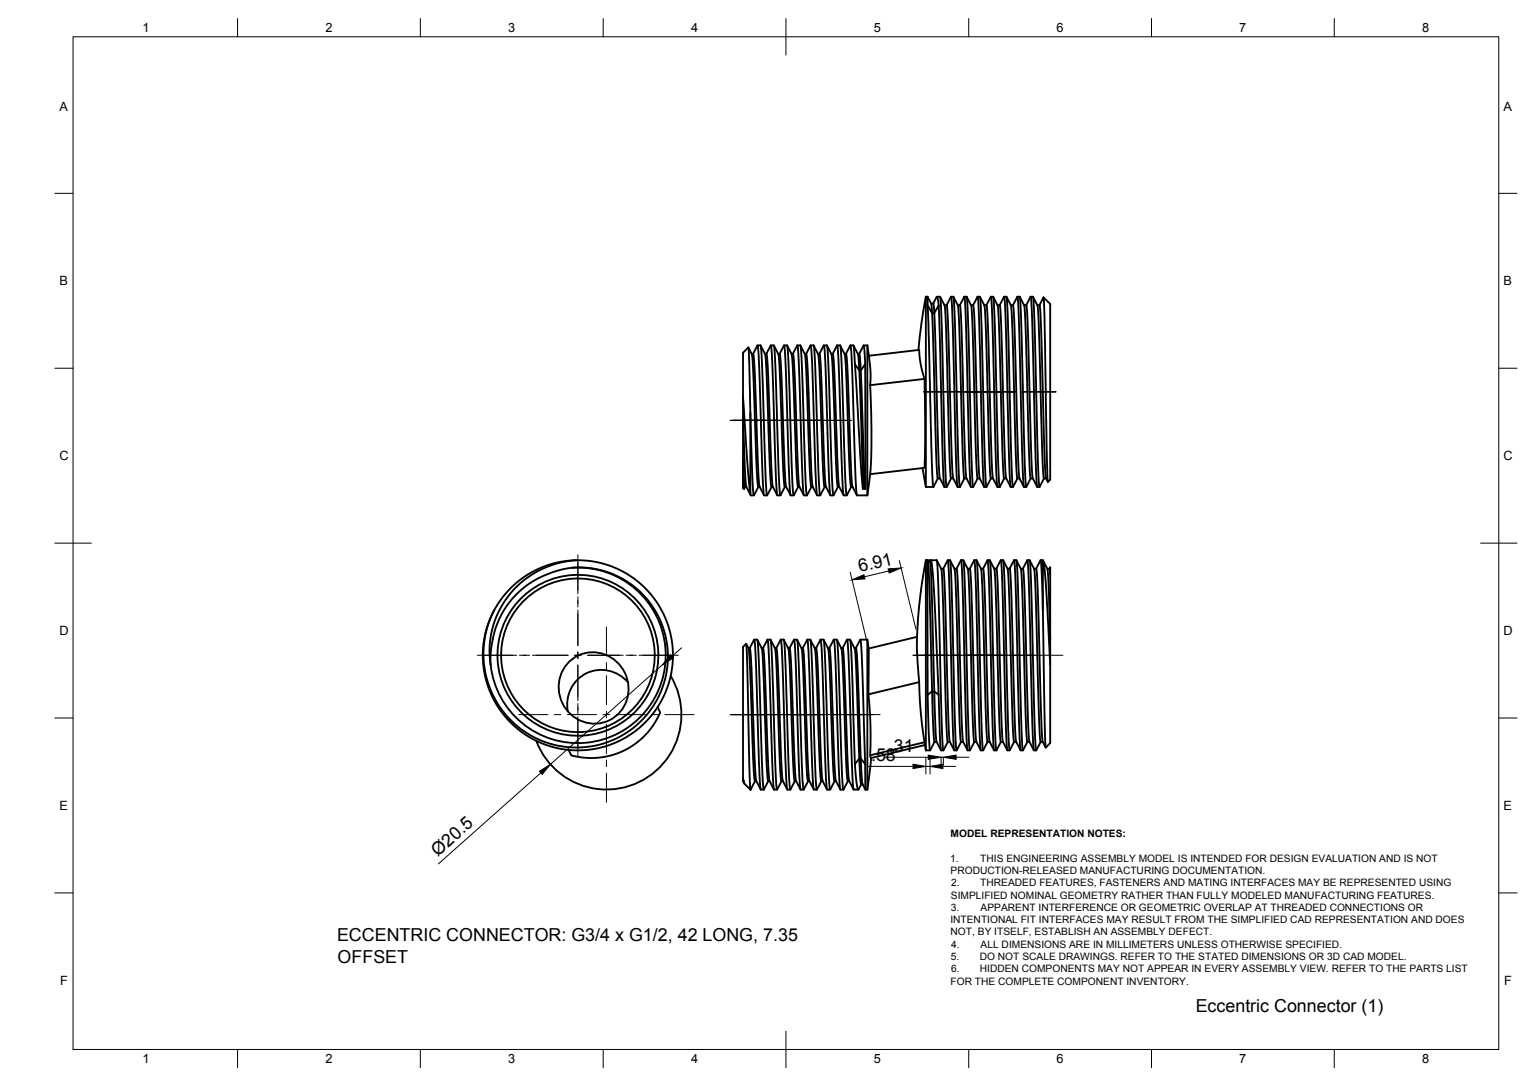
ISO-10303-21;
HEADER;
/* Generated by software containing ST-Developer
 * from STEP Tools, Inc. (www.steptools.com) 
 */

FILE_DESCRIPTION(
/* description */ ('STEP AP214'),
/* implementation_level */ '2;1');

FILE_NAME(
/* name */ 'Eccentric Connector (1).step',
/* time_stamp */ '2026-10-05T23:18:41-07:00',
/* author */ (''),
/* organization */ (''),
/* preprocessor_version */ 'ST-DEVELOPER v20.2',
/* originating_system */ 'Autodesk Translation Framework v15.15.0.0',
/* authorisation */ '');

FILE_SCHEMA (('AUTOMOTIVE_DESIGN { 1 0 10303 214 3 1 1 }'));
ENDSEC;

DATA;
#10=MECHANICAL_DESIGN_GEOMETRIC_PRESENTATION_REPRESENTATION('',(#111),#221662);
#72=MANIFOLD_SOLID_BREP('Body1',#79334);
#85=SHAPE_REPRESENTATION_RELATIONSHIP('SRR','None',#221720,#98);
#98=ADVANCED_BREP_SHAPE_REPRESENTATION('',(#72),#221660);
#111=STYLED_ITEM('',(#221783),#72);
#207=B_SPLINE_SURFACE_WITH_KNOTS('',3,3,((#208963,#208964,#208965,#208966,
#208967,#208968,#208969),(#208970,#208971,#208972,#208973,#208974,#208975,
#208976),(#208977,#208978,#208979,#208980,#208981,#208982,#208983),(#208984,
#208985,#208986,#208987,#208988,#208989,#208990)),.UNSPECIFIED.,.F.,.F.,
 .F.,(4,4),(4,1,1,1,4),(0.,1.),(0.,0.25,0.5,0.75,1.),.UNSPECIFIED.);
#208=B_SPLINE_SURFACE_WITH_KNOTS('',3,3,((#209027,#209028,#209029,#209030,
#209031,#209032,#209033,#209034,#209035,#209036,#209037,#209038,#209039,
#209040,#209041,#209042,#209043,#209044,#209045,#209046,#209047,#209048,
#209049,#209050,#209051,#209052,#209053,#209054,#209055,#209056,#209057,
#209058,#209059,#209060,#209061,#209062,#209063,#209064,#209065,#209066,
#209067,#209068,#209069,#209070,#209071,#209072,#209073,#209074,#209075,
#209076,#209077,#209078,#209079,#209080,#209081,#209082,#209083,#209084,
#209085,#209086,#209087,#209088,#209089,#209090,#209091,#209092,#209093),
(#209094,#209095,#209096,#209097,#209098,#209099,#209100,#209101,#209102,
#209103,#209104,#209105,#209106,#209107,#209108,#209109,#209110,#209111,
#209112,#209113,#209114,#209115,#209116,#209117,#209118,#209119,#209120,
#209121,#209122,#209123,#209124,#209125,#209126,#209127,#209128,#209129,
#209130,#209131,#209132,#209133,#209134,#209135,#209136,#209137,#209138,
#209139,#209140,#209141,#209142,#209143,#209144,#209145,#209146,#209147,
#209148,#209149,#209150,#209151,#209152,#209153,#209154,#209155,#209156,
#209157,#209158,#209159,#209160),(#209161,#209162,#209163,#209164,#209165,
#209166,#209167,#209168,#209169,#209170,#209171,#209172,#209173,#209174,
#209175,#209176,#209177,#209178,#209179,#209180,#209181,#209182,#209183,
#209184,#209185,#209186,#209187,#209188,#209189,#209190,#209191,#209192,
#209193,#209194,#209195,#209196,#209197,#209198,#209199,#209200,#209201,
#209202,#209203,#209204,#209205,#209206,#209207,#209208,#209209,#209210,
#209211,#209212,#209213,#209214,#209215,#209216,#209217,#209218,#209219,
#209220,#209221,#209222,#209223,#209224,#209225,#209226,#209227),(#209228,
#209229,#209230,#209231,#209232,#209233,#209234,#209235,#209236,#209237,
#209238,#209239,#209240,#209241,#209242,#209243,#209244,#209245,#209246,
#209247,#209248,#209249,#209250,#209251,#209252,#209253,#209254,#209255,
#209256,#209257,#209258,#209259,#209260,#209261,#209262,#209263,#209264,
#209265,#209266,#209267,#209268,#209269,#209270,#209271,#209272,#209273,
#209274,#209275,#209276,#209277,#209278,#209279,#209280,#209281,#209282,
#209283,#209284,#209285,#209286,#209287,#209288,#209289,#209290,#209291,
#209292,#209293,#209294)),.UNSPECIFIED.,.F.,.F.,.F.,(4,4),(4,1,1,1,1,1,
1,1,1,1,1,1,1,1,1,1,1,1,1,1,1,1,1,1,1,1,1,1,1,1,1,1,1,1,1,1,1,1,1,1,1,1,
1,1,1,1,1,1,1,1,1,1,1,1,1,1,1,1,1,1,1,1,1,1,4),(0.,1.),(0.,0.0156250000000022,
0.0312500000000006,0.0468750000000009,0.0625000000000012,0.0781250000000015,
0.0937500000000018,0.109375000000002,0.124999999999983,0.140624999999983,
0.156249999999984,0.171874999999984,0.187499999999984,0.203124999999984,
0.218749999999985,0.234374999999986,0.249999999999986,0.265624999999986,
0.281249999999986,0.296874999999986,0.312499999999987,0.328124999999987,
0.343749999999987,0.359374999999987,0.374999999999988,0.390624999999988,
0.406249999999988,0.421874999999989,0.437499999999989,0.45312499999999,
0.46874999999999,0.48437499999999,0.49999999999999,0.515624999999991,0.531249999999991,
0.546874999999991,0.562499999999992,0.578124999999992,0.593749999999992,
0.609374999999993,0.624999999999993,0.640624999999993,0.65625,0.671875,
0.6875,0.703125,0.71875,0.734375,0.75,0.765625,0.78125,0.796875,0.8125,
0.828125,0.84375,0.859375,0.875,0.890625,0.90625,0.921875,0.9375,0.953125,
0.96875,0.984375,1.),.UNSPECIFIED.);
#209=B_SPLINE_SURFACE_WITH_KNOTS('',3,3,((#209336,#209337,#209338,#209339,
#209340,#209341,#209342,#209343,#209344,#209345,#209346,#209347,#209348,
#209349,#209350,#209351,#209352,#209353,#209354,#209355,#209356,#209357,
#209358,#209359,#209360,#209361,#209362,#209363,#209364,#209365,#209366,
#209367,#209368,#209369,#209370,#209371,#209372,#209373,#209374,#209375,
#209376,#209377,#209378,#209379,#209380,#209381,#209382,#209383,#209384,
#209385,#209386,#209387,#209388,#209389,#209390,#209391,#209392,#209393,
#209394,#209395,#209396,#209397,#209398,#209399,#209400,#209401,#209402),
(#209403,#209404,#209405,#209406,#209407,#209408,#209409,#209410,#209411,
#209412,#209413,#209414,#209415,#209416,#209417,#209418,#209419,#209420,
#209421,#209422,#209423,#209424,#209425,#209426,#209427,#209428,#209429,
#209430,#209431,#209432,#209433,#209434,#209435,#209436,#209437,#209438,
#209439,#209440,#209441,#209442,#209443,#209444,#209445,#209446,#209447,
#209448,#209449,#209450,#209451,#209452,#209453,#209454,#209455,#209456,
#209457,#209458,#209459,#209460,#209461,#209462,#209463,#209464,#209465,
#209466,#209467,#209468,#209469),(#209470,#209471,#209472,#209473,#209474,
#209475,#209476,#209477,#209478,#209479,#209480,#209481,#209482,#209483,
#209484,#209485,#209486,#209487,#209488,#209489,#209490,#209491,#209492,
#209493,#209494,#209495,#209496,#209497,#209498,#209499,#209500,#209501,
#209502,#209503,#209504,#209505,#209506,#209507,#209508,#209509,#209510,
#209511,#209512,#209513,#209514,#209515,#209516,#209517,#209518,#209519,
#209520,#209521,#209522,#209523,#209524,#209525,#209526,#209527,#209528,
#209529,#209530,#209531,#209532,#209533,#209534,#209535,#209536),(#209537,
#209538,#209539,#209540,#209541,#209542,#209543,#209544,#209545,#209546,
#209547,#209548,#209549,#209550,#209551,#209552,#209553,#209554,#209555,
#209556,#209557,#209558,#209559,#209560,#209561,#209562,#209563,#209564,
#209565,#209566,#209567,#209568,#209569,#209570,#209571,#209572,#209573,
#209574,#209575,#209576,#209577,#209578,#209579,#209580,#209581,#209582,
#209583,#209584,#209585,#209586,#209587,#209588,#209589,#209590,#209591,
#209592,#209593,#209594,#209595,#209596,#209597,#209598,#209599,#209600,
#209601,#209602,#209603)),.UNSPECIFIED.,.F.,.F.,.F.,(4,4),(4,1,1,1,1,1,
1,1,1,1,1,1,1,1,1,1,1,1,1,1,1,1,1,1,1,1,1,1,1,1,1,1,1,1,1,1,1,1,1,1,1,1,
1,1,1,1,1,1,1,1,1,1,1,1,1,1,1,1,1,1,1,1,1,1,4),(0.,1.),(0.,0.0156250000000031,
0.03125,0.046875,0.0625,0.078125,0.09375,0.109375,0.124999999999992,0.140624999999992,
0.156249999999992,0.171874999999992,0.187499999999992,0.203124999999992,
0.218749999999993,0.234374999999993,0.249999999999993,0.265624999999993,
0.281249999999993,0.296874999999993,0.312499999999993,0.328124999999993,
0.343749999999994,0.359374999999994,0.374999999999994,0.390624999999994,
0.406249999999994,0.421874999999994,0.437499999999994,0.453125,0.46875,
0.484375,0.5,0.515625,0.53125,0.546875,0.5625,0.578125,0.59375,0.609375,
0.625,0.640625,0.65625,0.671875,0.6875,0.703125,0.71875,0.734375,0.75,0.765625,
0.78125,0.796875,0.8125,0.828125,0.84375,0.859375,0.875,0.890625,0.90625,
0.921875,0.9375,0.953125,0.96875,0.984375,1.),.UNSPECIFIED.);
#210=B_SPLINE_SURFACE_WITH_KNOTS('',3,3,((#209610,#209611,#209612,#209613,
#209614,#209615,#209616),(#209617,#209618,#209619,#209620,#209621,#209622,
#209623),(#209624,#209625,#209626,#209627,#209628,#209629,#209630),(#209631,
#209632,#209633,#209634,#209635,#209636,#209637)),.UNSPECIFIED.,.F.,.F.,
 .F.,(4,4),(4,1,1,1,4),(0.,1.),(0.,0.250000000000029,0.500000000000019,
0.75000000000001,1.),.UNSPECIFIED.);
#211=B_SPLINE_SURFACE_WITH_KNOTS('',3,3,((#209651,#209652,#209653,#209654,
#209655,#209656,#209657),(#209658,#209659,#209660,#209661,#209662,#209663,
#209664),(#209665,#209666,#209667,#209668,#209669,#209670,#209671),(#209672,
#209673,#209674,#209675,#209676,#209677,#209678)),.UNSPECIFIED.,.F.,.F.,
 .F.,(4,4),(4,1,1,1,4),(0.,1.),(0.,0.25,0.5,0.75,1.),.UNSPECIFIED.);
#212=B_SPLINE_SURFACE_WITH_KNOTS('',3,3,((#209685,#209686,#209687,#209688,
#209689,#209690,#209691,#209692,#209693,#209694,#209695,#209696,#209697,
#209698,#209699,#209700,#209701,#209702,#209703,#209704,#209705,#209706,
#209707,#209708,#209709,#209710,#209711,#209712,#209713,#209714,#209715,
#209716,#209717,#209718,#209719,#209720,#209721,#209722,#209723,#209724,
#209725,#209726,#209727,#209728,#209729,#209730,#209731,#209732,#209733,
#209734,#209735,#209736,#209737,#209738,#209739,#209740,#209741,#209742,
#209743,#209744,#209745,#209746,#209747,#209748,#209749,#209750,#209751),
(#209752,#209753,#209754,#209755,#209756,#209757,#209758,#209759,#209760,
#209761,#209762,#209763,#209764,#209765,#209766,#209767,#209768,#209769,
#209770,#209771,#209772,#209773,#209774,#209775,#209776,#209777,#209778,
#209779,#209780,#209781,#209782,#209783,#209784,#209785,#209786,#209787,
#209788,#209789,#209790,#209791,#209792,#209793,#209794,#209795,#209796,
#209797,#209798,#209799,#209800,#209801,#209802,#209803,#209804,#209805,
#209806,#209807,#209808,#209809,#209810,#209811,#209812,#209813,#209814,
#209815,#209816,#209817,#209818),(#209819,#209820,#209821,#209822,#209823,
#209824,#209825,#209826,#209827,#209828,#209829,#209830,#209831,#209832,
#209833,#209834,#209835,#209836,#209837,#209838,#209839,#209840,#209841,
#209842,#209843,#209844,#209845,#209846,#209847,#209848,#209849,#209850,
#209851,#209852,#209853,#209854,#209855,#209856,#209857,#209858,#209859,
#209860,#209861,#209862,#209863,#209864,#209865,#209866,#209867,#209868,
#209869,#209870,#209871,#209872,#209873,#209874,#209875,#209876,#209877,
#209878,#209879,#209880,#209881,#209882,#209883,#209884,#209885),(#209886,
#209887,#209888,#209889,#209890,#209891,#209892,#209893,#209894,#209895,
#209896,#209897,#209898,#209899,#209900,#209901,#209902,#209903,#209904,
#209905,#209906,#209907,#209908,#209909,#209910,#209911,#209912,#209913,
#209914,#209915,#209916,#209917,#209918,#209919,#209920,#209921,#209922,
#209923,#209924,#209925,#209926,#209927,#209928,#209929,#209930,#209931,
#209932,#209933,#209934,#209935,#209936,#209937,#209938,#209939,#209940,
#209941,#209942,#209943,#209944,#209945,#209946,#209947,#209948,#209949,
#209950,#209951,#209952)),.UNSPECIFIED.,.F.,.F.,.F.,(4,4),(4,1,1,1,1,1,
1,1,1,1,1,1,1,1,1,1,1,1,1,1,1,1,1,1,1,1,1,1,1,1,1,1,1,1,1,1,1,1,1,1,1,1,
1,1,1,1,1,1,1,1,1,1,1,1,1,1,1,1,1,1,1,1,1,1,4),(0.,1.),(0.,0.0156250000000031,
0.03125,0.046875,0.0625,0.078125,0.09375,0.109375,0.124999999999992,0.140624999999992,
0.156249999999992,0.171874999999992,0.187499999999992,0.203124999999992,
0.218749999999993,0.234374999999993,0.249999999999993,0.265624999999993,
0.281249999999993,0.296874999999993,0.312499999999993,0.328124999999993,
0.343749999999994,0.359374999999994,0.374999999999994,0.390624999999994,
0.406249999999994,0.421874999999994,0.437499999999994,0.453125,0.46875,
0.484375,0.5,0.515625,0.53125,0.546875,0.5625,0.578125,0.59375,0.609375,
0.625,0.640625,0.65625,0.671875,0.6875,0.703125,0.71875,0.734375,0.75,0.765625,
0.78125,0.796875,0.8125,0.828125,0.84375,0.859375,0.875,0.890625,0.90625,
0.921875,0.9375,0.953125,0.96875,0.984375,1.),.UNSPECIFIED.);
#213=B_SPLINE_SURFACE_WITH_KNOTS('',3,3,((#209954,#209955,#209956,#209957,
#209958,#209959,#209960,#209961,#209962,#209963,#209964,#209965,#209966,
#209967,#209968,#209969,#209970,#209971,#209972,#209973,#209974,#209975,
#209976,#209977,#209978,#209979,#209980,#209981,#209982,#209983,#209984,
#209985,#209986,#209987,#209988,#209989,#209990,#209991,#209992,#209993,
#209994,#209995,#209996,#209997,#209998,#209999,#210000,#210001,#210002,
#210003,#210004,#210005,#210006,#210007,#210008,#210009,#210010,#210011,
#210012,#210013,#210014,#210015,#210016,#210017,#210018,#210019,#210020),
(#210021,#210022,#210023,#210024,#210025,#210026,#210027,#210028,#210029,
#210030,#210031,#210032,#210033,#210034,#210035,#210036,#210037,#210038,
#210039,#210040,#210041,#210042,#210043,#210044,#210045,#210046,#210047,
#210048,#210049,#210050,#210051,#210052,#210053,#210054,#210055,#210056,
#210057,#210058,#210059,#210060,#210061,#210062,#210063,#210064,#210065,
#210066,#210067,#210068,#210069,#210070,#210071,#210072,#210073,#210074,
#210075,#210076,#210077,#210078,#210079,#210080,#210081,#210082,#210083,
#210084,#210085,#210086,#210087),(#210088,#210089,#210090,#210091,#210092,
#210093,#210094,#210095,#210096,#210097,#210098,#210099,#210100,#210101,
#210102,#210103,#210104,#210105,#210106,#210107,#210108,#210109,#210110,
#210111,#210112,#210113,#210114,#210115,#210116,#210117,#210118,#210119,
#210120,#210121,#210122,#210123,#210124,#210125,#210126,#210127,#210128,
#210129,#210130,#210131,#210132,#210133,#210134,#210135,#210136,#210137,
#210138,#210139,#210140,#210141,#210142,#210143,#210144,#210145,#210146,
#210147,#210148,#210149,#210150,#210151,#210152,#210153,#210154),(#210155,
#210156,#210157,#210158,#210159,#210160,#210161,#210162,#210163,#210164,
#210165,#210166,#210167,#210168,#210169,#210170,#210171,#210172,#210173,
#210174,#210175,#210176,#210177,#210178,#210179,#210180,#210181,#210182,
#210183,#210184,#210185,#210186,#210187,#210188,#210189,#210190,#210191,
#210192,#210193,#210194,#210195,#210196,#210197,#210198,#210199,#210200,
#210201,#210202,#210203,#210204,#210205,#210206,#210207,#210208,#210209,
#210210,#210211,#210212,#210213,#210214,#210215,#210216,#210217,#210218,
#210219,#210220,#210221)),.UNSPECIFIED.,.F.,.F.,.F.,(4,4),(4,1,1,1,1,1,
1,1,1,1,1,1,1,1,1,1,1,1,1,1,1,1,1,1,1,1,1,1,1,1,1,1,1,1,1,1,1,1,1,1,1,1,
1,1,1,1,1,1,1,1,1,1,1,1,1,1,1,1,1,1,1,1,1,1,4),(0.,1.),(0.,0.0156250000000022,
0.0312500000000006,0.0468750000000009,0.0625000000000012,0.0781250000000015,
0.0937500000000018,0.109375000000002,0.124999999999983,0.140624999999983,
0.156249999999984,0.171874999999984,0.187499999999984,0.203124999999984,
0.218749999999985,0.234374999999986,0.249999999999986,0.265624999999986,
0.281249999999986,0.296874999999986,0.312499999999987,0.328124999999987,
0.343749999999987,0.359374999999987,0.374999999999988,0.390624999999988,
0.406249999999988,0.421874999999989,0.437499999999989,0.45312499999999,
0.46874999999999,0.48437499999999,0.49999999999999,0.515624999999991,0.531249999999991,
0.546874999999991,0.562499999999992,0.578124999999992,0.593749999999992,
0.609374999999993,0.624999999999993,0.640624999999993,0.65625,0.671875,
0.6875,0.703125,0.71875,0.734375,0.75,0.765625,0.78125,0.796875,0.8125,
0.828125,0.84375,0.859375,0.875,0.890625,0.90625,0.921875,0.9375,0.953125,
0.96875,0.984375,1.),.UNSPECIFIED.);
#214=B_SPLINE_SURFACE_WITH_KNOTS('',3,3,((#210223,#210224,#210225,#210226,
#210227,#210228,#210229,#210230,#210231,#210232,#210233,#210234,#210235,
#210236,#210237,#210238,#210239,#210240,#210241),(#210242,#210243,#210244,
#210245,#210246,#210247,#210248,#210249,#210250,#210251,#210252,#210253,
#210254,#210255,#210256,#210257,#210258,#210259,#210260),(#210261,#210262,
#210263,#210264,#210265,#210266,#210267,#210268,#210269,#210270,#210271,
#210272,#210273,#210274,#210275,#210276,#210277,#210278,#210279),(#210280,
#210281,#210282,#210283,#210284,#210285,#210286,#210287,#210288,#210289,
#210290,#210291,#210292,#210293,#210294,#210295,#210296,#210297,#210298)),
 .UNSPECIFIED.,.F.,.F.,.F.,(4,4),(4,1,1,1,1,1,1,1,1,1,1,1,1,1,1,1,4),(0.,
1.),(0.,0.0624999999999738,0.124999999999948,0.187499999999503,0.249999999999477,
0.312499999999451,0.374999999999424,0.437499999999398,0.499999999999372,
0.562499999999346,0.62499999999932,0.687499999998875,0.749999999998849,
0.812499999998822,0.874999999998796,0.93749999999877,1.),.UNSPECIFIED.);
#215=B_SPLINE_SURFACE_WITH_KNOTS('',3,3,((#210340,#210341,#210342,#210343,
#210344,#210345,#210346),(#210347,#210348,#210349,#210350,#210351,#210352,
#210353),(#210354,#210355,#210356,#210357,#210358,#210359,#210360),(#210361,
#210362,#210363,#210364,#210365,#210366,#210367)),.UNSPECIFIED.,.F.,.F.,
 .F.,(4,4),(4,1,1,1,4),(0.,1.),(0.,0.25,0.5,0.75,1.),.UNSPECIFIED.);
#216=B_SPLINE_SURFACE_WITH_KNOTS('',3,3,((#210404,#210405,#210406,#210407,
#210408,#210409,#210410,#210411,#210412,#210413,#210414,#210415,#210416,
#210417,#210418,#210419,#210420,#210421,#210422,#210423,#210424,#210425,
#210426,#210427,#210428,#210429,#210430,#210431,#210432,#210433,#210434,
#210435,#210436,#210437,#210438),(#210439,#210440,#210441,#210442,#210443,
#210444,#210445,#210446,#210447,#210448,#210449,#210450,#210451,#210452,
#210453,#210454,#210455,#210456,#210457,#210458,#210459,#210460,#210461,
#210462,#210463,#210464,#210465,#210466,#210467,#210468,#210469,#210470,
#210471,#210472,#210473),(#210474,#210475,#210476,#210477,#210478,#210479,
#210480,#210481,#210482,#210483,#210484,#210485,#210486,#210487,#210488,
#210489,#210490,#210491,#210492,#210493,#210494,#210495,#210496,#210497,
#210498,#210499,#210500,#210501,#210502,#210503,#210504,#210505,#210506,
#210507,#210508),(#210509,#210510,#210511,#210512,#210513,#210514,#210515,
#210516,#210517,#210518,#210519,#210520,#210521,#210522,#210523,#210524,
#210525,#210526,#210527,#210528,#210529,#210530,#210531,#210532,#210533,
#210534,#210535,#210536,#210537,#210538,#210539,#210540,#210541,#210542,
#210543)),.UNSPECIFIED.,.F.,.F.,.F.,(4,4),(4,1,1,1,1,1,1,1,1,1,1,1,1,1,
1,1,1,1,1,1,1,1,1,1,1,1,1,1,1,1,1,1,4),(0.,1.),(0.,0.0312500000000088,0.0625000000000175,
0.0937500000000263,0.125000000000035,0.156250000000044,0.187500000000053,
0.218750000000062,0.25000000000007,0.281250000000078,0.312500000000087,
0.343750000000096,0.375000000000105,0.406250000000114,0.437500000000123,
0.468750000000131,0.50000000000014,0.531250000000149,0.562500000000157,
0.593750000000166,0.625000000000175,0.656250000000184,0.687500000000192,
0.718750000000201,0.75000000000021,0.781250000000079,0.812500000000087,
0.843750000000096,0.875000000000105,0.906250000000114,0.937500000000122,
0.968750000000131,1.),.UNSPECIFIED.);
#217=B_SPLINE_SURFACE_WITH_KNOTS('',3,3,((#211020,#211021,#211022,#211023,
#211024,#211025,#211026,#211027,#211028,#211029,#211030,#211031,#211032,
#211033,#211034,#211035,#211036,#211037,#211038,#211039,#211040,#211041,
#211042,#211043,#211044,#211045,#211046,#211047,#211048,#211049,#211050,
#211051,#211052,#211053,#211054,#211055,#211056,#211057,#211058,#211059,
#211060,#211061,#211062,#211063,#211064,#211065,#211066,#211067,#211068,
#211069,#211070,#211071,#211072,#211073,#211074,#211075,#211076,#211077,
#211078,#211079,#211080,#211081,#211082,#211083,#211084,#211085,#211086),
(#211087,#211088,#211089,#211090,#211091,#211092,#211093,#211094,#211095,
#211096,#211097,#211098,#211099,#211100,#211101,#211102,#211103,#211104,
#211105,#211106,#211107,#211108,#211109,#211110,#211111,#211112,#211113,
#211114,#211115,#211116,#211117,#211118,#211119,#211120,#211121,#211122,
#211123,#211124,#211125,#211126,#211127,#211128,#211129,#211130,#211131,
#211132,#211133,#211134,#211135,#211136,#211137,#211138,#211139,#211140,
#211141,#211142,#211143,#211144,#211145,#211146,#211147,#211148,#211149,
#211150,#211151,#211152,#211153),(#211154,#211155,#211156,#211157,#211158,
#211159,#211160,#211161,#211162,#211163,#211164,#211165,#211166,#211167,
#211168,#211169,#211170,#211171,#211172,#211173,#211174,#211175,#211176,
#211177,#211178,#211179,#211180,#211181,#211182,#211183,#211184,#211185,
#211186,#211187,#211188,#211189,#211190,#211191,#211192,#211193,#211194,
#211195,#211196,#211197,#211198,#211199,#211200,#211201,#211202,#211203,
#211204,#211205,#211206,#211207,#211208,#211209,#211210,#211211,#211212,
#211213,#211214,#211215,#211216,#211217,#211218,#211219,#211220),(#211221,
#211222,#211223,#211224,#211225,#211226,#211227,#211228,#211229,#211230,
#211231,#211232,#211233,#211234,#211235,#211236,#211237,#211238,#211239,
#211240,#211241,#211242,#211243,#211244,#211245,#211246,#211247,#211248,
#211249,#211250,#211251,#211252,#211253,#211254,#211255,#211256,#211257,
#211258,#211259,#211260,#211261,#211262,#211263,#211264,#211265,#211266,
#211267,#211268,#211269,#211270,#211271,#211272,#211273,#211274,#211275,
#211276,#211277,#211278,#211279,#211280,#211281,#211282,#211283,#211284,
#211285,#211286,#211287)),.UNSPECIFIED.,.F.,.F.,.F.,(4,4),(4,1,1,1,1,1,
1,1,1,1,1,1,1,1,1,1,1,1,1,1,1,1,1,1,1,1,1,1,1,1,1,1,1,1,1,1,1,1,1,1,1,1,
1,1,1,1,1,1,1,1,1,1,1,1,1,1,1,1,1,1,1,1,1,1,4),(0.,1.),(0.,0.015625,0.03125,
0.046875,0.0625,0.078125,0.09375,0.109375,0.125,0.140625,0.15625,0.171875,
0.1875,0.203125,0.21875,0.234375,0.25,0.265625,0.28125,0.296875,0.3125,
0.328125,0.34375,0.359375,0.375,0.390625,0.40625,0.421875,0.4375,0.453125,
0.46875,0.484375,0.5,0.515625,0.53125,0.546875,0.5625,0.578125,0.59375,
0.609375,0.625,0.640625,0.65625,0.671875,0.6875,0.703125,0.71875,0.734375,
0.75,0.765625,0.78125,0.796875,0.8125,0.828125,0.84375,0.859375,0.875,0.890625,
0.90625,0.921875,0.9375,0.953125,0.96875,0.984375,1.),.UNSPECIFIED.);
#218=B_SPLINE_SURFACE_WITH_KNOTS('',3,3,((#211354,#211355,#211356,#211357,
#211358,#211359,#211360),(#211361,#211362,#211363,#211364,#211365,#211366,
#211367),(#211368,#211369,#211370,#211371,#211372,#211373,#211374),(#211375,
#211376,#211377,#211378,#211379,#211380,#211381)),.UNSPECIFIED.,.F.,.F.,
 .F.,(4,4),(4,1,1,1,4),(0.,1.),(0.,0.250000000000007,0.5,0.75,1.),
 .UNSPECIFIED.);
#219=B_SPLINE_SURFACE_WITH_KNOTS('',3,3,((#211409,#211410,#211411,#211412,
#211413,#211414,#211415),(#211416,#211417,#211418,#211419,#211420,#211421,
#211422),(#211423,#211424,#211425,#211426,#211427,#211428,#211429),(#211430,
#211431,#211432,#211433,#211434,#211435,#211436)),.UNSPECIFIED.,.F.,.F.,
 .F.,(4,4),(4,1,1,1,4),(0.,1.),(0.,0.25,0.5,0.75,1.),.UNSPECIFIED.);
#220=B_SPLINE_SURFACE_WITH_KNOTS('',3,3,((#211443,#211444,#211445,#211446,
#211447,#211448,#211449,#211450,#211451,#211452,#211453,#211454,#211455,
#211456,#211457,#211458,#211459,#211460,#211461,#211462,#211463,#211464,
#211465,#211466,#211467,#211468,#211469,#211470,#211471,#211472,#211473,
#211474,#211475,#211476,#211477,#211478,#211479,#211480,#211481,#211482,
#211483,#211484,#211485,#211486,#211487,#211488,#211489,#211490,#211491,
#211492,#211493,#211494,#211495,#211496,#211497,#211498,#211499,#211500,
#211501,#211502,#211503,#211504,#211505,#211506,#211507,#211508,#211509),
(#211510,#211511,#211512,#211513,#211514,#211515,#211516,#211517,#211518,
#211519,#211520,#211521,#211522,#211523,#211524,#211525,#211526,#211527,
#211528,#211529,#211530,#211531,#211532,#211533,#211534,#211535,#211536,
#211537,#211538,#211539,#211540,#211541,#211542,#211543,#211544,#211545,
#211546,#211547,#211548,#211549,#211550,#211551,#211552,#211553,#211554,
#211555,#211556,#211557,#211558,#211559,#211560,#211561,#211562,#211563,
#211564,#211565,#211566,#211567,#211568,#211569,#211570,#211571,#211572,
#211573,#211574,#211575,#211576),(#211577,#211578,#211579,#211580,#211581,
#211582,#211583,#211584,#211585,#211586,#211587,#211588,#211589,#211590,
#211591,#211592,#211593,#211594,#211595,#211596,#211597,#211598,#211599,
#211600,#211601,#211602,#211603,#211604,#211605,#211606,#211607,#211608,
#211609,#211610,#211611,#211612,#211613,#211614,#211615,#211616,#211617,
#211618,#211619,#211620,#211621,#211622,#211623,#211624,#211625,#211626,
#211627,#211628,#211629,#211630,#211631,#211632,#211633,#211634,#211635,
#211636,#211637,#211638,#211639,#211640,#211641,#211642,#211643),(#211644,
#211645,#211646,#211647,#211648,#211649,#211650,#211651,#211652,#211653,
#211654,#211655,#211656,#211657,#211658,#211659,#211660,#211661,#211662,
#211663,#211664,#211665,#211666,#211667,#211668,#211669,#211670,#211671,
#211672,#211673,#211674,#211675,#211676,#211677,#211678,#211679,#211680,
#211681,#211682,#211683,#211684,#211685,#211686,#211687,#211688,#211689,
#211690,#211691,#211692,#211693,#211694,#211695,#211696,#211697,#211698,
#211699,#211700,#211701,#211702,#211703,#211704,#211705,#211706,#211707,
#211708,#211709,#211710)),.UNSPECIFIED.,.F.,.F.,.F.,(4,4),(4,1,1,1,1,1,
1,1,1,1,1,1,1,1,1,1,1,1,1,1,1,1,1,1,1,1,1,1,1,1,1,1,1,1,1,1,1,1,1,1,1,1,
1,1,1,1,1,1,1,1,1,1,1,1,1,1,1,1,1,1,1,1,1,1,4),(0.,1.),(0.,0.015625,0.03125,
0.046875,0.0625,0.078125,0.09375,0.109375,0.125,0.140625,0.15625,0.171875,
0.1875,0.203125,0.21875,0.234375,0.25,0.265625,0.28125,0.296875,0.3125,
0.328125,0.34375,0.359375,0.375,0.390625,0.40625,0.421875,0.4375,0.453125,
0.46875,0.484375,0.5,0.515625,0.53125,0.546875,0.5625,0.578125,0.59375,
0.609375,0.625,0.640625,0.65625,0.671875,0.6875,0.703125,0.71875,0.734375,
0.75,0.765625,0.78125,0.796875,0.8125,0.828125,0.84375,0.859375,0.875,0.890625,
0.90625,0.921875,0.9375,0.953125,0.96875,0.984375,1.),.UNSPECIFIED.);
#221=B_SPLINE_SURFACE_WITH_KNOTS('',3,3,((#211790,#211791,#211792,#211793,
#211794,#211795,#211796,#211797,#211798,#211799,#211800,#211801,#211802,
#211803,#211804,#211805,#211806,#211807,#211808,#211809,#211810,#211811,
#211812,#211813,#211814,#211815,#211816,#211817,#211818,#211819,#211820,
#211821,#211822,#211823,#211824,#211825,#211826,#211827,#211828,#211829,
#211830,#211831,#211832,#211833,#211834,#211835,#211836,#211837,#211838,
#211839,#211840,#211841,#211842,#211843,#211844,#211845,#211846,#211847,
#211848,#211849,#211850,#211851,#211852,#211853,#211854,#211855,#211856),
(#211857,#211858,#211859,#211860,#211861,#211862,#211863,#211864,#211865,
#211866,#211867,#211868,#211869,#211870,#211871,#211872,#211873,#211874,
#211875,#211876,#211877,#211878,#211879,#211880,#211881,#211882,#211883,
#211884,#211885,#211886,#211887,#211888,#211889,#211890,#211891,#211892,
#211893,#211894,#211895,#211896,#211897,#211898,#211899,#211900,#211901,
#211902,#211903,#211904,#211905,#211906,#211907,#211908,#211909,#211910,
#211911,#211912,#211913,#211914,#211915,#211916,#211917,#211918,#211919,
#211920,#211921,#211922,#211923),(#211924,#211925,#211926,#211927,#211928,
#211929,#211930,#211931,#211932,#211933,#211934,#211935,#211936,#211937,
#211938,#211939,#211940,#211941,#211942,#211943,#211944,#211945,#211946,
#211947,#211948,#211949,#211950,#211951,#211952,#211953,#211954,#211955,
#211956,#211957,#211958,#211959,#211960,#211961,#211962,#211963,#211964,
#211965,#211966,#211967,#211968,#211969,#211970,#211971,#211972,#211973,
#211974,#211975,#211976,#211977,#211978,#211979,#211980,#211981,#211982,
#211983,#211984,#211985,#211986,#211987,#211988,#211989,#211990),(#211991,
#211992,#211993,#211994,#211995,#211996,#211997,#211998,#211999,#212000,
#212001,#212002,#212003,#212004,#212005,#212006,#212007,#212008,#212009,
#212010,#212011,#212012,#212013,#212014,#212015,#212016,#212017,#212018,
#212019,#212020,#212021,#212022,#212023,#212024,#212025,#212026,#212027,
#212028,#212029,#212030,#212031,#212032,#212033,#212034,#212035,#212036,
#212037,#212038,#212039,#212040,#212041,#212042,#212043,#212044,#212045,
#212046,#212047,#212048,#212049,#212050,#212051,#212052,#212053,#212054,
#212055,#212056,#212057)),.UNSPECIFIED.,.F.,.F.,.F.,(4,4),(4,1,1,1,1,1,
1,1,1,1,1,1,1,1,1,1,1,1,1,1,1,1,1,1,1,1,1,1,1,1,1,1,1,1,1,1,1,1,1,1,1,1,
1,1,1,1,1,1,1,1,1,1,1,1,1,1,1,1,1,1,1,1,1,1,4),(0.,1.),(0.,0.015625,0.03125,
0.046875,0.0625,0.078125,0.09375,0.109375,0.125,0.140625,0.15625,0.171875,
0.1875,0.203125,0.21875,0.234375,0.25,0.265625,0.28125,0.296875,0.3125,
0.328125,0.34375,0.359375,0.375,0.390625,0.40625,0.421875,0.4375,0.453125,
0.46875,0.484375,0.5,0.515625,0.53125,0.546875,0.5625,0.578125,0.59375,
0.609375,0.625,0.640625,0.65625,0.671875,0.6875,0.703125,0.71875,0.734375,
0.75,0.765625,0.78125,0.796875,0.8125,0.828125,0.84375,0.859375,0.875,0.890625,
0.90625,0.921875,0.9375,0.953125,0.96875,0.984375,1.),.UNSPECIFIED.);
#222=B_SPLINE_SURFACE_WITH_KNOTS('',3,3,((#212059,#212060,#212061,#212062,
#212063,#212064,#212065,#212066,#212067,#212068,#212069,#212070,#212071,
#212072,#212073,#212074,#212075,#212076,#212077,#212078,#212079,#212080,
#212081,#212082,#212083,#212084,#212085,#212086,#212087,#212088,#212089,
#212090,#212091,#212092,#212093),(#212094,#212095,#212096,#212097,#212098,
#212099,#212100,#212101,#212102,#212103,#212104,#212105,#212106,#212107,
#212108,#212109,#212110,#212111,#212112,#212113,#212114,#212115,#212116,
#212117,#212118,#212119,#212120,#212121,#212122,#212123,#212124,#212125,
#212126,#212127,#212128),(#212129,#212130,#212131,#212132,#212133,#212134,
#212135,#212136,#212137,#212138,#212139,#212140,#212141,#212142,#212143,
#212144,#212145,#212146,#212147,#212148,#212149,#212150,#212151,#212152,
#212153,#212154,#212155,#212156,#212157,#212158,#212159,#212160,#212161,
#212162,#212163),(#212164,#212165,#212166,#212167,#212168,#212169,#212170,
#212171,#212172,#212173,#212174,#212175,#212176,#212177,#212178,#212179,
#212180,#212181,#212182,#212183,#212184,#212185,#212186,#212187,#212188,
#212189,#212190,#212191,#212192,#212193,#212194,#212195,#212196,#212197,
#212198)),.UNSPECIFIED.,.F.,.F.,.F.,(4,4),(4,1,1,1,1,1,1,1,1,1,1,1,1,1,
1,1,1,1,1,1,1,1,1,1,1,1,1,1,1,1,1,1,4),(0.,1.),(0.,0.0312499999999743,0.0624999999999486,
0.0937499999999229,0.125000000000034,0.156250000000008,0.187499999999983,
0.218749999999957,0.249999999999932,0.281250000000043,0.312500000000017,
0.343749999999991,0.374999999999966,0.406250000000077,0.437500000000052,
0.468750000000026,0.5,0.531249999999974,0.562500000000086,0.59375000000006,
0.625000000000034,0.656250000000009,0.687499999999983,0.718750000000095,
0.750000000000069,0.781250000000043,0.812500000000017,0.843750000000129,
0.875000000000103,0.906250000000077,0.937500000000052,0.968750000000026,
1.),.UNSPECIFIED.);
#223=B_SPLINE_SURFACE_WITH_KNOTS('',3,3,((#212211,#212212,#212213,#212214,
#212215,#212216,#212217,#212218,#212219,#212220,#212221,#212222,#212223,
#212224,#212225,#212226,#212227,#212228,#212229,#212230,#212231,#212232,
#212233,#212234,#212235,#212236,#212237,#212238,#212239,#212240,#212241,
#212242,#212243,#212244,#212245,#212246,#212247,#212248,#212249,#212250,
#212251,#212252,#212253,#212254,#212255,#212256,#212257,#212258,#212259,
#212260,#212261,#212262,#212263,#212264,#212265,#212266,#212267,#212268,
#212269,#212270,#212271,#212272,#212273,#212274,#212275,#212276,#212277),
(#212278,#212279,#212280,#212281,#212282,#212283,#212284,#212285,#212286,
#212287,#212288,#212289,#212290,#212291,#212292,#212293,#212294,#212295,
#212296,#212297,#212298,#212299,#212300,#212301,#212302,#212303,#212304,
#212305,#212306,#212307,#212308,#212309,#212310,#212311,#212312,#212313,
#212314,#212315,#212316,#212317,#212318,#212319,#212320,#212321,#212322,
#212323,#212324,#212325,#212326,#212327,#212328,#212329,#212330,#212331,
#212332,#212333,#212334,#212335,#212336,#212337,#212338,#212339,#212340,
#212341,#212342,#212343,#212344),(#212345,#212346,#212347,#212348,#212349,
#212350,#212351,#212352,#212353,#212354,#212355,#212356,#212357,#212358,
#212359,#212360,#212361,#212362,#212363,#212364,#212365,#212366,#212367,
#212368,#212369,#212370,#212371,#212372,#212373,#212374,#212375,#212376,
#212377,#212378,#212379,#212380,#212381,#212382,#212383,#212384,#212385,
#212386,#212387,#212388,#212389,#212390,#212391,#212392,#212393,#212394,
#212395,#212396,#212397,#212398,#212399,#212400,#212401,#212402,#212403,
#212404,#212405,#212406,#212407,#212408,#212409,#212410,#212411),(#212412,
#212413,#212414,#212415,#212416,#212417,#212418,#212419,#212420,#212421,
#212422,#212423,#212424,#212425,#212426,#212427,#212428,#212429,#212430,
#212431,#212432,#212433,#212434,#212435,#212436,#212437,#212438,#212439,
#212440,#212441,#212442,#212443,#212444,#212445,#212446,#212447,#212448,
#212449,#212450,#212451,#212452,#212453,#212454,#212455,#212456,#212457,
#212458,#212459,#212460,#212461,#212462,#212463,#212464,#212465,#212466,
#212467,#212468,#212469,#212470,#212471,#212472,#212473,#212474,#212475,
#212476,#212477,#212478)),.UNSPECIFIED.,.F.,.F.,.F.,(4,4),(4,1,1,1,1,1,
1,1,1,1,1,1,1,1,1,1,1,1,1,1,1,1,1,1,1,1,1,1,1,1,1,1,1,1,1,1,1,1,1,1,1,1,
1,1,1,1,1,1,1,1,1,1,1,1,1,1,1,1,1,1,1,1,1,1,4),(0.,1.),(0.,0.015625,0.03125,
0.046875,0.0625,0.078125,0.09375,0.109375,0.125,0.140625,0.15625,0.171875,
0.1875,0.203125,0.21875,0.234375,0.25,0.265625,0.28125,0.296875,0.3125,
0.328125,0.34375,0.359375,0.375,0.390625,0.40625,0.421875,0.4375,0.453125,
0.46875,0.484375,0.5,0.515625,0.53125,0.546875,0.5625,0.578125,0.59375,
0.609375,0.625,0.640625,0.65625,0.671875,0.6875,0.703125,0.71875,0.734375,
0.75,0.765625,0.78125,0.796875,0.8125,0.828125,0.84375,0.859375,0.875,0.890625,
0.90625,0.921875,0.9375,0.953125,0.96875,0.984375,1.),.UNSPECIFIED.);
#224=B_SPLINE_SURFACE_WITH_KNOTS('',3,3,((#212480,#212481,#212482,#212483,
#212484,#212485,#212486,#212487,#212488,#212489,#212490,#212491,#212492,
#212493,#212494,#212495,#212496,#212497,#212498,#212499,#212500,#212501,
#212502,#212503,#212504,#212505,#212506,#212507,#212508,#212509,#212510,
#212511,#212512,#212513,#212514),(#212515,#212516,#212517,#212518,#212519,
#212520,#212521,#212522,#212523,#212524,#212525,#212526,#212527,#212528,
#212529,#212530,#212531,#212532,#212533,#212534,#212535,#212536,#212537,
#212538,#212539,#212540,#212541,#212542,#212543,#212544,#212545,#212546,
#212547,#212548,#212549),(#212550,#212551,#212552,#212553,#212554,#212555,
#212556,#212557,#212558,#212559,#212560,#212561,#212562,#212563,#212564,
#212565,#212566,#212567,#212568,#212569,#212570,#212571,#212572,#212573,
#212574,#212575,#212576,#212577,#212578,#212579,#212580,#212581,#212582,
#212583,#212584),(#212585,#212586,#212587,#212588,#212589,#212590,#212591,
#212592,#212593,#212594,#212595,#212596,#212597,#212598,#212599,#212600,
#212601,#212602,#212603,#212604,#212605,#212606,#212607,#212608,#212609,
#212610,#212611,#212612,#212613,#212614,#212615,#212616,#212617,#212618,
#212619)),.UNSPECIFIED.,.F.,.F.,.F.,(4,4),(4,1,1,1,1,1,1,1,1,1,1,1,1,1,
1,1,1,1,1,1,1,1,1,1,1,1,1,1,1,1,1,1,4),(0.,1.),(0.,0.031249999999901,0.0624999999999529,
0.0937500000000048,0.125000000000057,0.156250000000109,0.187500000000009,
0.218750000000062,0.250000000000113,0.281250000000165,0.312500000000066,
0.343750000000118,0.37500000000017,0.406250000000221,0.437500000000123,
0.468750000000175,0.500000000000226,0.531250000000278,0.562500000000179,
0.593750000000231,0.625000000000283,0.656250000000335,0.687500000000236,
0.718750000000288,0.75000000000034,0.781250000000392,0.812500000000292,
0.843750000000344,0.875000000000396,0.906250000000448,0.937500000000349,
0.968750000000401,1.),.UNSPECIFIED.);
#225=B_SPLINE_SURFACE_WITH_KNOTS('',3,3,((#212696,#212697,#212698,#212699,
#212700,#212701,#212702,#212703,#212704,#212705,#212706,#212707,#212708,
#212709,#212710,#212711,#212712,#212713,#212714),(#212715,#212716,#212717,
#212718,#212719,#212720,#212721,#212722,#212723,#212724,#212725,#212726,
#212727,#212728,#212729,#212730,#212731,#212732,#212733),(#212734,#212735,
#212736,#212737,#212738,#212739,#212740,#212741,#212742,#212743,#212744,
#212745,#212746,#212747,#212748,#212749,#212750,#212751,#212752),(#212753,
#212754,#212755,#212756,#212757,#212758,#212759,#212760,#212761,#212762,
#212763,#212764,#212765,#212766,#212767,#212768,#212769,#212770,#212771)),
 .UNSPECIFIED.,.F.,.F.,.F.,(4,4),(4,1,1,1,1,1,1,1,1,1,1,1,1,1,1,1,4),(0.,
1.),(0.,0.0625,0.124999999999643,0.187499999999643,0.249999999999643,0.312499999999286,
0.374999999999286,0.437499999999286,0.499999999999286,0.562499999998929,
0.624999999998929,0.687499999998929,0.749999999998572,0.812499999998572,
0.874999999998572,0.937499999998572,1.),.UNSPECIFIED.);
#1721=FACE_BOUND('',#29289,.T.);
#1722=FACE_BOUND('',#29291,.T.);
#1723=FACE_BOUND('',#29293,.T.);
#1724=FACE_BOUND('',#29297,.T.);
#1963=CONICAL_SURFACE('',#85991,12.87032685775,0.785398346845167);
#1964=CONICAL_SURFACE('',#86011,9.75000242976401,0.785398331532869);
#1965=CONICAL_SURFACE('',#86014,9.75000242976401,0.785398331532869);
#1966=CONICAL_SURFACE('',#86035,12.87032685775,0.785398346845167);
#1967=CONICAL_SURFACE('',#86042,10.75000319972,0.785398446953936);
#1968=CONICAL_SURFACE('',#86050,7.999997663262,0.785397845123046);
#2299=CYLINDRICAL_SURFACE('',#85968,10.25);
#2300=CYLINDRICAL_SURFACE('',#85971,10.25);
#2301=CYLINDRICAL_SURFACE('',#85972,10.25);
#2302=CYLINDRICAL_SURFACE('',#85973,10.25);
#2303=CYLINDRICAL_SURFACE('',#85974,10.25);
#2304=CYLINDRICAL_SURFACE('',#85975,10.25);
#2305=CYLINDRICAL_SURFACE('',#85976,10.25);
#2306=CYLINDRICAL_SURFACE('',#85977,10.25);
#2307=CYLINDRICAL_SURFACE('',#85978,13.);
#2308=CYLINDRICAL_SURFACE('',#85980,13.);
#2309=CYLINDRICAL_SURFACE('',#85982,13.);
#2310=CYLINDRICAL_SURFACE('',#85983,13.);
#2311=CYLINDRICAL_SURFACE('',#85984,13.);
#2312=CYLINDRICAL_SURFACE('',#85985,13.);
#2313=CYLINDRICAL_SURFACE('',#85986,13.);
#2314=CYLINDRICAL_SURFACE('',#85987,13.);
#2315=CYLINDRICAL_SURFACE('',#85988,13.);
#2316=CYLINDRICAL_SURFACE('',#85993,9.09006752601109);
#2317=CYLINDRICAL_SURFACE('',#85994,9.09006752601109);
#2318=CYLINDRICAL_SURFACE('',#85995,9.09006752601109);
#2319=CYLINDRICAL_SURFACE('',#85996,9.09006752601109);
#2320=CYLINDRICAL_SURFACE('',#85997,9.0900675260086);
#2321=CYLINDRICAL_SURFACE('',#85998,9.0900675260086);
#2322=CYLINDRICAL_SURFACE('',#85999,9.0900675260086);
#2323=CYLINDRICAL_SURFACE('',#86000,9.0900675260086);
#2324=CYLINDRICAL_SURFACE('',#86001,9.08769033371916);
#2325=CYLINDRICAL_SURFACE('',#86003,11.8397710119949);
#2326=CYLINDRICAL_SURFACE('',#86005,11.8397710119949);
#2327=CYLINDRICAL_SURFACE('',#86006,11.8397710119949);
#2328=CYLINDRICAL_SURFACE('',#86007,11.8397710119877);
#2329=CYLINDRICAL_SURFACE('',#86008,11.8397710119877);
#2330=CYLINDRICAL_SURFACE('',#86009,11.8397710119877);
#2331=CYLINDRICAL_SURFACE('',#86010,11.8397710119877);
#2332=CYLINDRICAL_SURFACE('',#86016,4.75);
#2333=CYLINDRICAL_SURFACE('',#86019,11.8397710119877);
#2334=CYLINDRICAL_SURFACE('',#86020,11.8397710119949);
#2335=CYLINDRICAL_SURFACE('',#86022,10.3625);
#2336=CYLINDRICAL_SURFACE('',#86023,9.08769033371916);
#2337=CYLINDRICAL_SURFACE('',#86025,9.0900675260086);
#2338=CYLINDRICAL_SURFACE('',#86026,9.09006752601109);
#2339=CYLINDRICAL_SURFACE('',#86037,13.);
#2340=CYLINDRICAL_SURFACE('',#86038,10.5);
#2341=CYLINDRICAL_SURFACE('',#86048,7.75);
#2342=CYLINDRICAL_SURFACE('',#86053,10.25);
#2343=CYLINDRICAL_SURFACE('',#86058,10.3625);
#2697=ELLIPSE('',#86017,4.91756185694802,4.75000000000025);
#2698=ELLIPSE('',#86018,4.91756185694662,4.74999999999883);
#9646=LINE('',#203970,#16713);
#9647=LINE('',#204037,#16714);
#9648=LINE('',#204089,#16715);
#9649=LINE('',#204141,#16716);
#9650=LINE('',#204283,#16717);
#9651=LINE('',#204417,#16718);
#9652=LINE('',#204554,#16719);
#9653=LINE('',#204693,#16720);
#9654=LINE('',#204831,#16721);
#9655=LINE('',#204967,#16722);
#9656=LINE('',#205096,#16723);
#9657=LINE('',#205110,#16724);
#9658=LINE('',#205244,#16725);
#9659=LINE('',#205387,#16726);
#9660=LINE('',#205552,#16727);
#9661=LINE('',#205712,#16728);
#9662=LINE('',#205879,#16729);
#9663=LINE('',#206044,#16730);
#9664=LINE('',#206207,#16731);
#9665=LINE('',#206216,#16732);
#9666=LINE('',#206225,#16733);
#9667=LINE('',#206303,#16734);
#9668=LINE('',#206419,#16735);
#9669=LINE('',#206439,#16736);
#9670=LINE('',#206521,#16737);
#9671=LINE('',#206589,#16738);
#9672=LINE('',#206737,#16739);
#9673=LINE('',#206881,#16740);
#9674=LINE('',#206897,#16741);
#9675=LINE('',#206975,#16742);
#9676=LINE('',#207043,#16743);
#9677=LINE('',#207171,#16744);
#9678=LINE('',#207317,#16745);
#9679=LINE('',#207334,#16746);
#9680=LINE('',#207487,#16747);
#9681=LINE('',#207645,#16748);
#9682=LINE('',#207803,#16749);
#9683=LINE('',#207835,#16750);
#9684=LINE('',#207937,#16751);
#9685=LINE('',#208019,#16752);
#9686=LINE('',#208181,#16753);
#9687=LINE('',#208339,#16754);
#9688=LINE('',#208471,#16755);
#9689=LINE('',#208573,#16756);
#9690=LINE('',#208591,#16757);
#9691=LINE('',#209012,#16758);
#9692=LINE('',#209296,#16759);
#9693=LINE('',#209335,#16760);
#9694=LINE('',#209953,#16761);
#9695=LINE('',#210222,#16762);
#9696=LINE('',#210314,#16763);
#9697=LINE('',#210389,#16764);
#9698=LINE('',#211295,#16765);
#9699=LINE('',#211789,#16766);
#9700=LINE('',#212058,#16767);
#9701=LINE('',#212479,#16768);
#9702=LINE('',#212636,#16769);
#9703=LINE('',#212641,#16770);
#9704=LINE('',#212650,#16771);
#9705=LINE('',#212654,#16772);
#9706=LINE('',#212787,#16773);
#16713=VECTOR('',#106083,10.25);
#16714=VECTOR('',#106084,10.25);
#16715=VECTOR('',#106089,1000.);
#16716=VECTOR('',#106092,10.25);
#16717=VECTOR('',#106095,10.25);
#16718=VECTOR('',#106098,10.25);
#16719=VECTOR('',#106101,10.25);
#16720=VECTOR('',#106104,10.25);
#16721=VECTOR('',#106107,10.25);
#16722=VECTOR('',#106110,10.25);
#16723=VECTOR('',#106113,13.);
#16724=VECTOR('',#106118,13.);
#16725=VECTOR('',#106123,13.);
#16726=VECTOR('',#106126,13.);
#16727=VECTOR('',#106129,13.);
#16728=VECTOR('',#106132,13.);
#16729=VECTOR('',#106135,13.);
#16730=VECTOR('',#106138,13.);
#16731=VECTOR('',#106145,13.);
#16732=VECTOR('',#106146,1000.);
#16733=VECTOR('',#106147,13.);
#16734=VECTOR('',#106150,12.87032685775);
#16735=VECTOR('',#106155,9.09006752601109);
#16736=VECTOR('',#106156,10.);
#16737=VECTOR('',#106159,9.09006752601109);
#16738=VECTOR('',#106162,9.09006752601109);
#16739=VECTOR('',#106165,9.09006752601109);
#16740=VECTOR('',#106168,9.0900675260086);
#16741=VECTOR('',#106169,10.);
#16742=VECTOR('',#106172,9.0900675260086);
#16743=VECTOR('',#106175,9.0900675260086);
#16744=VECTOR('',#106178,9.0900675260086);
#16745=VECTOR('',#106181,9.08769033371916);
#16746=VECTOR('',#106186,11.8397710119949);
#16747=VECTOR('',#106191,11.8397710119949);
#16748=VECTOR('',#106194,11.8397710119949);
#16749=VECTOR('',#106197,11.8397710119877);
#16750=VECTOR('',#106198,10.);
#16751=VECTOR('',#106201,11.8397710119877);
#16752=VECTOR('',#106204,11.8397710119877);
#16753=VECTOR('',#106207,11.8397710119877);
#16754=VECTOR('',#106210,9.75000242976401);
#16755=VECTOR('',#106223,4.75);
#16756=VECTOR('',#106234,1000.);
#16757=VECTOR('',#106235,1000.);
#16758=VECTOR('',#106244,1000.);
#16759=VECTOR('',#106245,10.);
#16760=VECTOR('',#106246,10.);
#16761=VECTOR('',#106249,10.);
#16762=VECTOR('',#106250,10.);
#16763=VECTOR('',#106253,1000.);
#16764=VECTOR('',#106268,1000.);
#16765=VECTOR('',#106269,10.);
#16766=VECTOR('',#106272,10.);
#16767=VECTOR('',#106273,10.);
#16768=VECTOR('',#106276,10.);
#16769=VECTOR('',#106281,10.5);
#16770=VECTOR('',#106288,10.75000319972);
#16771=VECTOR('',#106301,7.75);
#16772=VECTOR('',#106306,7.999997663262);
#16773=VECTOR('',#106321,1000.);
#19857=PLANE('',#86027);
#19858=PLANE('',#86028);
#19859=PLANE('',#86036);
#19860=PLANE('',#86044);
#19861=PLANE('',#86045);
#19862=PLANE('',#86046);
#19863=PLANE('',#86052);
#19864=PLANE('',#86057);
#23728=FACE_OUTER_BOUND('',#29219,.T.);
#23729=FACE_OUTER_BOUND('',#29220,.T.);
#23730=FACE_OUTER_BOUND('',#29221,.T.);
#23731=FACE_OUTER_BOUND('',#29222,.T.);
#23732=FACE_OUTER_BOUND('',#29223,.T.);
#23733=FACE_OUTER_BOUND('',#29224,.T.);
#23734=FACE_OUTER_BOUND('',#29225,.T.);
#23735=FACE_OUTER_BOUND('',#29226,.T.);
#23736=FACE_OUTER_BOUND('',#29227,.T.);
#23737=FACE_OUTER_BOUND('',#29228,.T.);
#23738=FACE_OUTER_BOUND('',#29229,.T.);
#23739=FACE_OUTER_BOUND('',#29230,.T.);
#23740=FACE_OUTER_BOUND('',#29231,.T.);
#23741=FACE_OUTER_BOUND('',#29232,.T.);
#23742=FACE_OUTER_BOUND('',#29233,.T.);
#23743=FACE_OUTER_BOUND('',#29234,.T.);
#23744=FACE_OUTER_BOUND('',#29235,.T.);
#23745=FACE_OUTER_BOUND('',#29236,.T.);
#23746=FACE_OUTER_BOUND('',#29237,.T.);
#23747=FACE_OUTER_BOUND('',#29238,.T.);
#23748=FACE_OUTER_BOUND('',#29239,.T.);
#23749=FACE_OUTER_BOUND('',#29240,.T.);
#23750=FACE_OUTER_BOUND('',#29241,.T.);
#23751=FACE_OUTER_BOUND('',#29242,.T.);
#23752=FACE_OUTER_BOUND('',#29243,.T.);
#23753=FACE_OUTER_BOUND('',#29244,.T.);
#23754=FACE_OUTER_BOUND('',#29245,.T.);
#23755=FACE_OUTER_BOUND('',#29246,.T.);
#23756=FACE_OUTER_BOUND('',#29247,.T.);
#23757=FACE_OUTER_BOUND('',#29248,.T.);
#23758=FACE_OUTER_BOUND('',#29249,.T.);
#23759=FACE_OUTER_BOUND('',#29250,.T.);
#23760=FACE_OUTER_BOUND('',#29251,.T.);
#23761=FACE_OUTER_BOUND('',#29252,.T.);
#23762=FACE_OUTER_BOUND('',#29253,.T.);
#23763=FACE_OUTER_BOUND('',#29254,.T.);
#23764=FACE_OUTER_BOUND('',#29255,.T.);
#23765=FACE_OUTER_BOUND('',#29256,.T.);
#23766=FACE_OUTER_BOUND('',#29257,.T.);
#23767=FACE_OUTER_BOUND('',#29258,.T.);
#23768=FACE_OUTER_BOUND('',#29259,.T.);
#23769=FACE_OUTER_BOUND('',#29260,.T.);
#23770=FACE_OUTER_BOUND('',#29261,.T.);
#23771=FACE_OUTER_BOUND('',#29262,.T.);
#23772=FACE_OUTER_BOUND('',#29263,.T.);
#23773=FACE_OUTER_BOUND('',#29264,.T.);
#23774=FACE_OUTER_BOUND('',#29265,.T.);
#23775=FACE_OUTER_BOUND('',#29266,.T.);
#23776=FACE_OUTER_BOUND('',#29267,.T.);
#23777=FACE_OUTER_BOUND('',#29268,.T.);
#23778=FACE_OUTER_BOUND('',#29269,.T.);
#23779=FACE_OUTER_BOUND('',#29270,.T.);
#23780=FACE_OUTER_BOUND('',#29271,.T.);
#23781=FACE_OUTER_BOUND('',#29272,.T.);
#23782=FACE_OUTER_BOUND('',#29273,.T.);
#23783=FACE_OUTER_BOUND('',#29274,.T.);
#23784=FACE_OUTER_BOUND('',#29275,.T.);
#23785=FACE_OUTER_BOUND('',#29276,.T.);
#23786=FACE_OUTER_BOUND('',#29277,.T.);
#23787=FACE_OUTER_BOUND('',#29278,.T.);
#23788=FACE_OUTER_BOUND('',#29279,.T.);
#23789=FACE_OUTER_BOUND('',#29280,.T.);
#23790=FACE_OUTER_BOUND('',#29281,.T.);
#23791=FACE_OUTER_BOUND('',#29282,.T.);
#23792=FACE_OUTER_BOUND('',#29283,.T.);
#23793=FACE_OUTER_BOUND('',#29284,.T.);
#23794=FACE_OUTER_BOUND('',#29285,.T.);
#23795=FACE_OUTER_BOUND('',#29286,.T.);
#23796=FACE_OUTER_BOUND('',#29287,.T.);
#23797=FACE_OUTER_BOUND('',#29288,.T.);
#23798=FACE_OUTER_BOUND('',#29290,.T.);
#23799=FACE_OUTER_BOUND('',#29292,.T.);
#23800=FACE_OUTER_BOUND('',#29294,.T.);
#23801=FACE_OUTER_BOUND('',#29295,.T.);
#23802=FACE_OUTER_BOUND('',#29296,.T.);
#23803=FACE_OUTER_BOUND('',#29298,.T.);
#23804=FACE_OUTER_BOUND('',#29299,.T.);
#23805=FACE_OUTER_BOUND('',#29300,.T.);
#23806=FACE_OUTER_BOUND('',#29301,.T.);
#23807=FACE_OUTER_BOUND('',#29302,.T.);
#29219=EDGE_LOOP('',(#74337,#74338,#74339,#74340,#74341,#74342,#74343,#74344,
#74345,#74346,#74347,#74348,#74349));
#29220=EDGE_LOOP('',(#74350,#74351,#74352,#74353));
#29221=EDGE_LOOP('',(#74354,#74355,#74356,#74357));
#29222=EDGE_LOOP('',(#74358,#74359,#74360,#74361,#74362));
#29223=EDGE_LOOP('',(#74363,#74364,#74365,#74366,#74367));
#29224=EDGE_LOOP('',(#74368,#74369,#74370,#74371));
#29225=EDGE_LOOP('',(#74372,#74373,#74374,#74375));
#29226=EDGE_LOOP('',(#74376,#74377,#74378,#74379,#74380));
#29227=EDGE_LOOP('',(#74381,#74382,#74383));
#29228=EDGE_LOOP('',(#74384,#74385,#74386,#74387,#74388,#74389,#74390));
#29229=EDGE_LOOP('',(#74391,#74392,#74393,#74394,#74395));
#29230=EDGE_LOOP('',(#74396,#74397,#74398,#74399,#74400));
#29231=EDGE_LOOP('',(#74401,#74402,#74403,#74404));
#29232=EDGE_LOOP('',(#74405,#74406,#74407,#74408,#74409));
#29233=EDGE_LOOP('',(#74410,#74411,#74412,#74413,#74414));
#29234=EDGE_LOOP('',(#74415,#74416,#74417,#74418));
#29235=EDGE_LOOP('',(#74419,#74420,#74421,#74422,#74423,#74424,#74425,#74426,
#74427,#74428));
#29236=EDGE_LOOP('',(#74429,#74430,#74431,#74432,#74433,#74434));
#29237=EDGE_LOOP('',(#74435,#74436,#74437,#74438,#74439));
#29238=EDGE_LOOP('',(#74440,#74441,#74442,#74443));
#29239=EDGE_LOOP('',(#74444,#74445,#74446,#74447));
#29240=EDGE_LOOP('',(#74448,#74449,#74450,#74451));
#29241=EDGE_LOOP('',(#74452,#74453,#74454,#74455,#74456));
#29242=EDGE_LOOP('',(#74457,#74458,#74459,#74460));
#29243=EDGE_LOOP('',(#74461,#74462,#74463,#74464));
#29244=EDGE_LOOP('',(#74465,#74466,#74467,#74468));
#29245=EDGE_LOOP('',(#74469,#74470,#74471,#74472));
#29246=EDGE_LOOP('',(#74473,#74474,#74475,#74476));
#29247=EDGE_LOOP('',(#74477,#74478,#74479,#74480));
#29248=EDGE_LOOP('',(#74481,#74482,#74483,#74484));
#29249=EDGE_LOOP('',(#74485,#74486,#74487,#74488,#74489));
#29250=EDGE_LOOP('',(#74490,#74491,#74492,#74493));
#29251=EDGE_LOOP('',(#74494,#74495,#74496,#74497));
#29252=EDGE_LOOP('',(#74498,#74499,#74500,#74501));
#29253=EDGE_LOOP('',(#74502,#74503,#74504,#74505,#74506,#74507,#74508));
#29254=EDGE_LOOP('',(#74509,#74510,#74511));
#29255=EDGE_LOOP('',(#74512,#74513,#74514,#74515));
#29256=EDGE_LOOP('',(#74516,#74517,#74518,#74519));
#29257=EDGE_LOOP('',(#74520,#74521,#74522,#74523));
#29258=EDGE_LOOP('',(#74524,#74525,#74526,#74527,#74528));
#29259=EDGE_LOOP('',(#74529,#74530,#74531,#74532,#74533,#74534,#74535));
#29260=EDGE_LOOP('',(#74536,#74537,#74538,#74539,#74540,#74541));
#29261=EDGE_LOOP('',(#74542,#74543,#74544,#74545,#74546,#74547));
#29262=EDGE_LOOP('',(#74548,#74549,#74550,#74551));
#29263=EDGE_LOOP('',(#74552,#74553,#74554,#74555,#74556,#74557,#74558,#74559,
#74560,#74561,#74562,#74563,#74564));
#29264=EDGE_LOOP('',(#74565,#74566,#74567,#74568,#74569,#74570,#74571,#74572,
#74573,#74574,#74575,#74576,#74577));
#29265=EDGE_LOOP('',(#74578,#74579,#74580,#74581,#74582));
#29266=EDGE_LOOP('',(#74583,#74584,#74585,#74586));
#29267=EDGE_LOOP('',(#74587,#74588,#74589,#74590,#74591));
#29268=EDGE_LOOP('',(#74592,#74593,#74594,#74595,#74596,#74597,#74598,#74599,
#74600,#74601,#74602,#74603,#74604,#74605));
#29269=EDGE_LOOP('',(#74606,#74607,#74608,#74609,#74610,#74611,#74612,#74613,
#74614,#74615,#74616,#74617,#74618,#74619));
#29270=EDGE_LOOP('',(#74620,#74621,#74622,#74623,#74624,#74625,#74626,#74627));
#29271=EDGE_LOOP('',(#74628,#74629,#74630,#74631,#74632));
#29272=EDGE_LOOP('',(#74633,#74634,#74635,#74636,#74637,#74638,#74639,#74640,
#74641));
#29273=EDGE_LOOP('',(#74642,#74643,#74644));
#29274=EDGE_LOOP('',(#74645,#74646,#74647,#74648));
#29275=EDGE_LOOP('',(#74649,#74650,#74651,#74652,#74653));
#29276=EDGE_LOOP('',(#74654,#74655,#74656,#74657,#74658,#74659,#74660,#74661,
#74662,#74663,#74664,#74665));
#29277=EDGE_LOOP('',(#74666,#74667,#74668,#74669,#74670));
#29278=EDGE_LOOP('',(#74671,#74672,#74673,#74674));
#29279=EDGE_LOOP('',(#74675,#74676,#74677,#74678,#74679));
#29280=EDGE_LOOP('',(#74680,#74681,#74682,#74683,#74684,#74685,#74686,#74687,
#74688,#74689,#74690));
#29281=EDGE_LOOP('',(#74691,#74692,#74693,#74694,#74695,#74696,#74697,#74698,
#74699,#74700));
#29282=EDGE_LOOP('',(#74701,#74702,#74703,#74704,#74705,#74706,#74707,#74708,
#74709,#74710,#74711));
#29283=EDGE_LOOP('',(#74712,#74713,#74714,#74715,#74716));
#29284=EDGE_LOOP('',(#74717,#74718,#74719,#74720,#74721,#74722,#74723,#74724,
#74725,#74726));
#29285=EDGE_LOOP('',(#74727,#74728,#74729,#74730,#74731,#74732,#74733,#74734,
#74735));
#29286=EDGE_LOOP('',(#74736,#74737,#74738,#74739,#74740));
#29287=EDGE_LOOP('',(#74741,#74742,#74743,#74744,#74745));
#29288=EDGE_LOOP('',(#74746,#74747,#74748,#74749,#74750,#74751,#74752));
#29289=EDGE_LOOP('',(#74753));
#29290=EDGE_LOOP('',(#74754));
#29291=EDGE_LOOP('',(#74755));
#29292=EDGE_LOOP('',(#74756));
#29293=EDGE_LOOP('',(#74757));
#29294=EDGE_LOOP('',(#74758,#74759,#74760,#74761));
#29295=EDGE_LOOP('',(#74762,#74763,#74764,#74765));
#29296=EDGE_LOOP('',(#74766,#74767,#74768,#74769,#74770));
#29297=EDGE_LOOP('',(#74771));
#29298=EDGE_LOOP('',(#74772,#74773,#74774,#74775,#74776,#74777,#74778,#74779));
#29299=EDGE_LOOP('',(#74780,#74781,#74782,#74783,#74784,#74785,#74786,#74787,
#74788,#74789,#74790,#74791));
#29300=EDGE_LOOP('',(#74792,#74793,#74794,#74795,#74796,#74797,#74798,#74799,
#74800));
#29301=EDGE_LOOP('',(#74801,#74802,#74803,#74804));
#29302=EDGE_LOOP('',(#74805,#74806,#74807,#74808));
#30340=B_SPLINE_CURVE_WITH_KNOTS('',3,(#203972,#203973,#203974,#203975,
#203976,#203977,#203978,#203979,#203980,#203981,#203982,#203983,#203984,
#203985,#203986,#203987,#203988,#203989,#203990,#203991,#203992,#203993,
#203994,#203995,#203996,#203997,#203998,#203999,#204000,#204001,#204002,
#204003,#204004,#204005,#204006,#204007,#204008,#204009,#204010,#204011,
#204012,#204013,#204014,#204015,#204016,#204017,#204018,#204019,#204020,
#204021,#204022,#204023,#204024,#204025,#204026,#204027,#204028,#204029,
#204030,#204031,#204032,#204033,#204034,#204035),.UNSPECIFIED.,.F.,.F.,
(4,2,2,2,2,2,2,2,2,2,2,2,2,2,2,2,2,2,2,2,2,2,2,2,2,2,2,2,2,2,2,4),(-23.4687033631746,
-23.3852838488551,-23.2308554847859,-23.0393647019256,-22.8498155999754,
-22.652833031898,-22.315915647242,-22.1130911030338,-21.9105460832706,-21.8118793336342,
-21.502550365139,-21.4036127891307,-21.0871228937064,-20.9089890751837,
-20.7563727831538,-20.5652998484044,-20.3758816924102,-20.1791368906873,
-19.7735353482811,-19.3679961261668,-19.0912031493949,-18.8269861994187,
-18.682485974505,-18.4754244900494,-18.3751033651293,-18.1841021938767,
-18.0344520619974,-17.8766239737055,-17.6844266758722,-17.4946282500565,
-17.2972509069455,-17.0172746992294),.UNSPECIFIED.);
#30341=B_SPLINE_CURVE_WITH_KNOTS('',3,(#204042,#204043,#204044,#204045,
#204046,#204047,#204048,#204049,#204050,#204051,#204052,#204053,#204054,
#204055,#204056,#204057,#204058,#204059,#204060,#204061,#204062,#204063),
 .UNSPECIFIED.,.F.,.F.,(4,2,2,2,2,2,2,2,2,2,4),(-25.3610794444717,-25.215820953514,
-25.0739186005887,-24.7915033253179,-24.6197089966247,-24.4661941325765,
-24.2748584769765,-24.0853564193073,-23.8884542762642,-23.5522025045507,
-23.4687033631746),.UNSPECIFIED.);
#30342=B_SPLINE_CURVE_WITH_KNOTS('',3,(#204065,#204066,#204067,#204068,
#204069,#204070,#204071,#204072,#204073,#204074,#204075,#204076),
 .UNSPECIFIED.,.F.,.F.,(4,2,2,2,2,4),(0.,0.250779295927707,0.498420132328089,
0.665822634254374,0.997622742450792,1.33240355331691),.UNSPECIFIED.);
#30343=B_SPLINE_CURVE_WITH_KNOTS('',3,(#204078,#204079,#204080,#204081,
#204082,#204083,#204084,#204085,#204086,#204087),.UNSPECIFIED.,.F.,.F.,
(4,2,2,2,4),(1.00000001498937E-6,0.17890870313992,0.360010001015776,0.541048047587083,
0.720025159562802),.UNSPECIFIED.);
#30344=B_SPLINE_CURVE_WITH_KNOTS('',3,(#204091,#204092,#204093,#204094,
#204095,#204096,#204097,#204098,#204099,#204100),.UNSPECIFIED.,.F.,.F.,
(4,2,2,2,4),(9.72076722375712E-6,0.1792358276481,0.360521578492281,0.541895207425263,
0.721026938707022),.UNSPECIFIED.);
#30345=B_SPLINE_CURVE_WITH_KNOTS('',3,(#204102,#204103,#204104,#204105,
#204106,#204107,#204108,#204109,#204110,#204111,#204112,#204113),
 .UNSPECIFIED.,.F.,.F.,(4,2,2,2,2,4),(4.89083575497185E-5,0.33528796581701,
0.667578151924638,0.835217190795273,1.08321230565051,1.33434816674587),
 .UNSPECIFIED.);
#30346=B_SPLINE_CURVE_WITH_KNOTS('',3,(#204114,#204115,#204116,#204117,
#204118,#204119,#204120,#204121,#204122,#204123,#204124,#204125,#204126,
#204127,#204128,#204129,#204130,#204131,#204132,#204133,#204134,#204135,
#204136,#204137),.UNSPECIFIED.,.F.,.F.,(4,2,2,2,2,2,2,2,2,2,2,4),(-1.8922192761269,
-1.82208104036279,-1.72310272792682,-1.57263894437134,-1.37868950925003,
-1.09799372962318,-0.944358317890287,-0.741461864009143,-0.570015728206036,
-0.287462712367492,-0.145517952353573,-0.000222633823225556),
 .UNSPECIFIED.);
#30347=B_SPLINE_CURVE_WITH_KNOTS('',3,(#204142,#204143,#204144,#204145,
#204146,#204147,#204148,#204149,#204150,#204151,#204152,#204153,#204154,
#204155,#204156,#204157,#204158,#204159,#204160,#204161,#204162,#204163,
#204164,#204165,#204166,#204167,#204168,#204169,#204170,#204171,#204172,
#204173,#204174,#204175,#204176,#204177,#204178,#204179,#204180,#204181,
#204182,#204183,#204184,#204185,#204186,#204187,#204188,#204189,#204190,
#204191,#204192,#204193,#204194,#204195,#204196,#204197,#204198,#204199,
#204200,#204201,#204202,#204203,#204204,#204205,#204206,#204207,#204208,
#204209,#204210,#204211),.UNSPECIFIED.,.F.,.F.,(4,2,2,2,2,2,2,2,2,2,2,2,
2,2,2,2,2,2,2,2,2,2,2,2,2,2,2,2,2,2,2,2,2,2,4),(-17.0172746992294,-16.9570341593048,
-16.792101803634,-16.6373190264763,-16.4457456987925,-16.2561661420914,
-16.0591346632691,-15.7218448464861,-15.5190147192512,-15.3164628814597,
-15.1613876841587,-15.0618956354682,-14.6562439169265,-14.2510449276501,
-14.0643280509466,-13.9112414278334,-13.7081367905437,-13.549089547108,
-13.2661265111997,-13.0733681568302,-12.9227481717328,-12.8230280772896,
-12.6800940302714,-12.5372991613764,-12.3424755693224,-12.2420612363616,
-12.0263381283204,-11.8746885503234,-11.6898041466877,-11.487305003181,
-11.1798393325958,-11.000772028645,-10.7623483749487,-10.5732527961531,
-10.5668376876055),.UNSPECIFIED.);
#30348=B_SPLINE_CURVE_WITH_KNOTS('',3,(#204212,#204213,#204214,#204215,
#204216,#204217,#204218,#204219,#204220,#204221,#204222,#204223,#204224,
#204225,#204226,#204227,#204228,#204229,#204230,#204231,#204232,#204233,
#204234,#204235,#204236,#204237,#204238,#204239,#204240,#204241,#204242,
#204243,#204244,#204245,#204246,#204247,#204248,#204249,#204250,#204251,
#204252,#204253,#204254,#204255,#204256,#204257,#204258,#204259,#204260,
#204261,#204262,#204263,#204264,#204265,#204266,#204267,#204268,#204269,
#204270,#204271,#204272,#204273,#204274,#204275,#204276,#204277,#204278,
#204279),.UNSPECIFIED.,.F.,.F.,(4,2,2,2,2,2,2,2,2,2,2,2,2,2,2,2,2,2,2,2,
2,2,2,2,2,2,2,2,2,2,2,2,2,4),(-8.34223146287018,-8.2437468689296,-8.1445331304528,
-8.00277428460089,-7.90363519637987,-7.75312469070092,-7.55950114862038,
-7.27821172189581,-7.123201953391,-6.92024992819774,-6.75401545855723,-6.41641697923769,
-6.21935513267499,-6.02975645077751,-5.83812241235353,-5.68302985602848,
-5.51983283504851,-5.17607855273823,-4.77054981706035,-4.57406021893795,
-4.3847652397882,-4.19413112242747,-4.04325574447564,-3.8525494370582,-3.56528972580251,
-3.39427279588752,-3.12386295022243,-2.92760142092666,-2.73840859284267,
-2.55306289660506,-2.40680761858462,-2.16930160980798,-1.96607832439979,
-1.8922192761269),.UNSPECIFIED.);
#30349=B_SPLINE_CURVE_WITH_KNOTS('',3,(#204284,#204285,#204286,#204287,
#204288,#204289,#204290,#204291,#204292,#204293,#204294,#204295,#204296,
#204297,#204298,#204299,#204300,#204301,#204302,#204303,#204304,#204305,
#204306,#204307,#204308,#204309,#204310,#204311,#204312,#204313,#204314,
#204315,#204316,#204317,#204318,#204319,#204320,#204321,#204322,#204323,
#204324,#204325,#204326,#204327,#204328,#204329,#204330,#204331,#204332,
#204333,#204334,#204335,#204336,#204337,#204338,#204339,#204340,#204341,
#204342,#204343,#204344,#204345,#204346,#204347),.UNSPECIFIED.,.F.,.F.,
(4,2,2,2,2,2,2,2,2,2,2,2,2,2,2,2,2,2,2,2,2,2,2,2,2,2,2,2,2,2,2,4),(-10.5668376876055,
-10.3695145546731,-10.209549091418,-10.0687533668579,-9.96852459979405,
-9.81829531262626,-9.62238319389152,-9.41979214179699,-9.16391241020837,
-8.89180940188572,-8.69451601949468,-8.5047725837468,-8.3127197684882,-8.15558944526667,
-8.00275113624896,-7.81574606685221,-7.41056799669842,-7.00492097173905,
-6.90542366392111,-6.74999661874291,-6.43214336167413,-6.3331580848781,
-6.13066135698989,-5.81906147311646,-5.63291565467514,-5.47685015982526,
-5.27386467844866,-5.11127794339281,-4.7662573920237,-4.3606919703882,-4.164031884149,
-4.11510768846113),.UNSPECIFIED.);
#30350=B_SPLINE_CURVE_WITH_KNOTS('',3,(#204348,#204349,#204350,#204351,
#204352,#204353,#204354,#204355,#204356,#204357,#204358,#204359,#204360,
#204361,#204362,#204363,#204364,#204365,#204366,#204367,#204368,#204369,
#204370,#204371,#204372,#204373,#204374,#204375,#204376,#204377,#204378,
#204379,#204380,#204381,#204382,#204383,#204384,#204385,#204386,#204387,
#204388,#204389,#204390,#204391,#204392,#204393,#204394,#204395,#204396,
#204397,#204398,#204399,#204400,#204401,#204402,#204403,#204404,#204405,
#204406,#204407,#204408,#204409,#204410,#204411,#204412,#204413),
 .UNSPECIFIED.,.F.,.F.,(4,2,2,2,2,2,2,2,2,2,2,2,2,2,2,2,2,2,2,2,2,2,2,2,
2,2,2,2,2,2,2,2,4),(-14.7941896039958,-14.7907288342538,-14.6014565735193,
-14.4050047082297,-13.999485821835,-13.6559995232801,-13.4926811791532,
-13.3376171268456,-13.1187143338417,-13.0182737576245,-12.8221486482289,
-12.6797078495678,-12.5371531258208,-12.437175717494,-12.2865086245459,
-12.0941605946292,-11.8104011366496,-11.6492897792206,-11.4461076163316,
-11.299077152733,-11.1046903401399,-11.0042879555534,-10.789600296376,-10.6389655833835,
-10.4463614481799,-10.1631164110068,-10.0033311713694,-9.80020187469263,
-9.64934811132958,-9.45988021821959,-9.05486186397317,-8.64923209009487,
-8.34223146287018),.UNSPECIFIED.);
#30351=B_SPLINE_CURVE_WITH_KNOTS('',3,(#204419,#204420,#204421,#204422,
#204423,#204424,#204425,#204426,#204427,#204428,#204429,#204430,#204431,
#204432,#204433,#204434,#204435,#204436,#204437,#204438,#204439,#204440,
#204441,#204442,#204443,#204444),.UNSPECIFIED.,.F.,.F.,(4,2,2,2,2,2,2,2,
2,2,2,2,4),(-25.358128575953,-25.2282057716136,-25.1006369562764,-24.8605143713168,
-24.6990322666366,-24.4301037612475,-24.1855417081035,-23.9829494758163,
-23.7841984111289,-23.6343112149622,-23.4204024134121,-23.2450169133133,
-23.0216689529943),.UNSPECIFIED.);
#30352=B_SPLINE_CURVE_WITH_KNOTS('',3,(#204445,#204446,#204447,#204448,
#204449,#204450,#204451,#204452,#204453,#204454,#204455,#204456,#204457,
#204458,#204459,#204460,#204461,#204462,#204463,#204464,#204465,#204466,
#204467,#204468,#204469,#204470,#204471,#204472,#204473,#204474,#204475,
#204476,#204477,#204478,#204479,#204480,#204481,#204482,#204483,#204484),
 .UNSPECIFIED.,.F.,.F.,(4,2,2,2,2,2,2,2,2,2,2,2,2,2,2,2,2,2,2,4),(-4.11510768846113,
-3.97465611214066,-3.78372531762154,-3.63167160766886,-3.44970718078692,
-3.13906620947007,-3.04035407326069,-2.72332235910956,-2.62436848539607,
-2.42186942376738,-2.2191087758114,-2.01653460754979,-1.63854808421647,
-1.23292144483628,-0.827416533095915,-0.728204201083642,-0.586019509433464,
-0.293840301528918,-0.148831020870704,-5.5569436307398E-6),
 .UNSPECIFIED.);
#30353=B_SPLINE_CURVE_WITH_KNOTS('',3,(#204485,#204486,#204487,#204488,
#204489,#204490,#204491,#204492,#204493,#204494,#204495,#204496,#204497,
#204498,#204499,#204500,#204501,#204502,#204503,#204504,#204505,#204506,
#204507,#204508,#204509,#204510,#204511,#204512,#204513,#204514,#204515,
#204516,#204517,#204518,#204519,#204520,#204521,#204522,#204523,#204524,
#204525,#204526,#204527,#204528,#204529,#204530,#204531,#204532,#204533,
#204534,#204535,#204536,#204537,#204538,#204539,#204540,#204541,#204542,
#204543,#204544,#204545,#204546,#204547,#204548,#204549,#204550),
 .UNSPECIFIED.,.F.,.F.,(4,2,2,2,2,2,2,2,2,2,2,2,2,2,2,2,2,2,2,2,2,2,2,2,
2,2,2,2,2,2,2,2,4),(-21.2441617485895,-21.070587928597,-20.9234573689237,
-20.8241336310768,-20.4185450674067,-20.0459830102852,-19.8434197686704,
-19.6692135233886,-19.4663449269589,-19.2438763143868,-19.0963949961391,
-18.90938123838,-18.7201711314077,-18.5238604605068,-18.1923834699827,-18.0229719748758,
-17.8689758692299,-17.5844471973557,-17.3819988020371,-17.2827921156069,
-17.0133277526635,-16.7668635407395,-16.6212559306274,-16.4125806174337,
-16.3122464198425,-16.1205036043305,-15.9714483969571,-15.7683020315977,
-15.6079042345084,-15.324423539191,-15.1319451009706,-14.9813001926369,
-14.7941896039958),.UNSPECIFIED.);
#30354=B_SPLINE_CURVE_WITH_KNOTS('',3,(#204555,#204556,#204557,#204558,
#204559,#204560,#204561,#204562,#204563,#204564,#204565,#204566,#204567,
#204568,#204569,#204570,#204571,#204572,#204573,#204574,#204575,#204576,
#204577,#204578,#204579,#204580,#204581,#204582,#204583,#204584,#204585,
#204586,#204587,#204588,#204589,#204590,#204591,#204592,#204593,#204594,
#204595,#204596,#204597,#204598,#204599,#204600,#204601,#204602,#204603,
#204604,#204605,#204606,#204607,#204608,#204609,#204610,#204611,#204612,
#204613,#204614,#204615,#204616,#204617,#204618,#204619,#204620,#204621,
#204622),.UNSPECIFIED.,.F.,.F.,(4,2,2,2,2,2,2,2,2,2,2,2,2,2,2,2,2,2,2,2,
2,2,2,2,2,2,2,2,2,2,2,2,2,4),(-23.0216689529943,-22.9399958735644,-22.7375037591772,
-22.5521572389522,-22.4005761281261,-22.1849223594256,-22.0845124981317,
-21.8897176262462,-21.6961038208106,-21.4935285235385,-21.3206979684953,
-21.1178183959759,-20.9646317914223,-20.6841456784191,-20.490099223666,
-20.3396486032863,-20.2408119398105,-20.048836819849,-19.8462725323272,
-19.6730062813175,-19.5196477425073,-19.3284088871973,-19.1389480903071,
-18.9421137731765,-18.5365182788126,-18.2626806906338,-18.0031887816691,
-17.8006076556692,-17.6055964822867,-17.4552678130184,-17.2409037369228,
-17.0654526175782,-16.7603904867758,-16.572626139466),.UNSPECIFIED.);
#30355=B_SPLINE_CURVE_WITH_KNOTS('',3,(#204624,#204625,#204626,#204627,
#204628,#204629,#204630,#204631,#204632,#204633,#204634,#204635,#204636,
#204637,#204638,#204639,#204640,#204641,#204642,#204643,#204644,#204645,
#204646,#204647,#204648,#204649,#204650,#204651,#204652,#204653,#204654,
#204655,#204656,#204657,#204658,#204659,#204660,#204661,#204662,#204663),
 .UNSPECIFIED.,.F.,.F.,(4,2,2,2,2,2,2,2,2,2,2,2,2,2,2,2,2,2,2,4),(-25.3597291394773,
-25.2285499994245,-25.099819969673,-24.8569096210103,-24.6946723481893,
-24.3848163488543,-24.2859059766642,-23.9700785764519,-23.7915143928961,
-23.6389722847768,-23.4479188760001,-23.2585105543305,-23.0617791374454,
-22.6561917407724,-22.3106553070311,-22.1617955868105,-22.0624360532406,
-21.6568261998587,-21.2513780415546,-21.2441617485895),.UNSPECIFIED.);
#30356=B_SPLINE_CURVE_WITH_KNOTS('',3,(#204664,#204665,#204666,#204667,
#204668,#204669,#204670,#204671,#204672,#204673,#204674,#204675,#204676,
#204677,#204678,#204679,#204680,#204681,#204682,#204683,#204684,#204685,
#204686,#204687,#204688,#204689),.UNSPECIFIED.,.F.,.F.,(4,2,2,2,2,2,2,2,
2,2,2,2,4),(-2.33658628848224,-2.10644543766237,-1.91798466615612,-1.74806681040746,
-1.47807527992586,-1.28215067339681,-1.09308272844972,-0.889352076714527,
-0.730281318729365,-0.586371993056161,-0.293984893799743,-0.14890606456612,
-5.55694363607431E-6),.UNSPECIFIED.);
#30357=B_SPLINE_CURVE_WITH_KNOTS('',3,(#204694,#204695,#204696,#204697,
#204698,#204699,#204700,#204701,#204702,#204703,#204704,#204705,#204706,
#204707,#204708,#204709,#204710,#204711,#204712,#204713,#204714,#204715,
#204716,#204717,#204718,#204719,#204720,#204721,#204722,#204723,#204724,
#204725,#204726,#204727,#204728,#204729,#204730,#204731,#204732,#204733,
#204734,#204735,#204736,#204737,#204738,#204739,#204740,#204741,#204742,
#204743,#204744,#204745,#204746,#204747,#204748,#204749,#204750,#204751,
#204752,#204753,#204754,#204755,#204756,#204757,#204758,#204759),
 .UNSPECIFIED.,.F.,.F.,(4,2,2,2,2,2,2,2,2,2,2,2,2,2,2,2,2,2,2,2,2,2,2,2,
2,2,2,2,2,2,2,2,4),(-16.572626139466,-16.5579064723409,-16.4588708780629,
-16.189728250312,-16.0236918146546,-15.8358602520613,-15.6400498510376,
-15.3125659356413,-15.1409698691107,-14.987336698355,-14.7960302402308,
-14.6065447833013,-14.4096696235586,-14.0040574873121,-13.7301365342186,
-13.4704980259158,-13.2679112814905,-13.0729287155005,-12.9225917833455,
-12.8244358269876,-12.6792390808328,-12.5343267001255,-12.3468510891694,
-11.941714258584,-11.5360819504349,-11.4365769701358,-11.2806264452415,
-10.964592008435,-10.8656781544007,-10.5558023852578,-10.4571215809503,
-10.1390736746432,-10.1206942749107),.UNSPECIFIED.);
#30358=B_SPLINE_CURVE_WITH_KNOTS('',3,(#204760,#204761,#204762,#204763,
#204764,#204765,#204766,#204767,#204768,#204769,#204770,#204771,#204772,
#204773,#204774,#204775,#204776,#204777,#204778,#204779,#204780,#204781,
#204782,#204783,#204784,#204785,#204786,#204787,#204788,#204789,#204790,
#204791,#204792,#204793,#204794,#204795,#204796,#204797,#204798,#204799,
#204800,#204801,#204802,#204803,#204804,#204805,#204806,#204807,#204808,
#204809,#204810,#204811,#204812,#204813,#204814,#204815,#204816,#204817,
#204818,#204819,#204820,#204821,#204822,#204823,#204824,#204825,#204826,
#204827),.UNSPECIFIED.,.F.,.F.,(4,2,2,2,2,2,2,2,2,2,2,2,2,2,2,2,2,2,2,2,
2,2,2,2,2,2,2,2,2,2,2,2,2,4),(-8.78547365602618,-8.69348451276142,-8.5041269058269,
-8.31327657074127,-8.16156881945659,-7.97709475252234,-7.77459226543236,
-7.46494243339529,-7.28228169534135,-7.14413707085143,-6.94154150864123,
-6.69020367748547,-6.41969738046043,-6.22336323422511,-6.03413591023072,
-5.84650660349539,-5.69854632462125,-5.48123669444399,-5.27845229594527,
-5.09164011359389,-4.88915281314924,-4.59150589507809,-4.42554170215773,
-4.2606008691664,-4.05800247084799,-3.80526013087876,-3.53432581759653,
-3.33769514728129,-3.14832978216314,-2.95745696485319,-2.80566562102031,
-2.62178165020044,-2.41927475517814,-2.33658628848224),.UNSPECIFIED.);
#30359=B_SPLINE_CURVE_WITH_KNOTS('',3,(#204832,#204833,#204834,#204835,
#204836,#204837,#204838,#204839,#204840,#204841,#204842,#204843,#204844,
#204845,#204846,#204847,#204848,#204849,#204850,#204851,#204852,#204853,
#204854,#204855,#204856,#204857,#204858,#204859,#204860,#204861,#204862,
#204863,#204864,#204865,#204866,#204867,#204868,#204869,#204870,#204871,
#204872,#204873,#204874,#204875,#204876,#204877,#204878,#204879,#204880,
#204881,#204882,#204883,#204884,#204885,#204886,#204887,#204888,#204889,
#204890,#204891,#204892,#204893,#204894,#204895),.UNSPECIFIED.,.F.,.F.,
(4,2,2,2,2,2,2,2,2,2,2,2,2,2,2,2,2,2,2,2,2,2,2,2,2,2,2,2,2,2,2,4),(-10.1206942749107,
-10.0400839521642,-9.83759471021484,-9.52699477320647,-9.34264981477488,
-9.19621348106729,-8.99352683439908,-8.79166491131934,-8.5890659650105,
-8.35566614364774,-8.15254681303885,-8.0011384430874,-7.81236926147717,
-7.40730673342809,-7.00167445589182,-6.90213798484658,-6.74473748892279,
-6.43338739195136,-6.33464876950753,-6.01857571089482,-5.91965836156433,
-5.60981558607575,-5.51113398519595,-5.19302395275696,-5.09402985252356,
-4.8915360684116,-4.58119198016509,-4.39730850756027,-4.25322027900818,
-4.05057562847383,-3.83652325505148,-3.66932922096601),.UNSPECIFIED.);
#30360=B_SPLINE_CURVE_WITH_KNOTS('',3,(#204896,#204897,#204898,#204899,
#204900,#204901,#204902,#204903,#204904,#204905,#204906,#204907,#204908,
#204909,#204910,#204911,#204912,#204913,#204914,#204915,#204916,#204917,
#204918,#204919,#204920,#204921,#204922,#204923,#204924,#204925,#204926,
#204927,#204928,#204929,#204930,#204931,#204932,#204933,#204934,#204935,
#204936,#204937,#204938,#204939,#204940,#204941,#204942,#204943,#204944,
#204945,#204946,#204947,#204948,#204949,#204950,#204951,#204952,#204953,
#204954,#204955,#204956,#204957,#204958,#204959,#204960,#204961,#204962,
#204963),.UNSPECIFIED.,.F.,.F.,(4,2,2,2,2,2,2,2,2,2,2,2,2,2,2,2,2,2,2,2,
2,2,2,2,2,2,2,2,2,2,2,2,2,4),(-15.2358584380909,-14.8883885392091,-14.728212944849,
-14.5251956127154,-14.3683968473714,-14.182115397803,-13.9864134048351,
-13.6598620632904,-13.4877215195534,-13.3341662488961,-13.1166141821009,
-13.0161814909876,-12.8205979419664,-12.6780030352916,-12.5352842902373,
-12.435411099845,-12.2847577367461,-12.0922290363848,-11.8087984536162,
-11.6485680946771,-11.4454108591613,-11.2958281511512,-11.1047309033229,
-11.0044031080027,-10.7971359215093,-10.6524992354358,-10.3905358718725,
-10.1152482405395,-9.70960192401104,-9.51214685878303,-9.32229105452583,
-9.22401521382655,-8.8901013239156,-8.78547365602618),.UNSPECIFIED.);
#30361=B_SPLINE_CURVE_WITH_KNOTS('',3,(#204969,#204970,#204971,#204972,
#204973,#204974,#204975,#204976,#204977,#204978,#204979,#204980,#204981,
#204982,#204983,#204984,#204985,#204986,#204987,#204988,#204989,#204990,
#204991,#204992),.UNSPECIFIED.,.F.,.F.,(4,2,2,2,2,2,2,2,2,2,2,4),(5.07374035525052E-5,
0.196063149027679,0.390967942257574,0.792252129422216,1.19229882428634,
1.39196195962885,1.59087444470586,1.78833640693344,1.98791847080214,2.18776996778451,
2.48510060443421,2.78256740042434),.UNSPECIFIED.);
#30362=B_SPLINE_CURVE_WITH_KNOTS('',3,(#204993,#204994,#204995,#204996,
#204997,#204998,#204999,#205000,#205001,#205002,#205003,#205004,#205005,
#205006,#205007,#205008,#205009,#205010,#205011,#205012,#205013,#205014,
#205015,#205016,#205017,#205018,#205019,#205020,#205021,#205022,#205023,
#205024,#205025,#205026,#205027,#205028,#205029,#205030),.UNSPECIFIED.,
 .F.,.F.,(4,2,2,2,2,2,2,2,2,2,2,2,2,2,2,2,2,2,4),(-3.66932922096601,-3.63379619948926,
-3.43837159610714,-3.23577904909041,-2.97792121223131,-2.70491838769706,
-2.29941172035685,-2.10299660590446,-1.91373585149283,-1.72322993852301,
-1.57285025595175,-1.37821359396355,-1.09875040975318,-0.947825149927794,
-0.745015350883296,-0.562989317652314,-0.284735747904233,-0.144100026768447,
-1.91474371047745E-5),.UNSPECIFIED.);
#30363=B_SPLINE_CURVE_WITH_KNOTS('',3,(#205031,#205032,#205033,#205034,
#205035,#205036,#205037,#205038,#205039,#205040,#205041,#205042,#205043,
#205044,#205045,#205046,#205047,#205048,#205049,#205050,#205051,#205052,
#205053,#205054,#205055,#205056,#205057,#205058,#205059,#205060,#205061,
#205062,#205063,#205064,#205065,#205066,#205067,#205068,#205069,#205070,
#205071,#205072,#205073,#205074,#205075,#205076,#205077,#205078,#205079,
#205080,#205081,#205082,#205083,#205084,#205085,#205086,#205087,#205088,
#205089,#205090,#205091,#205092),.UNSPECIFIED.,.F.,.F.,(4,2,2,2,2,2,2,2,
2,2,2,2,2,2,2,2,2,2,2,2,2,2,2,2,2,2,2,2,2,2,4),(-21.689764260827,-21.5004354920718,
-21.4014712593995,-21.0843183727269,-20.9856029012984,-20.675026378304,
-20.576123130789,-20.2605890177469,-20.1044705304227,-20.0049574917496,
-19.599311014219,-19.2223904560661,-19.0198129778767,-18.8170498102401,
-18.6145467724549,-18.5155815017818,-18.1983732976846,-18.0996606679563,
-17.7891316225265,-17.6314561471473,-17.5319132563183,-17.1262842576294,
-16.7212408715178,-16.5321987154693,-16.3809997804679,-16.2235136125589,
-16.031384250264,-15.8416120625211,-15.6442728268669,-15.2386130816602,
-15.2358584380909),.UNSPECIFIED.);
#30364=B_SPLINE_CURVE_WITH_KNOTS('',3,(#205098,#205099,#205100,#205101,
#205102,#205103,#205104,#205105),.UNSPECIFIED.,.F.,.F.,(4,2,2,4),(9.21790452011069,
9.43188320060596,9.73296466447981,10.0352832224195),.UNSPECIFIED.);
#30365=B_SPLINE_CURVE_WITH_KNOTS('',3,(#205111,#205112,#205113,#205114,
#205115,#205116,#205117,#205118,#205119,#205120,#205121,#205122,#205123,
#205124,#205125,#205126,#205127,#205128,#205129,#205130,#205131,#205132,
#205133,#205134,#205135,#205136,#205137,#205138,#205139,#205140,#205141,
#205142,#205143,#205144,#205145,#205146,#205147,#205148,#205149,#205150,
#205151,#205152,#205153,#205154,#205155,#205156,#205157,#205158,#205159,
#205160,#205161,#205162,#205163,#205164,#205165,#205166,#205167,#205168,
#205169,#205170,#205171,#205172,#205173,#205174),.UNSPECIFIED.,.F.,.F.,
(4,2,2,2,2,2,2,2,2,2,2,2,2,2,2,2,2,2,2,2,2,2,2,2,2,2,2,2,2,2,2,4),(1.03510113506635,
1.42190076144482,1.65975570624358,1.90918310386553,2.03534477977229,2.54453754089879,
2.78186254656011,3.03265366633356,3.15880260896223,3.66811591822015,3.9093765188749,
4.15314502279335,4.27935426029752,4.78786109189824,5.01857442700664,5.24596204488937,
5.53988512634698,5.76236179366713,6.26691663032822,6.39333733950275,6.62191123079057,
6.74582667446146,6.99053079452599,7.33725916007856,7.58275600969113,7.82878226923088,
8.05831356871582,8.32996067834969,8.55807863234559,9.0659946634424,9.1922346984401,
9.21790452011069),.UNSPECIFIED.);
#30366=B_SPLINE_CURVE_WITH_KNOTS('',3,(#205178,#205179,#205180,#205181),
 .UNSPECIFIED.,.F.,.F.,(4,4),(0.,0.000545808001568916),.UNSPECIFIED.);
#30367=B_SPLINE_CURVE_WITH_KNOTS('',3,(#205183,#205184,#205185,#205186,
#205187,#205188,#205189,#205190,#205191,#205192,#205193,#205194,#205195,
#205196,#205197,#205198,#205199,#205200,#205201,#205202,#205203,#205204,
#205205,#205206,#205207,#205208,#205209,#205210,#205211,#205212),
 .UNSPECIFIED.,.F.,.F.,(4,2,2,2,2,2,2,2,2,2,2,2,2,2,4),(0.,0.161665978883775,
0.323391460360772,0.526063184698653,0.925852633975413,1.05183001042864,
1.56958669063238,1.76531286768935,1.96277562636044,2.47502393525148,2.70447577935272,
3.02961056722481,3.22205209759142,3.37599328488627,3.53032372881095),
 .UNSPECIFIED.);
#30368=B_SPLINE_CURVE_WITH_KNOTS('',3,(#205213,#205214,#205215,#205216,
#205217,#205218,#205219,#205220,#205221,#205222,#205223,#205224,#205225,
#205226,#205227,#205228,#205229,#205230,#205231,#205232,#205233,#205234,
#205235,#205236,#205237,#205238,#205239,#205240),.UNSPECIFIED.,.F.,.F.,
(4,2,2,2,2,2,2,2,2,2,2,2,2,4),(-4.09286724239512,-3.809817967321,-3.64049485149474,
-3.12585719629425,-2.93571507424271,-2.57217968239084,-2.39990451051648,
-1.88602332786757,-1.68187581713282,-1.33960776342174,-1.16853206857936,
-0.653965814988459,-0.343366468889826,-1.00000001346245E-6),
 .UNSPECIFIED.);
#30369=B_SPLINE_CURVE_WITH_KNOTS('',3,(#205246,#205247,#205248,#205249,
#205250,#205251,#205252,#205253,#205254,#205255,#205256,#205257,#205258,
#205259,#205260,#205261,#205262,#205263,#205264,#205265,#205266,#205267,
#205268,#205269,#205270,#205271,#205272,#205273,#205274,#205275,#205276,
#205277,#205278,#205279,#205280,#205281,#205282,#205283,#205284,#205285,
#205286,#205287,#205288,#205289,#205290,#205291,#205292,#205293,#205294,
#205295,#205296,#205297,#205298,#205299,#205300,#205301,#205302,#205303,
#205304,#205305,#205306,#205307,#205308,#205309,#205310,#205311,#205312,
#205313),.UNSPECIFIED.,.F.,.F.,(4,2,2,2,2,2,2,2,2,2,2,2,2,2,2,2,2,2,2,2,
2,2,2,2,2,2,2,2,2,2,2,2,2,4),(19.9487996122062,20.142855664464,20.3820278485055,
20.6144155244437,20.7885129097536,21.0464983427962,21.346008746776,21.4714454550556,
21.6929535544609,21.9237633529913,22.2093771833086,22.3344845972046,22.5904306859218,
22.8486338537469,22.9737744527411,23.2243002103828,23.4635057336823,23.6958961400256,
23.8701093935839,24.1280890660469,24.4283422020099,24.5537978750225,24.7778505729301,
25.0089108086963,25.3110493184325,25.4365629915189,25.6675530044301,25.9257492918385,
26.0506057192989,26.3016248087996,26.5596650416896,26.8209909987335,26.954995010501,
27.0898578193234),.UNSPECIFIED.);
#30370=B_SPLINE_CURVE_WITH_KNOTS('',3,(#205314,#205315,#205316,#205317,
#205318,#205319,#205320,#205321,#205322,#205323,#205324,#205325),
 .UNSPECIFIED.,.F.,.F.,(4,2,2,2,2,4),(4.25269675076831E-5,0.255194498558364,
0.508955632320006,0.799301344136182,0.91256206172092,1.03510113506635),
 .UNSPECIFIED.);
#30371=B_SPLINE_CURVE_WITH_KNOTS('',3,(#205326,#205327,#205328,#205329,
#205330,#205331,#205332,#205333,#205334,#205335,#205336,#205337,#205338,
#205339,#205340,#205341,#205342,#205343,#205344,#205345,#205346,#205347,
#205348,#205349,#205350,#205351,#205352,#205353,#205354,#205355,#205356,
#205357,#205358,#205359,#205360,#205361,#205362,#205363,#205364,#205365,
#205366,#205367,#205368,#205369,#205370,#205371,#205372,#205373,#205374,
#205375,#205376,#205377,#205378,#205379,#205380,#205381,#205382,#205383),
 .UNSPECIFIED.,.F.,.F.,(4,2,2,2,2,2,2,2,2,2,2,2,2,2,2,2,2,2,2,2,2,2,2,2,
2,2,2,2,4),(-12.2749063733074,-12.1187904451948,-11.8798089113104,-11.5535691718836,
-11.3094012788877,-10.8019635842849,-10.6138794912441,-10.2280063178699,
-10.0105009951333,-9.68641783018162,-9.41284063967618,-8.97177822450054,
-8.76888849823266,-8.36889877655667,-8.24292592734775,-7.88568962568576,
-7.63571172493582,-7.27227457659428,-7.02175834137767,-6.65613264294611,
-6.26737152351897,-6.07660330010159,-5.57048100512442,-5.3257325836551,
-4.99778399629202,-4.71802225801622,-4.39296620643604,-4.16592791232279,
-4.09286724239512),.UNSPECIFIED.);
#30372=B_SPLINE_CURVE_WITH_KNOTS('',3,(#205388,#205389,#205390,#205391,
#205392,#205393,#205394,#205395,#205396,#205397,#205398,#205399,#205400,
#205401,#205402,#205403,#205404,#205405,#205406,#205407,#205408,#205409,
#205410,#205411,#205412,#205413,#205414,#205415,#205416,#205417,#205418,
#205419,#205420,#205421,#205422,#205423,#205424,#205425,#205426,#205427,
#205428,#205429,#205430,#205431,#205432,#205433,#205434,#205435,#205436,
#205437,#205438,#205439,#205440,#205441,#205442,#205443,#205444,#205445,
#205446,#205447,#205448,#205449,#205450,#205451,#205452,#205453,#205454,
#205455,#205456,#205457,#205458,#205459,#205460,#205461,#205462,#205463,
#205464,#205465),.UNSPECIFIED.,.F.,.F.,(4,2,2,2,2,2,2,2,2,2,2,2,2,2,2,2,
2,2,2,2,2,2,2,2,2,2,2,2,2,2,2,2,2,2,2,2,2,2,4),(11.7724815045368,11.9880232082335,
12.2186987115618,12.4765421102483,12.6019106871588,12.8601182538573,13.0971443443364,
13.328594358856,13.5448091327034,13.7614888636755,13.9929278017894,14.2301122870459,
14.488318743795,14.6137006386228,14.8715479886744,15.1029029510991,15.3611256858989,
15.4860272745404,15.7370133629348,15.992357545874,16.2505543540056,16.3760124056608,
16.6338779445043,16.8697402281887,17.1279511122735,17.2532293185732,17.503512257197,
17.7339521368796,17.9649654333985,18.2644048003711,18.3898427277393,18.6110955292288,
18.8419052284847,19.1259978968563,19.2510812383165,19.5089682466988,19.7671789135495,
19.8923237629256,19.9487996122062),.UNSPECIFIED.);
#30373=B_SPLINE_CURVE_WITH_KNOTS('',3,(#205467,#205468,#205469,#205470,
#205471,#205472,#205473,#205474,#205475,#205476,#205477,#205478),
 .UNSPECIFIED.,.F.,.F.,(4,2,2,2,2,4),(-13.3097623343318,-13.0506231758963,
-12.7981080529111,-12.6277705686398,-12.4570074402762,-12.2749063733074),
 .UNSPECIFIED.);
#30374=B_SPLINE_CURVE_WITH_KNOTS('',3,(#205479,#205480,#205481,#205482,
#205483,#205484,#205485,#205486,#205487,#205488,#205489,#205490,#205491,
#205492,#205493,#205494,#205495,#205496,#205497,#205498,#205499,#205500,
#205501,#205502,#205503,#205504,#205505,#205506,#205507,#205508,#205509,
#205510,#205511,#205512,#205513,#205514,#205515,#205516,#205517,#205518,
#205519,#205520,#205521,#205522,#205523,#205524,#205525,#205526,#205527,
#205528,#205529,#205530,#205531,#205532,#205533,#205534,#205535,#205536,
#205537,#205538,#205539,#205540,#205541,#205542,#205543,#205544,#205545,
#205546,#205547,#205548),.UNSPECIFIED.,.F.,.F.,(4,2,2,2,2,2,2,2,2,2,2,2,
2,2,2,2,2,2,2,2,2,2,2,2,2,2,2,2,2,2,2,2,2,2,4),(-7.14122009963437,-7.10127310707761,
-6.97636086161089,-6.76788215683646,-6.51626329539109,-6.26141374359471,
-6.00319987140726,-5.87811140533219,-5.62747313366361,-5.38458271921353,
-5.12636745030447,-5.00151505431046,-4.75046058999399,-4.49223192810647,
-4.23405928698162,-4.10848089710744,-3.85059081999491,-3.5842634917128,
-3.33942218792414,-3.08877078337361,-2.96290962115914,-2.66718399600173,
-2.54184986425145,-2.31676961113023,-2.08596597217156,-1.80509407491701,
-1.68006608005489,-1.42222650442997,-1.16402119388851,-1.03914810583125,
-0.788143072776472,-0.530949948001708,-0.269269866189475,-0.135098326930044,
-6.79217263228586E-5),.UNSPECIFIED.);
#30375=B_SPLINE_CURVE_WITH_KNOTS('',3,(#205553,#205554,#205555,#205556,
#205557,#205558,#205559,#205560,#205561,#205562,#205563,#205564,#205565,
#205566,#205567,#205568,#205569,#205570,#205571,#205572,#205573,#205574,
#205575,#205576,#205577,#205578,#205579,#205580,#205581,#205582,#205583,
#205584,#205585,#205586,#205587,#205588,#205589,#205590,#205591,#205592,
#205593,#205594,#205595,#205596,#205597,#205598,#205599,#205600,#205601,
#205602,#205603,#205604,#205605,#205606,#205607,#205608,#205609,#205610,
#205611,#205612,#205613,#205614,#205615,#205616,#205617,#205618,#205619,
#205620,#205621,#205622,#205623,#205624,#205625,#205626,#205627,#205628,
#205629,#205630,#205631,#205632),.UNSPECIFIED.,.F.,.F.,(4,2,2,2,2,2,2,2,
2,2,2,2,2,2,2,2,2,2,2,2,2,2,2,2,2,2,2,2,2,2,2,2,2,2,2,2,2,2,2,4),(3.59627226695956,
3.6820600167183,3.80682696477215,4.06503601396435,4.32286613510125,4.44787779959693,
4.72748981290888,4.85322792225321,5.10340879996836,5.34812827344507,5.61203495282972,
5.86991733555808,5.99546211326746,6.25364136016089,6.49309994339892,6.75097551172211,
6.87648804579222,7.13467380487495,7.37367211565911,7.63154747763148,7.7986701016379,
8.03053802827694,8.2746699170043,8.39982470434024,8.68749696161902,8.94546076267652,
9.11758260107282,9.34982456475858,9.59575501121538,9.84716629837951,10.0584626241018,
10.1833748416066,10.4528951173875,10.7108031723359,10.8364283644821,11.0945998805693,
11.3538735001863,11.6049615553723,11.7298011915162,11.7724815045368),
 .UNSPECIFIED.);
#30376=B_SPLINE_CURVE_WITH_KNOTS('',3,(#205633,#205634,#205635,#205636,
#205637,#205638,#205639,#205640,#205641,#205642,#205643,#205644,#205645,
#205646,#205647,#205648,#205649,#205650,#205651,#205652,#205653,#205654,
#205655,#205656,#205657,#205658,#205659,#205660,#205661,#205662,#205663,
#205664,#205665,#205666,#205667,#205668,#205669,#205670,#205671,#205672,
#205673,#205674,#205675,#205676,#205677,#205678,#205679,#205680,#205681,
#205682,#205683,#205684,#205685,#205686,#205687,#205688,#205689,#205690,
#205691,#205692,#205693,#205694,#205695,#205696,#205697,#205698,#205699,
#205700,#205701,#205702,#205703,#205704,#205705,#205706,#205707,#205708),
 .UNSPECIFIED.,.F.,.F.,(4,2,2,2,2,2,2,2,2,2,2,2,2,2,2,2,2,2,2,2,2,2,2,2,
2,2,2,2,2,2,2,2,2,2,2,2,2,4),(-15.317600608495,-15.1056219580742,-14.8722513427225,
-14.6143963369378,-14.4889800020028,-14.2307783488225,-13.99312958769,-13.7617239607727,
-13.544813767322,-13.328495618661,-13.0970771655347,-12.8596184019178,-12.601415245543,
-12.4760144538482,-12.2181639986697,-11.9856237537738,-11.7274032423102,
-11.6023998741531,-11.3515970506217,-11.1029633060686,-10.8447459947707,
-10.7196010603171,-10.4690595259377,-10.2297444117701,-9.9973186109037,
-9.82280774939264,-9.56481055125628,-9.26273553467217,-9.13721415315108,
-8.90657398144562,-8.64835908946668,-8.52352550164255,-8.27243999430361,
-8.01300468974959,-7.75484166851552,-7.6292129323572,-7.3713101840488,-7.14122009963437),
 .UNSPECIFIED.);
#30377=B_SPLINE_CURVE_WITH_KNOTS('',3,(#205714,#205715,#205716,#205717,
#205718,#205719,#205720,#205721,#205722,#205723,#205724,#205725,#205726,
#205727,#205728,#205729,#205730,#205731,#205732,#205733,#205734,#205735,
#205736,#205737,#205738,#205739,#205740,#205741,#205742,#205743,#205744,
#205745,#205746,#205747,#205748,#205749,#205750,#205751,#205752,#205753,
#205754,#205755,#205756,#205757,#205758,#205759),.UNSPECIFIED.,.F.,.F.,
(4,2,2,2,2,2,2,2,2,2,2,2,2,2,2,2,2,2,2,2,2,2,4),(-27.0910624136568,-26.9485297956287,
-26.8071562305741,-26.5294229406298,-26.3120852980215,-26.0764565382135,
-25.8991731920804,-25.6664808600428,-25.4263379769398,-25.1757865161133,
-25.013524286709,-24.8875050591639,-24.6363094106816,-24.3912847026917,
-24.1219528354226,-23.8909880111037,-23.6725325990257,-23.438024623467,
-23.2587214500234,-23.1324894158539,-22.7613668132535,-22.6364211647448,
-22.5113746151152),.UNSPECIFIED.);
#30378=B_SPLINE_CURVE_WITH_KNOTS('',3,(#205760,#205761,#205762,#205763,
#205764,#205765,#205766,#205767,#205768,#205769,#205770,#205771,#205772,
#205773,#205774,#205775,#205776,#205777,#205778,#205779,#205780,#205781,
#205782,#205783,#205784,#205785,#205786,#205787,#205788,#205789,#205790,
#205791,#205792,#205793,#205794,#205795),.UNSPECIFIED.,.F.,.F.,(4,2,2,2,
2,2,2,2,2,2,2,2,2,2,2,2,2,4),(6.63670082959331E-6,0.138847337507348,0.276650112027392,
0.546239332473065,0.724776399663302,0.98298432656475,1.22509099349884,1.47570301961592,
1.60079692900476,1.8590027850634,2.11687597018492,2.24194740912891,2.52544615201078,
2.78338592312406,2.90917826586352,3.16729181898307,3.43087394279093,3.59627226695956),
 .UNSPECIFIED.);
#30379=B_SPLINE_CURVE_WITH_KNOTS('',3,(#205796,#205797,#205798,#205799,
#205800,#205801,#205802,#205803,#205804,#205805,#205806,#205807,#205808,
#205809,#205810,#205811,#205812,#205813,#205814,#205815,#205816,#205817,
#205818,#205819,#205820,#205821,#205822,#205823,#205824,#205825,#205826,
#205827,#205828,#205829,#205830,#205831,#205832,#205833,#205834,#205835,
#205836,#205837,#205838,#205839,#205840,#205841,#205842,#205843,#205844,
#205845,#205846,#205847,#205848,#205849,#205850,#205851,#205852,#205853,
#205854,#205855,#205856,#205857,#205858,#205859,#205860,#205861,#205862,
#205863,#205864,#205865,#205866,#205867,#205868,#205869,#205870,#205871,
#205872,#205873,#205874,#205875),.UNSPECIFIED.,.F.,.F.,(4,2,2,2,2,2,2,2,
2,2,2,2,2,2,2,2,2,2,2,2,2,2,2,2,2,2,2,2,2,2,2,2,2,2,2,2,2,2,2,4),(-23.4937717245981,
-23.4149622474878,-23.2518531829715,-23.0202626120369,-22.7851106159285,
-22.5346906323585,-22.4094834242548,-22.151270805228,-21.9013492411497,
-21.6505124378202,-21.5255288848259,-21.2673100902392,-21.0094439097838,
-20.7573343531256,-20.5557090153031,-20.4307869371161,-20.1594159310078,
-19.9015048799453,-19.7758559447382,-19.5176942020619,-19.2578307792033,
-19.0067304919821,-18.8819009556285,-18.623682631028,-18.3812729116814,
-18.1306445818583,-18.0055462446488,-17.7473293917388,-17.5136733528107,
-17.2558191980766,-17.1303989826605,-16.8721999568476,-16.6176890754392,
-16.3667268578538,-16.2418132831234,-15.9835923810468,-15.7395918633547,
-15.488916783225,-15.363841527225,-15.317600608495),.UNSPECIFIED.);
#30380=B_SPLINE_CURVE_WITH_KNOTS('',3,(#205880,#205881,#205882,#205883,
#205884,#205885,#205886,#205887,#205888,#205889,#205890,#205891,#205892,
#205893,#205894,#205895,#205896,#205897,#205898,#205899,#205900,#205901,
#205902,#205903,#205904,#205905,#205906,#205907,#205908,#205909,#205910,
#205911,#205912,#205913,#205914,#205915,#205916,#205917,#205918,#205919,
#205920,#205921,#205922,#205923,#205924,#205925,#205926,#205927,#205928,
#205929,#205930,#205931,#205932,#205933,#205934,#205935,#205936,#205937,
#205938,#205939,#205940,#205941,#205942,#205943,#205944,#205945,#205946,
#205947,#205948,#205949,#205950,#205951,#205952,#205953,#205954,#205955,
#205956,#205957),.UNSPECIFIED.,.F.,.F.,(4,2,2,2,2,2,2,2,2,2,2,2,2,2,2,2,
2,2,2,2,2,2,2,2,2,2,2,2,2,2,2,2,2,2,2,2,2,2,4),(-22.5113746151152,-22.3622013116186,
-22.2365061539233,-21.9295000211994,-21.8035549222477,-21.5526094311646,
-21.3076712345341,-21.039790083002,-20.7818879132803,-20.6562842093903,
-20.3981100668058,-20.1393696152133,-19.8882954198129,-19.763446951026,
-19.5052254143252,-19.2624813513231,-19.0118407093092,-18.8867459155375,
-18.6285258780502,-18.3809498202434,-18.1301741601724,-18.0051528863069,
-17.7469311137219,-17.4890562011227,-17.2369979097946,-17.0345635881456,
-16.9096411105631,-16.63842716538,-16.3805132473707,-16.2548647611498,-15.9966991588529,
-15.7368835496313,-15.4857812656124,-15.3609492874221,-15.1027275466364,
-14.8721471489679,-14.6143039871265,-14.4889361920765,-14.3348679765578),
 .UNSPECIFIED.);
#30381=B_SPLINE_CURVE_WITH_KNOTS('',3,(#205959,#205960,#205961,#205962,
#205963,#205964,#205965,#205966,#205967,#205968,#205969,#205970,#205971,
#205972,#205973,#205974,#205975,#205976,#205977,#205978,#205979,#205980,
#205981,#205982,#205983,#205984,#205985,#205986,#205987,#205988,#205989,
#205990,#205991,#205992,#205993,#205994),.UNSPECIFIED.,.F.,.F.,(4,2,2,2,
2,2,2,2,2,2,2,2,2,2,2,2,2,4),(-27.0899870889368,-26.9530598593633,-26.8171091942596,
-26.5516008514074,-26.3748538499552,-26.1166597858708,-25.8789718218379,
-25.6475129080143,-25.4306415300505,-25.3052641631091,-25.0079344600063,
-24.776962792956,-24.5470734614413,-24.2968096085422,-24.1326327675215,
-23.9009712650346,-23.6653943076616,-23.4937717245981),.UNSPECIFIED.);
#30382=B_SPLINE_CURVE_WITH_KNOTS('',3,(#205995,#205996,#205997,#205998,
#205999,#206000,#206001,#206002,#206003,#206004,#206005,#206006,#206007,
#206008,#206009,#206010,#206011,#206012,#206013,#206014,#206015,#206016,
#206017,#206018,#206019,#206020,#206021,#206022,#206023,#206024,#206025,
#206026,#206027,#206028,#206029,#206030,#206031,#206032,#206033,#206034,
#206035,#206036,#206037,#206038,#206039,#206040),.UNSPECIFIED.,.F.,.F.,
(4,2,2,2,2,2,2,2,2,2,2,2,2,2,2,2,2,2,2,2,2,2,4),(-4.57954798347794,-4.51040613143666,
-4.27892855829839,-4.11745185319605,-3.86677760228649,-3.62237827806238,
-3.36416946717782,-3.23924161777639,-2.98832792653369,-2.73518719314125,
-2.4769938688065,-2.35164184692701,-2.09381583051975,-1.86367735928636,
-1.60547069925905,-1.4806851661486,-1.22953536858346,-0.967443934401527,
-0.709310837623982,-0.533692325490634,-0.270605510121337,-0.135776812330919,
-3.84812749395499E-6),.UNSPECIFIED.);
#30383=B_SPLINE_CURVE_WITH_KNOTS('',3,(#206045,#206046,#206047,#206048,
#206049,#206050,#206051,#206052,#206053,#206054,#206055,#206056,#206057,
#206058,#206059,#206060,#206061,#206062,#206063,#206064,#206065,#206066,
#206067,#206068,#206069,#206070,#206071,#206072,#206073,#206074,#206075,
#206076,#206077,#206078,#206079,#206080,#206081,#206082,#206083,#206084,
#206085,#206086,#206087,#206088,#206089,#206090,#206091,#206092,#206093,
#206094,#206095,#206096,#206097,#206098,#206099,#206100,#206101,#206102,
#206103,#206104,#206105,#206106,#206107,#206108,#206109,#206110,#206111,
#206112,#206113,#206114,#206115,#206116,#206117,#206118,#206119,#206120,
#206121,#206122),.UNSPECIFIED.,.F.,.F.,(4,2,2,2,2,2,2,2,2,2,2,2,2,2,2,2,
2,2,2,2,2,2,2,2,2,2,2,2,2,2,2,2,2,2,2,2,2,2,4),(-14.3348679765578,-14.2307291371401,
-13.9937264081978,-13.7622752350275,-13.5460663942738,-13.3293994027905,
-13.0979594006491,-12.8607996474343,-12.6025935681271,-12.4772150610294,
-12.2193696239954,-11.9881213265458,-11.7298995835503,-11.605008893432,
-11.3540079235617,-11.0980479583536,-10.8398545998019,-10.7143709190112,
-10.4564996619228,-10.2189743116877,-9.96077385475969,-9.83536896601102,
-9.57751937674932,-9.3446829071744,-9.08646492332606,-8.96143705944965,
-8.71068232766445,-8.4637182852313,-8.2055010592925,-8.08043922563878,-7.8297466815448,
-7.58501360152563,-7.32679533589724,-7.20184622275508,-6.95095231324976,
-6.69888065047845,-6.44067411083485,-6.31536707642487,-6.15860212849669),
 .UNSPECIFIED.);
#30384=B_SPLINE_CURVE_WITH_KNOTS('',3,(#206123,#206124,#206125,#206126,
#206127,#206128,#206129,#206130,#206131,#206132,#206133,#206134,#206135,
#206136,#206137,#206138,#206139,#206140,#206141,#206142,#206143,#206144,
#206145,#206146,#206147,#206148,#206149,#206150,#206151,#206152,#206153,
#206154,#206155,#206156,#206157,#206158,#206159,#206160,#206161,#206162,
#206163,#206164,#206165,#206166,#206167,#206168,#206169,#206170,#206171,
#206172,#206173,#206174,#206175,#206176,#206177,#206178,#206179,#206180,
#206181,#206182,#206183,#206184,#206185,#206186,#206187,#206188,#206189,
#206190,#206191,#206192,#206193,#206194,#206195,#206196,#206197,#206198,
#206199,#206200),.UNSPECIFIED.,.F.,.F.,(4,2,2,2,2,2,2,2,2,2,2,2,2,2,2,2,
2,2,2,2,2,2,2,2,2,2,2,2,2,2,2,2,2,2,2,2,2,2,4),(-12.7553611554937,-12.6017145941975,
-12.4763762122337,-12.2185474892998,-11.9893326254508,-11.7567223866939,
-11.5798310036023,-11.3436886696159,-11.1266310767901,-10.895255140734,
-10.6572994907987,-10.3991097311077,-10.2736757350015,-10.0158250513052,
-9.78107512198834,-9.52286890232859,-9.39768468763165,-9.14723654608586,
-8.91085699546733,-8.67905773239113,-8.51279779148808,-8.25494725044977,
-8.01983611288601,-7.76163292372143,-7.63642023060741,-7.38603097600229,
-7.15161907456632,-6.92015153602238,-6.75884077192061,-6.50814063174183,
-6.26282945460571,-6.00462037579504,-5.87964569336017,-5.62881318350843,
-5.37869162359585,-5.12048884010234,-4.99527739343617,-4.74488656402094,
-4.57954798347794),.UNSPECIFIED.);
#30385=B_SPLINE_CURVE_WITH_KNOTS('',3,(#206209,#206210,#206211,#206212,
#206213,#206214),.UNSPECIFIED.,.F.,.F.,(4,2,4),(1.00000001053189E-6,0.291982877240883,
0.583963182531396),.UNSPECIFIED.);
#30386=B_SPLINE_CURVE_WITH_KNOTS('',3,(#206218,#206219,#206220,#206221,
#206222,#206223),.UNSPECIFIED.,.F.,.F.,(4,2,4),(1.18860081555568E-5,0.292247563585408,
0.584494052040901),.UNSPECIFIED.);
#30387=B_SPLINE_CURVE_WITH_KNOTS('',3,(#206227,#206228,#206229,#206230,
#206231,#206232,#206233,#206234,#206235,#206236,#206237,#206238,#206239,
#206240,#206241,#206242,#206243,#206244,#206245,#206246,#206247,#206248,
#206249,#206250,#206251,#206252,#206253,#206254,#206255,#206256,#206257,
#206258,#206259,#206260,#206261,#206262,#206263,#206264,#206265,#206266,
#206267,#206268,#206269,#206270,#206271,#206272,#206273,#206274,#206275,
#206276,#206277,#206278,#206279,#206280,#206281,#206282,#206283,#206284,
#206285,#206286),.UNSPECIFIED.,.F.,.F.,(4,2,2,2,2,2,2,2,2,2,2,2,2,2,2,2,
2,2,2,2,2,2,2,2,2,2,2,2,2,4),(-27.088923764392,-26.950639491994,-26.8133525669105,
-26.544907036575,-26.3668620021181,-26.108660746686,-25.8508123833913,-25.7257678773642,
-25.4436361357283,-25.1857075525708,-25.0145798547139,-24.8884489823397,
-24.5204161698867,-24.3954710664388,-24.1209093810336,-23.86300038075,-23.6932540021783,
-23.461206206101,-23.2161229095314,-22.9647484897821,-22.7531956056424,
-22.6282932069822,-22.3588407689814,-22.1009488738442,-21.9753313793407,
-21.717177140173,-21.4579376178504,-21.2068654511702,-21.082032595878,-20.9312459291626),
 .UNSPECIFIED.);
#30388=B_SPLINE_CURVE_WITH_KNOTS('',3,(#206287,#206288,#206289,#206290,
#206291,#206292,#206293,#206294,#206295,#206296,#206297,#206298,#206299,
#206300),.UNSPECIFIED.,.F.,.F.,(4,2,2,2,2,2,4),(0.,0.254132792260243,0.504072118513533,
1.01015766536926,1.26037994975052,1.64270580735409,2.01988313929201),
 .UNSPECIFIED.);
#30389=B_SPLINE_CURVE_WITH_KNOTS('',3,(#206305,#206306,#206307,#206308),
 .UNSPECIFIED.,.F.,.F.,(4,4),(-0.00220042394823992,0.),.UNSPECIFIED.);
#30390=B_SPLINE_CURVE_WITH_KNOTS('',3,(#206310,#206311,#206312,#206313,
#206314,#206315,#206316,#206317,#206318,#206319,#206320,#206321,#206322,
#206323,#206324,#206325,#206326,#206327,#206328,#206329,#206330,#206331,
#206332,#206333,#206334,#206335,#206336,#206337,#206338,#206339,#206340,
#206341,#206342,#206343,#206344,#206345,#206346,#206347,#206348,#206349,
#206350,#206351,#206352,#206353,#206354,#206355),.UNSPECIFIED.,.F.,.F.,
(4,2,2,2,2,2,2,2,2,2,2,2,2,2,2,2,2,2,2,2,2,2,4),(3.77495847620787E-5,0.239786601820601,
0.486605707253356,0.970538667061549,1.45703768164805,1.71085426685705,1.9510783074641,
2.07349206054835,2.55160936918151,2.80110529120666,3.03699522422384,3.28275824999066,
3.52002970929671,3.76617821420918,4.00121882590241,4.49262572156392,4.61272242555606,
4.85423743096944,5.08785380877291,5.57193736666279,6.05829820485225,6.18384427889897,
6.56939833044204),.UNSPECIFIED.);
#30391=B_SPLINE_CURVE_WITH_KNOTS('',3,(#206358,#206359,#206360,#206361,
#206362,#206363,#206364,#206365,#206366,#206367,#206368,#206369,#206370,
#206371,#206372,#206373,#206374,#206375,#206376,#206377,#206378,#206379,
#206380,#206381,#206382,#206383,#206384,#206385,#206386,#206387,#206388,
#206389,#206390,#206391,#206392,#206393,#206394,#206395,#206396,#206397,
#206398,#206399,#206400,#206401,#206402,#206403,#206404,#206405,#206406,
#206407,#206408,#206409,#206410,#206411,#206412,#206413,#206414,#206415),
 .UNSPECIFIED.,.F.,.F.,(4,3,3,3,3,3,3,3,3,3,3,3,3,3,3,3,3,3,3,4),(0.,0.0577023232576086,
0.115555621115906,0.173492165360545,0.231551782116938,0.25,0.307569756346692,
0.365075787326178,0.422538236884358,0.479957516808789,0.537334036195474,
0.594651018367717,0.651929822766841,0.709155453145986,0.75,0.807257177142689,
0.864351407537183,0.921347999936588,0.978207659355297,0.999999816562461),
 .UNSPECIFIED.);
#30392=B_SPLINE_CURVE_WITH_KNOTS('',3,(#206421,#206422,#206423,#206424),
 .UNSPECIFIED.,.F.,.F.,(4,4),(-6.83645232667685E-6,-1.00000001587719E-6),
 .UNSPECIFIED.);
#30393=B_SPLINE_CURVE_WITH_KNOTS('',3,(#206426,#206427,#206428,#206429,
#206430,#206431,#206432,#206433,#206434,#206435,#206436,#206437),
 .UNSPECIFIED.,.F.,.F.,(4,2,2,2,2,4),(0.000339869836820149,0.296752020291076,
0.39447181405845,0.493164400823495,0.639110988050355,0.788070724201917),
 .UNSPECIFIED.);
#30394=B_SPLINE_CURVE_WITH_KNOTS('',3,(#206440,#206441,#206442,#206443,
#206444,#206445,#206446,#206447,#206448,#206449,#206450,#206451),
 .UNSPECIFIED.,.F.,.F.,(4,2,2,2,2,4),(-0.787810247909609,-0.491424601924294,
-0.393707156562174,-0.29503529184239,-0.149115943288715,-9.76537854778592E-5),
 .UNSPECIFIED.);
#30395=B_SPLINE_CURVE_WITH_KNOTS('',3,(#206454,#206455,#206456,#206457,
#206458,#206459,#206460,#206461,#206462,#206463,#206464,#206465,#206466,
#206467,#206468,#206469,#206470,#206471,#206472,#206473,#206474,#206475,
#206476,#206477,#206478,#206479,#206480,#206481,#206482,#206483,#206484,
#206485,#206486,#206487,#206488,#206489,#206490,#206491,#206492,#206493,
#206494,#206495,#206496,#206497,#206498,#206499,#206500,#206501,#206502,
#206503,#206504,#206505,#206506,#206507,#206508,#206509,#206510,#206511,
#206512,#206513,#206514,#206515,#206516,#206517,#206518,#206519),
 .UNSPECIFIED.,.F.,.F.,(4,2,2,2,2,2,2,2,2,2,2,2,2,2,2,2,2,2,2,2,2,2,2,2,
2,2,2,2,2,2,2,2,4),(-20.0251822700621,-19.783399253692,-19.7027995529101,
-19.3819220086887,-19.2335279991671,-19.0806295483898,-18.9217357990387,
-18.8325340301694,-18.6562482399521,-18.4948478066825,-18.3256422331843,
-18.173550209753,-17.9918384866733,-17.8262128753862,-17.7375272992725,
-17.5586636565654,-17.3917395152,-17.2468299270429,-17.0904651127749,-16.9212870128186,
-16.7510701900917,-16.4818730929832,-16.3432229200778,-16.1264751872471,
-15.947096589243,-15.7717268657687,-15.6306011902255,-15.4602842612329,
-15.2908239990938,-15.1162436454238,-14.756984936882,-14.3959660136892,
-14.3036677916835),.UNSPECIFIED.);
#30396=B_SPLINE_CURVE_WITH_KNOTS('',3,(#206522,#206523,#206524,#206525,
#206526,#206527,#206528,#206529,#206530,#206531,#206532,#206533,#206534,
#206535,#206536,#206537,#206538,#206539,#206540,#206541,#206542,#206543,
#206544,#206545,#206546,#206547,#206548,#206549,#206550,#206551,#206552,
#206553,#206554,#206555,#206556,#206557,#206558,#206559,#206560,#206561,
#206562,#206563,#206564,#206565,#206566,#206567,#206568,#206569,#206570,
#206571,#206572,#206573,#206574,#206575,#206576,#206577,#206578,#206579,
#206580,#206581,#206582,#206583,#206584,#206585),.UNSPECIFIED.,.F.,.F.,
(4,2,2,2,2,2,2,2,2,2,2,2,2,2,2,2,2,2,2,2,2,2,2,2,2,2,2,2,2,2,2,4),(-5.72191210760107,
-5.41349515739714,-5.05567096156071,-4.96749892296319,-4.81840590942988,
-4.63859224637836,-4.45820907173672,-4.18760610519457,-4.09983054832184,
-3.79969878315938,-3.44429584089838,-3.27068421004476,-3.10024231552191,
-2.92994627866288,-2.76951740584553,-2.62353240632635,-2.46635235484725,
-2.28748261501643,-2.19879437053061,-2.03356792410285,-1.85427977681009,
-1.70336284067883,-1.51995057865207,-1.36630179602626,-1.19012013778883,
-1.10095232118681,-0.94005746713909,-0.759230972609438,-0.616488683133836,
-0.385776320856448,-0.195646578274231,-6.83645232667685E-6),
 .UNSPECIFIED.);
#30397=B_SPLINE_CURVE_WITH_KNOTS('',3,(#206590,#206591,#206592,#206593,
#206594,#206595,#206596,#206597,#206598,#206599,#206600,#206601,#206602,
#206603,#206604,#206605,#206606,#206607,#206608,#206609,#206610,#206611,
#206612,#206613,#206614,#206615,#206616,#206617,#206618,#206619,#206620,
#206621,#206622,#206623,#206624,#206625,#206626,#206627,#206628,#206629,
#206630,#206631,#206632,#206633,#206634,#206635,#206636,#206637,#206638,
#206639,#206640,#206641,#206642,#206643,#206644,#206645,#206646,#206647,
#206648,#206649,#206650,#206651,#206652,#206653,#206654,#206655,#206656,
#206657,#206658,#206659,#206660,#206661,#206662,#206663),.UNSPECIFIED.,
 .F.,.F.,(4,2,2,2,2,2,2,2,2,2,2,2,2,2,2,2,2,2,2,2,2,2,2,2,2,2,2,2,2,2,2,
2,2,2,2,2,4),(-11.4417380987961,-11.3553364651864,-11.1774160383949,-11.0372075791858,
-10.8667631656153,-10.6973773346602,-10.5226016322737,-10.2477974621797,
-10.0995357553595,-10.0114468986988,-9.65549049338967,-9.48138958945092,
-9.31089325773942,-9.14006813818346,-8.98157553049582,-8.82713166956379,
-8.68104046619338,-8.50127889414351,-8.41281799829901,-8.24999629874056,
-8.08982187212831,-7.94014904278731,-7.62303054035336,-7.5348458585733,
-7.39685004091648,-7.21874574487305,-7.04217836617445,-6.95300076868866,
-6.79472871579089,-6.63547366518565,-6.48774654885689,-6.31196696168113,
-6.22263750831177,-6.07312396277187,-5.9302570348509,-5.7687427317654,-5.72191210760107),
 .UNSPECIFIED.);
#30398=B_SPLINE_CURVE_WITH_KNOTS('',3,(#206664,#206665,#206666,#206667,
#206668,#206669,#206670,#206671,#206672,#206673,#206674,#206675,#206676,
#206677,#206678,#206679,#206680,#206681,#206682,#206683,#206684,#206685,
#206686,#206687,#206688,#206689,#206690,#206691,#206692,#206693,#206694,
#206695,#206696,#206697,#206698,#206699,#206700,#206701,#206702,#206703,
#206704,#206705,#206706,#206707,#206708,#206709,#206710,#206711,#206712,
#206713,#206714,#206715,#206716,#206717,#206718,#206719,#206720,#206721,
#206722,#206723,#206724,#206725,#206726,#206727,#206728,#206729,#206730,
#206731,#206732,#206733),.UNSPECIFIED.,.F.,.F.,(4,2,2,2,2,2,2,2,2,2,2,2,
2,2,2,2,2,2,2,2,2,2,2,2,2,2,2,2,2,2,2,2,2,2,4),(-14.3036677916835,-14.0340394295821,
-13.7520315188632,-13.5974111949159,-13.4400684067818,-13.3508209983375,
-13.1749381983995,-12.9996246650309,-12.8581361268037,-12.7010224181862,
-12.5108779886259,-12.3442110009737,-12.2554161351745,-12.07716356736,-11.9192026641883,
-11.76735048996,-11.6082372190042,-11.5197094013378,-11.3400263407629,-11.1895026213211,
-11.0407835689815,-10.8835502767979,-10.7128843788238,-10.5424684480171,
-10.3684595925684,-10.0124870321069,-9.92436933678178,-9.76328708361137,
-9.58305914112651,-9.3895913390335,-9.20952067832326,-9.04285406091558,
-8.78771294563985,-8.61662518543304,-8.58288598458152),.UNSPECIFIED.);
#30399=B_SPLINE_CURVE_WITH_KNOTS('',3,(#206738,#206739,#206740,#206741,
#206742,#206743,#206744,#206745,#206746,#206747,#206748,#206749,#206750,
#206751,#206752,#206753,#206754,#206755,#206756,#206757,#206758,#206759,
#206760,#206761,#206762,#206763,#206764,#206765,#206766,#206767,#206768,
#206769,#206770,#206771,#206772,#206773,#206774,#206775,#206776,#206777,
#206778,#206779,#206780,#206781,#206782,#206783,#206784,#206785,#206786,
#206787,#206788,#206789,#206790,#206791,#206792,#206793,#206794,#206795,
#206796,#206797,#206798,#206799,#206800,#206801,#206802,#206803,#206804,
#206805,#206806,#206807,#206808,#206809),.UNSPECIFIED.,.F.,.F.,(4,2,2,2,
2,2,2,2,2,2,2,2,2,2,2,2,2,2,2,2,2,2,2,2,2,2,2,2,2,2,2,2,2,2,2,4),(-17.1620566513902,
-17.0701997094641,-16.904359851517,-16.73085642586,-16.4591336747313,-16.3106797711992,
-16.2225325965221,-15.864752733382,-15.5094655368914,-15.350730421272,-15.206575755354,
-15.0564334242206,-14.9671036987014,-14.7913228671624,-14.6434878566294,
-14.4840597819354,-14.3255899820278,-14.2364158793949,-14.0597959539414,
-13.8817212505758,-13.7015961877199,-13.5488101428796,-13.3943208444835,
-13.2307006383988,-13.1420687705111,-12.9628774862974,-12.7987939786307,
-12.6529353983322,-12.4973750820984,-12.3038931681488,-12.1420166067712,
-12.0583227818685,-11.8789515515351,-11.7435506383085,-11.5348041836882,
-11.4417380987961),.UNSPECIFIED.);
#30400=B_SPLINE_CURVE_WITH_KNOTS('',3,(#206810,#206811,#206812,#206813,
#206814,#206815,#206816,#206817,#206818,#206819,#206820,#206821,#206822,
#206823,#206824,#206825,#206826,#206827,#206828,#206829,#206830,#206831,
#206832,#206833,#206834,#206835,#206836,#206837,#206838,#206839,#206840,
#206841,#206842,#206843,#206844,#206845,#206846,#206847,#206848,#206849,
#206850,#206851,#206852,#206853,#206854,#206855,#206856,#206857,#206858,
#206859,#206860,#206861,#206862,#206863,#206864,#206865,#206866,#206867,
#206868,#206869,#206870,#206871,#206872,#206873,#206874,#206875,#206876,
#206877),.UNSPECIFIED.,.F.,.F.,(4,2,2,2,2,2,2,2,2,2,2,2,2,2,2,2,2,2,2,2,
2,2,2,2,2,2,2,2,2,2,2,2,2,4),(-8.58288598458152,-8.46851059617028,-8.31821013384429,
-8.03138467818614,-7.67593192574583,-7.58797629524239,-7.43061142801808,
-7.25095832007405,-7.16241149566316,-7.004909138247,-6.86028525748937,-6.69154418576299,
-6.51323022248577,-6.42445253407658,-6.25733786057316,-6.06457571797289,
-5.90460532302624,-5.74822811543796,-5.59531793438502,-5.41934787698796,
-5.33009193009703,-5.17355970644515,-5.02475475717209,-4.87451797166454,
-4.69873282775091,-4.51879651590067,-4.16262955435834,-3.80463506979839,
-3.7166292175596,-3.56433073312492,-3.29214753994671,-3.11861456496206,
-2.95246910301541,-2.8610678083529),.UNSPECIFIED.);
#30401=B_SPLINE_CURVE_WITH_KNOTS('',3,(#206883,#206884,#206885,#206886),
 .UNSPECIFIED.,.F.,.F.,(4,4),(-9.10624753604124E-6,-1.00000002245526E-6),
 .UNSPECIFIED.);
#30402=B_SPLINE_CURVE_WITH_KNOTS('',3,(#206888,#206889,#206890,#206891,
#206892,#206893,#206894,#206895),.UNSPECIFIED.,.F.,.F.,(4,2,2,4),(0.000264654385573201,
0.197179255479995,0.294830977384857,0.393932741177773),.UNSPECIFIED.);
#30403=B_SPLINE_CURVE_WITH_KNOTS('',3,(#206898,#206899,#206900,#206901,
#206902,#206903,#206904,#206905),.UNSPECIFIED.,.F.,.F.,(4,2,2,4),(-0.393859367021486,
-0.195155499306153,-0.0984062565036703,-0.000187054781717022),
 .UNSPECIFIED.);
#30404=B_SPLINE_CURVE_WITH_KNOTS('',3,(#206908,#206909,#206910,#206911,
#206912,#206913,#206914,#206915,#206916,#206917,#206918,#206919,#206920,
#206921,#206922,#206923,#206924,#206925,#206926,#206927,#206928,#206929,
#206930,#206931,#206932,#206933,#206934,#206935,#206936,#206937,#206938,
#206939,#206940,#206941,#206942,#206943,#206944,#206945,#206946,#206947,
#206948,#206949,#206950,#206951,#206952,#206953,#206954,#206955,#206956,
#206957,#206958,#206959,#206960,#206961,#206962,#206963,#206964,#206965,
#206966,#206967,#206968,#206969,#206970,#206971,#206972,#206973),
 .UNSPECIFIED.,.F.,.F.,(4,2,2,2,2,2,2,2,2,2,2,2,2,2,2,2,2,2,2,2,2,2,2,2,
2,2,2,2,2,2,2,2,4),(-20.0261911591635,-19.7901934295335,-19.5560940283505,
-19.4036395436267,-19.2565931006169,-19.1672547768,-18.9914680343798,-18.8452477477883,
-18.7102619323775,-18.5409811946449,-18.3351165290447,-18.1682508621197,
-17.9965602320071,-17.8266219334632,-17.608983519323,-17.4393211233688,
-17.3507328805447,-17.1721276112691,-17.0229918399559,-16.8616276503751,
-16.7018749905528,-16.531682353722,-16.3612915040967,-16.1877446686152,
-15.8323524409229,-15.5329897781126,-15.4452006269922,-15.1739016223424,
-14.993531276491,-14.813721299713,-14.6606761967681,-14.5726633728389,-14.30529387033),
 .UNSPECIFIED.);
#30405=B_SPLINE_CURVE_WITH_KNOTS('',3,(#206976,#206977,#206978,#206979,
#206980,#206981,#206982,#206983,#206984,#206985,#206986,#206987,#206988,
#206989,#206990,#206991,#206992,#206993,#206994,#206995,#206996,#206997,
#206998,#206999,#207000,#207001,#207002,#207003,#207004,#207005,#207006,
#207007,#207008,#207009,#207010,#207011,#207012,#207013,#207014,#207015,
#207016,#207017,#207018,#207019,#207020,#207021,#207022,#207023,#207024,
#207025,#207026,#207027,#207028,#207029,#207030,#207031,#207032,#207033,
#207034,#207035,#207036,#207037,#207038,#207039),.UNSPECIFIED.,.F.,.F.,
(4,2,2,2,2,2,2,2,2,2,2,2,2,2,2,2,2,2,2,2,2,2,2,2,2,2,2,2,2,2,2,4),(-5.72211617364862,
-5.45144606650527,-5.3633052520705,-5.21572875839572,-4.94204657011516,
-4.7684701239606,-4.60105176610644,-4.41970948295995,-4.27072885820464,
-4.12114797529049,-3.82944484156022,-3.47369830924017,-3.29998251974305,
-3.1295246180773,-2.95909462929261,-2.79532532558971,-2.63619886337304,
-2.48604117540911,-2.17544688801221,-2.08746385928504,-1.93484205763217,
-1.76012459250849,-1.58397517528309,-1.49481489335935,-1.33338753263079,
-1.1490392729983,-1.00494293849868,-0.801857008033588,-0.664088345956647,
-0.335938630733057,-0.252209855432774,-9.10624753604124E-6),
 .UNSPECIFIED.);
#30406=B_SPLINE_CURVE_WITH_KNOTS('',3,(#207044,#207045,#207046,#207047,
#207048,#207049,#207050,#207051,#207052,#207053,#207054,#207055,#207056,
#207057,#207058,#207059,#207060,#207061,#207062,#207063,#207064,#207065,
#207066,#207067,#207068,#207069,#207070,#207071,#207072,#207073,#207074,
#207075,#207076,#207077,#207078,#207079,#207080,#207081,#207082,#207083,
#207084,#207085,#207086,#207087,#207088,#207089,#207090,#207091,#207092,
#207093,#207094,#207095,#207096,#207097,#207098,#207099,#207100,#207101,
#207102,#207103,#207104,#207105),.UNSPECIFIED.,.F.,.F.,(4,2,2,2,2,2,2,2,
2,2,2,2,2,2,2,2,2,2,2,2,2,2,2,2,2,2,2,2,2,2,4),(-11.4453555711932,-11.2868526815436,
-10.9283028098601,-10.5679594860918,-10.3092878491564,-10.1011704626875,
-10.0136956633507,-9.83704715036268,-9.74840954808365,-9.6037178358129,
-9.30695121065821,-8.95089887793476,-8.77626913462526,-8.60529767077106,
-8.43340752041267,-8.26372948570216,-8.14556017964418,-7.97486491658098,
-7.79763042634811,-7.70867088721176,-7.54222343817563,-7.34448119580206,
-7.18264701373627,-7.00152016368675,-6.85719439430696,-6.64009268403691,
-6.50065906693968,-6.32149308911038,-6.16486393792819,-5.80935272002635,
-5.72211617364862),.UNSPECIFIED.);
#30407=B_SPLINE_CURVE_WITH_KNOTS('',3,(#207106,#207107,#207108,#207109,
#207110,#207111,#207112,#207113,#207114,#207115,#207116,#207117,#207118,
#207119,#207120,#207121,#207122,#207123,#207124,#207125,#207126,#207127,
#207128,#207129,#207130,#207131,#207132,#207133,#207134,#207135,#207136,
#207137,#207138,#207139,#207140,#207141,#207142,#207143,#207144,#207145,
#207146,#207147,#207148,#207149,#207150,#207151,#207152,#207153,#207154,
#207155,#207156,#207157,#207158,#207159,#207160,#207161,#207162,#207163,
#207164,#207165,#207166,#207167),.UNSPECIFIED.,.F.,.F.,(4,2,2,2,2,2,2,2,
2,2,2,2,2,2,2,2,2,2,2,2,2,2,2,2,2,2,2,2,2,2,4),(-14.30529387033,-14.214635198436,
-13.8584617770324,-13.6785499880908,-13.5027518196477,-13.3546092672862,
-13.2001155595787,-13.0453669138218,-12.956086461402,-12.7800997287169,
-12.6232959758484,-12.4961681013161,-12.3267364071978,-12.1226954065264,
-11.9540253642301,-11.7562548269082,-11.5881848396705,-11.4172301653806,
-11.2466872819809,-11.0725892239989,-10.7163691877442,-10.436500748924,
-10.2781001697233,-10.1895252680676,-10.0128939376982,-9.92540538050117,
-9.7221803864745,-9.46331745376698,-9.10309646813805,-8.74493137208567,
-8.5824306122609),.UNSPECIFIED.);
#30408=B_SPLINE_CURVE_WITH_KNOTS('',3,(#207172,#207173,#207174,#207175,
#207176,#207177,#207178,#207179,#207180,#207181,#207182,#207183,#207184,
#207185,#207186,#207187,#207188,#207189,#207190,#207191,#207192,#207193,
#207194,#207195,#207196,#207197,#207198,#207199,#207200,#207201,#207202,
#207203,#207204,#207205,#207206,#207207,#207208,#207209,#207210,#207211,
#207212,#207213,#207214,#207215,#207216,#207217,#207218,#207219,#207220,
#207221,#207222,#207223,#207224,#207225,#207226,#207227,#207228,#207229,
#207230,#207231,#207232,#207233,#207234,#207235,#207236,#207237,#207238,
#207239,#207240,#207241,#207242,#207243,#207244,#207245),.UNSPECIFIED.,
 .F.,.F.,(4,2,2,2,2,2,2,2,2,2,2,2,2,2,2,2,2,2,2,2,2,2,2,2,2,2,2,2,2,2,2,
2,2,2,2,2,4),(-17.166235588483,-17.1290620281814,-16.8564247638492,-16.7081866111978,
-16.6200472505132,-16.262216084275,-15.9068054388724,-15.7503880717279,
-15.6001841980369,-15.4518261553452,-15.3624610849156,-15.1866414162631,
-15.0348927644298,-14.8800867026375,-14.7224140652765,-14.6332233584554,
-14.4565822398736,-14.2784347564555,-14.0983608695542,-13.944597984781,
-13.7912875839889,-13.6280294912066,-13.5393862977335,-13.3601858785979,
-13.2005980542115,-13.0781456483354,-12.9084210492395,-12.823102902181,
-12.735600182679,-12.5645357834063,-12.3901511907983,-12.1044488364628,
-11.9461820660416,-11.8015524326663,-11.6310593138553,-11.4613677768082,
-11.4453555711932),.UNSPECIFIED.);
#30409=B_SPLINE_CURVE_WITH_KNOTS('',3,(#207246,#207247,#207248,#207249,
#207250,#207251,#207252,#207253,#207254,#207255,#207256,#207257,#207258,
#207259,#207260,#207261,#207262,#207263,#207264,#207265,#207266,#207267,
#207268,#207269,#207270,#207271,#207272,#207273,#207274,#207275,#207276,
#207277,#207278,#207279,#207280,#207281,#207282,#207283,#207284,#207285,
#207286,#207287,#207288,#207289,#207290,#207291,#207292,#207293,#207294,
#207295,#207296,#207297,#207298,#207299,#207300,#207301,#207302,#207303,
#207304,#207305,#207306,#207307,#207308,#207309,#207310,#207311,#207312,
#207313),.UNSPECIFIED.,.F.,.F.,(4,2,2,2,2,2,2,2,2,2,2,2,2,2,2,2,2,2,2,2,
2,2,2,2,2,2,2,2,2,2,2,2,2,4),(-8.5824306122609,-8.57103770819693,-8.40325571514215,
-8.23587731607054,-8.09807718898508,-7.87804323785844,-7.74008814103692,
-7.55930879121377,-7.26215386073682,-6.906151748955,-6.73157115865593,-6.56061385975624,
-6.38879209803198,-6.21911161776177,-5.99012880275868,-5.90238817036819,
-5.71544395322699,-5.56262175016414,-5.3827312589457,-5.29369993625239,
-5.12458390792792,-5.00403736786862,-4.84033276501113,-4.6645241502789,
-4.57516300392967,-4.42711804071362,-4.27509016740412,-4.1199929652534,
-3.7645535559046,-3.40672055774514,-3.3185896395958,-3.17024067651289,-2.89755199278977,
-2.8604020772222),.UNSPECIFIED.);
#30410=B_SPLINE_CURVE_WITH_KNOTS('',3,(#207319,#207320,#207321,#207322),
 .UNSPECIFIED.,.F.,.F.,(4,4),(0.000166910408725463,0.000172246164436567),
 .UNSPECIFIED.);
#30411=B_SPLINE_CURVE_WITH_KNOTS('',3,(#207324,#207325,#207326,#207327,
#207328,#207329),.UNSPECIFIED.,.F.,.F.,(4,2,4),(0.000158868425727158,0.234718202342811,
0.469154050604624),.UNSPECIFIED.);
#30412=B_SPLINE_CURVE_WITH_KNOTS('',3,(#207336,#207337,#207338,#207339,
#207340,#207341,#207342,#207343,#207344,#207345,#207346,#207347,#207348,
#207349,#207350,#207351,#207352,#207353,#207354,#207355,#207356,#207357,
#207358,#207359,#207360,#207361,#207362,#207363,#207364,#207365,#207366,
#207367,#207368,#207369,#207370,#207371,#207372,#207373,#207374,#207375,
#207376,#207377,#207378,#207379,#207380,#207381,#207382,#207383,#207384,
#207385,#207386,#207387,#207388,#207389,#207390,#207391,#207392,#207393,
#207394,#207395,#207396,#207397,#207398,#207399,#207400,#207401,#207402,
#207403,#207404,#207405,#207406,#207407,#207408,#207409),.UNSPECIFIED.,
 .F.,.F.,(4,2,2,2,2,2,2,2,2,2,2,2,2,2,2,2,2,2,2,2,2,2,2,2,2,2,2,2,2,2,2,
2,2,2,2,2,4),(-6.99961622965257,-6.96391578728215,-6.73460522677822,-6.49987907509467,
-6.27549114934176,-6.16171354295781,-5.9319207685918,-5.69736222847282,
-5.47298362661363,-5.35906532128113,-5.1290559345853,-4.89456581019745,
-4.67025576664923,-4.55618747183648,-4.32637094188848,-4.09174449679306,
-3.8675865506281,-3.75343209190301,-3.52419107187844,-3.25370641558361,
-3.13975920840176,-2.95251199520079,-2.72382611475827,-2.44530613821909,
-2.33128288872491,-2.00859486011215,-1.89364040439153,-1.73174264476915,
-1.50515816911957,-1.24787775884641,-1.13380587579145,-0.958202539565173,
-0.729140507942947,-0.494185151112094,-0.250153069066657,-0.125295117691977,
-0.000535240498741617),.UNSPECIFIED.);
#30413=B_SPLINE_CURVE_WITH_KNOTS('',3,(#207412,#207413,#207414,#207415,
#207416,#207417,#207418,#207419,#207420,#207421,#207422,#207423,#207424,
#207425,#207426,#207427,#207428,#207429,#207430,#207431,#207432,#207433,
#207434,#207435,#207436,#207437,#207438,#207439,#207440,#207441,#207442,
#207443,#207444,#207445,#207446,#207447,#207448,#207449,#207450,#207451,
#207452,#207453,#207454,#207455,#207456,#207457,#207458,#207459,#207460,
#207461,#207462,#207463,#207464,#207465,#207466,#207467,#207468,#207469,
#207470,#207471,#207472,#207473,#207474,#207475,#207476,#207477,#207478,
#207479,#207480,#207481,#207482,#207483),.UNSPECIFIED.,.F.,.F.,(4,2,2,2,
2,2,2,2,2,2,2,2,2,2,2,2,2,2,2,2,2,2,2,2,2,2,2,2,2,2,2,2,2,2,2,4),(-24.6761488606007,
-24.5536439797374,-24.4309909429808,-24.1916221027102,-23.9565240762551,
-23.7281632573065,-23.6142884178381,-23.390153971156,-23.1549002339024,
-23.0406665683764,-22.7725487102365,-22.6579276896609,-22.4304762591835,
-22.2063853627223,-21.9629289515731,-21.7352875834566,-21.5770834181909,
-21.4624147721794,-21.2334477924476,-21.0093471006007,-20.7550531474735,
-20.525866361529,-20.3726134692837,-20.2580599272056,-19.938146030468,-19.7071268961134,
-19.4776001634708,-19.1298823887128,-19.0156965246622,-18.7922790652087,
-18.567360532056,-18.3326914807233,-18.2184489417264,-17.9944926139954,
-17.7699051708102,-17.6762610095338),.UNSPECIFIED.);
#30414=B_SPLINE_CURVE_WITH_KNOTS('',3,(#207488,#207489,#207490,#207491,
#207492,#207493,#207494,#207495,#207496,#207497,#207498,#207499,#207500,
#207501,#207502,#207503,#207504,#207505,#207506,#207507,#207508,#207509,
#207510,#207511,#207512,#207513,#207514,#207515,#207516,#207517,#207518,
#207519,#207520,#207521,#207522,#207523,#207524,#207525,#207526,#207527,
#207528,#207529,#207530,#207531,#207532,#207533,#207534,#207535,#207536,
#207537,#207538,#207539,#207540,#207541,#207542,#207543,#207544,#207545,
#207546,#207547,#207548,#207549,#207550,#207551,#207552,#207553,#207554,
#207555,#207556,#207557,#207558,#207559,#207560,#207561,#207562,#207563),
 .UNSPECIFIED.,.F.,.F.,(4,2,2,2,2,2,2,2,2,2,2,2,2,2,2,2,2,2,2,2,2,2,2,2,
2,2,2,2,2,2,2,2,2,2,2,2,2,4),(-14.4468995549683,-14.3338230138911,-14.1049853155161,
-13.9911346407241,-13.7668625729503,-13.5317910990408,-13.3034542451472,
-13.1121055062976,-12.9980663688873,-12.7755786428509,-12.5511637402028,
-12.3376524508539,-12.1169631347962,-11.89244615783,-11.7786512059243,-11.5484712642546,
-11.2576695020677,-11.1435363437395,-10.8691017091229,-10.7551201682166,
-10.4083152994627,-10.1772149624584,-9.94805105254814,-9.63178517014678,
-9.51704203555597,-9.36866156248235,-9.14039244722859,-8.9051388454019,
-8.68103340781509,-8.56718342498947,-8.33883211661612,-8.10371161990445,
-7.87945222661585,-7.76569166175392,-7.53692932536058,-7.30199255339616,
-7.07763708918854,-6.99961622965257),.UNSPECIFIED.);
#30415=B_SPLINE_CURVE_WITH_KNOTS('',3,(#207564,#207565,#207566,#207567,
#207568,#207569,#207570,#207571,#207572,#207573,#207574,#207575,#207576,
#207577,#207578,#207579,#207580,#207581,#207582,#207583,#207584,#207585,
#207586,#207587,#207588,#207589,#207590,#207591,#207592,#207593,#207594,
#207595,#207596,#207597,#207598,#207599,#207600,#207601,#207602,#207603,
#207604,#207605,#207606,#207607,#207608,#207609,#207610,#207611,#207612,
#207613,#207614,#207615,#207616,#207617,#207618,#207619,#207620,#207621,
#207622,#207623,#207624,#207625,#207626,#207627,#207628,#207629,#207630,
#207631,#207632,#207633,#207634,#207635,#207636,#207637,#207638,#207639,
#207640,#207641),.UNSPECIFIED.,.F.,.F.,(4,2,2,2,2,2,2,2,2,2,2,2,2,2,2,2,
2,2,2,2,2,2,2,2,2,2,2,2,2,2,2,2,2,2,2,2,2,2,4),(-17.6762610095338,-17.5419908579114,
-17.3131157857729,-17.1992573974253,-16.9749636654749,-16.7398785388768,
-16.5115085298758,-16.3975830001727,-16.1734076813033,-15.9381503008392,
-15.7100545893463,-15.5960347950023,-15.3720110876936,-15.1366797103947,
-14.9084672287798,-14.7578872231388,-14.6431928204129,-14.414883927883,
-14.1907508768027,-13.9437496450835,-13.8294506512664,-13.5267457198042,
-13.412662900829,-13.1289422646053,-12.898879177942,-12.7849725900379,-12.5605070969637,
-12.3388849321193,-12.1230679108322,-11.8986867387086,-11.6758968209308,
-11.5618217668304,-11.3774685411443,-11.1487011126834,-10.9136767675669,
-10.6892651770141,-10.4651893114796,-10.3509213635975,-10.2287171917464),
 .UNSPECIFIED.);
#30416=B_SPLINE_CURVE_WITH_KNOTS('',3,(#207646,#207647,#207648,#207649,
#207650,#207651,#207652,#207653,#207654,#207655,#207656,#207657,#207658,
#207659,#207660,#207661,#207662,#207663,#207664,#207665,#207666,#207667,
#207668,#207669,#207670,#207671,#207672,#207673,#207674,#207675,#207676,
#207677,#207678,#207679,#207680,#207681,#207682,#207683,#207684,#207685,
#207686,#207687,#207688,#207689,#207690,#207691,#207692,#207693,#207694,
#207695,#207696,#207697,#207698,#207699,#207700,#207701,#207702,#207703,
#207704,#207705,#207706,#207707,#207708,#207709,#207710,#207711,#207712,
#207713,#207714,#207715,#207716,#207717,#207718,#207719,#207720,#207721),
 .UNSPECIFIED.,.F.,.F.,(4,2,2,2,2,2,2,2,2,2,2,2,2,2,2,2,2,2,2,2,2,2,2,2,
2,2,2,2,2,2,2,2,2,2,2,2,2,4),(-21.8941006277626,-21.780740412087,-21.545887927874,
-21.4315987982601,-21.1966662763011,-20.9720787002586,-20.7868693665202,
-20.5619196383158,-20.3833365915359,-20.2680385408366,-19.9362331764476,
-19.8221772895811,-19.5618881397594,-19.3352647253081,-19.1728063081744,
-19.0579504591606,-18.8293134558212,-18.6050181008145,-18.348427763471,
-18.1198963356815,-18.0055357561925,-17.7815590670609,-17.5793331813053,
-17.3442776335965,-17.1710180856163,-17.0563086033263,-16.7283892268032,
-16.4972731113214,-16.2678539132103,-15.9217722116351,-15.8075940171985,
-15.5841696373609,-15.3592839501101,-15.1246300414118,-15.0103952794729,
-14.7864374327893,-14.5618787393385,-14.4468995549683),.UNSPECIFIED.);
#30417=B_SPLINE_CURVE_WITH_KNOTS('',3,(#207722,#207723,#207724,#207725,
#207726,#207727,#207728,#207729,#207730,#207731,#207732,#207733,#207734,
#207735,#207736,#207737,#207738,#207739,#207740,#207741,#207742,#207743,
#207744,#207745,#207746,#207747,#207748,#207749,#207750,#207751,#207752,
#207753,#207754,#207755,#207756,#207757,#207758,#207759,#207760,#207761,
#207762,#207763,#207764,#207765,#207766,#207767,#207768,#207769,#207770,
#207771,#207772,#207773,#207774,#207775,#207776,#207777,#207778,#207779,
#207780,#207781,#207782,#207783,#207784,#207785,#207786,#207787,#207788,
#207789,#207790,#207791,#207792,#207793,#207794,#207795,#207796,#207797,
#207798,#207799),.UNSPECIFIED.,.F.,.F.,(4,2,2,2,2,2,2,2,2,2,2,2,2,2,2,2,
2,2,2,2,2,2,2,2,2,2,2,2,2,2,2,2,2,2,2,2,2,2,4),(-10.2287171917464,-10.1161007911178,
-9.89141055980067,-9.6678705935114,-9.55364216626409,-9.23717401805758,
-9.12262327489105,-8.88796410295785,-8.66393856533794,-8.5491156077035,
-8.3209369932818,-8.0592223034357,-7.94507330386266,-7.62969963912177,-7.51523207325705,
-7.23314021509567,-7.11877209325123,-6.85536329826687,-6.74132701173776,
-6.41901820793362,-6.30428383308501,-6.13938890573675,-5.90463023907916,
-5.74450993837472,-5.51737633472601,-5.26681979415362,-5.04220502816595,
-4.81376837806515,-4.69871024394659,-4.53568257856599,-4.30924644403034,
-4.04662489230807,-3.9323967044129,-3.69737473426783,-3.47297320997549,
-3.24926425480023,-3.13503985545589,-2.90021146096247,-2.78095249520184),
 .UNSPECIFIED.);
#30418=B_SPLINE_CURVE_WITH_KNOTS('',3,(#207805,#207806,#207807,#207808),
 .UNSPECIFIED.,.F.,.F.,(4,4),(-2.9809807408467E-6,-9.99999997800541E-7),
 .UNSPECIFIED.);
#30419=B_SPLINE_CURVE_WITH_KNOTS('',3,(#207810,#207811,#207812,#207813,
#207814,#207815,#207816,#207817,#207818,#207819,#207820,#207821,#207822,
#207823,#207824,#207825,#207826,#207827,#207828,#207829,#207830,#207831,
#207832,#207833),.UNSPECIFIED.,.F.,.F.,(4,2,2,2,2,2,2,2,2,2,2,4),(-1.88511749360749,
-1.67932546370318,-1.47452695473615,-1.33807794357269,-1.10356671114348,
-0.989276200715796,-0.873916730130468,-0.661501517586868,-0.498025260970523,
-0.252000037949951,-0.126229715468468,-0.0002548003213796),
 .UNSPECIFIED.);
#30420=B_SPLINE_CURVE_WITH_KNOTS('',3,(#207836,#207837,#207838,#207839,
#207840,#207841,#207842,#207843,#207844,#207845,#207846,#207847,#207848,
#207849,#207850,#207851,#207852,#207853,#207854,#207855,#207856,#207857),
 .UNSPECIFIED.,.F.,.F.,(4,2,2,2,2,2,2,2,2,2,4),(5.98718350647653E-5,0.203932709927811,
0.406516261468775,0.541488095383762,0.718522052217883,0.942619519328388,
1.17051888563054,1.39440958810362,1.63674335451152,1.76079483716854,1.88502497314767),
 .UNSPECIFIED.);
#30421=B_SPLINE_CURVE_WITH_KNOTS('',3,(#207860,#207861,#207862,#207863,
#207864,#207865,#207866,#207867,#207868,#207869,#207870,#207871,#207872,
#207873,#207874,#207875,#207876,#207877,#207878,#207879,#207880,#207881,
#207882,#207883,#207884,#207885,#207886,#207887,#207888,#207889,#207890,
#207891,#207892,#207893,#207894,#207895,#207896,#207897,#207898,#207899,
#207900,#207901,#207902,#207903,#207904,#207905,#207906,#207907,#207908,
#207909,#207910,#207911,#207912,#207913,#207914,#207915,#207916,#207917,
#207918,#207919,#207920,#207921,#207922,#207923,#207924,#207925,#207926,
#207927,#207928,#207929,#207930,#207931,#207932,#207933,#207934,#207935),
 .UNSPECIFIED.,.F.,.F.,(4,2,2,2,2,2,2,2,2,2,2,2,2,2,2,2,2,2,2,2,2,2,2,2,
2,2,2,2,2,2,2,2,2,2,2,2,2,4),(-22.7898778497251,-22.5769609640614,-22.3695124452767,
-22.2312330244057,-21.9516446289458,-21.7229229900236,-21.5359972853678,
-21.4220437741558,-21.1514317382949,-20.9221716042284,-20.808009654741,
-20.5838347309842,-20.3491911828098,-20.1193525791475,-20.0052765391877,
-19.7809474046369,-19.5464387603694,-19.3164055772272,-19.2024801658494,
-18.9780819391374,-18.7435052159597,-18.5136887949594,-18.3999053854775,
-18.1754991758094,-17.9407566335972,-17.7114241829266,-17.5976984882579,
-17.3733273241935,-17.1399839200798,-16.9113426684198,-16.7974862500793,
-16.5732417254602,-16.3380788243774,-16.1098509568817,-15.9959077981696,
-15.7718116070002,-15.5365143255446,-15.3427013025877),.UNSPECIFIED.);
#30422=B_SPLINE_CURVE_WITH_KNOTS('',3,(#207938,#207939,#207940,#207941,
#207942,#207943,#207944,#207945,#207946,#207947,#207948,#207949,#207950,
#207951,#207952,#207953,#207954,#207955,#207956,#207957,#207958,#207959,
#207960,#207961,#207962,#207963,#207964,#207965,#207966,#207967,#207968,
#207969,#207970,#207971,#207972,#207973,#207974,#207975,#207976,#207977,
#207978,#207979,#207980,#207981,#207982,#207983,#207984,#207985,#207986,
#207987,#207988,#207989,#207990,#207991,#207992,#207993,#207994,#207995,
#207996,#207997,#207998,#207999,#208000,#208001,#208002,#208003,#208004,
#208005,#208006,#208007,#208008,#208009,#208010,#208011,#208012,#208013,
#208014,#208015),.UNSPECIFIED.,.F.,.F.,(4,2,2,2,2,2,2,2,2,2,2,2,2,2,2,2,
2,2,2,2,2,2,2,2,2,2,2,2,2,2,2,2,2,2,2,2,2,2,4),(-7.44716700303765,-7.38821906924776,
-7.27428145715534,-7.06688827855258,-6.83996772069574,-6.62191392601838,
-6.39766012445358,-6.17371232000397,-6.05949518821232,-5.8245461642506,
-5.60000112988346,-5.37668289458153,-5.26247364391113,-5.02769031769412,
-4.80274782323196,-4.56791504903113,-4.45364256518003,-4.21899719582635,
-3.99432645102175,-3.7701326911471,-3.65593332336233,-3.33757632247385,
-3.22304872331591,-2.94112313631895,-2.8267168206034,-2.56242098741452,
-2.44830716819401,-2.14282098982722,-2.02851425171739,-1.77636422371573,
-1.66241821220455,-1.44250391547649,-1.20765092501976,-1.03094059547456,
-0.796125839660265,-0.602228919090577,-0.45287392841626,-0.226871301920059,
-2.9809807408467E-6),.UNSPECIFIED.);
#30423=B_SPLINE_CURVE_WITH_KNOTS('',3,(#208020,#208021,#208022,#208023,
#208024,#208025,#208026,#208027,#208028,#208029,#208030,#208031,#208032,
#208033,#208034,#208035,#208036,#208037,#208038,#208039,#208040,#208041,
#208042,#208043,#208044,#208045,#208046,#208047,#208048,#208049,#208050,
#208051,#208052,#208053,#208054,#208055,#208056,#208057,#208058,#208059,
#208060,#208061,#208062,#208063,#208064,#208065,#208066,#208067,#208068,
#208069,#208070,#208071,#208072,#208073,#208074,#208075,#208076,#208077,
#208078,#208079,#208080,#208081,#208082,#208083,#208084,#208085,#208086,
#208087,#208088,#208089,#208090,#208091,#208092,#208093,#208094,#208095,
#208096,#208097),.UNSPECIFIED.,.F.,.F.,(4,2,2,2,2,2,2,2,2,2,2,2,2,2,2,2,
2,2,2,2,2,2,2,2,2,2,2,2,2,2,2,2,2,2,2,2,2,2,4),(-14.8946700477258,-14.8517362223534,
-14.6214125150804,-14.4352051146492,-14.3210509902728,-14.0979141027459,
-13.8728253741749,-13.638230718361,-13.5240136865351,-13.3002647009627,
-13.0755452699733,-12.8408118139435,-12.7265409496863,-12.4916521557968,
-12.2667033382962,-12.0523755399774,-11.8242444978479,-11.6248243519107,
-11.3949567393001,-11.2807671494687,-11.1004347878287,-10.8697045571671,
-10.635190741098,-10.4104612772714,-10.1861089283667,-10.0719981856532,
-9.73942527197504,-9.62457831078745,-9.43460635965954,-9.19962189879514,
-9.0854757521845,-8.85637593762672,-8.5832741345898,-8.4693089289279,-8.28989617589463,
-8.06088048439594,-7.75546279704184,-7.64098328995621,-7.44716700303765),
 .UNSPECIFIED.);
#30424=B_SPLINE_CURVE_WITH_KNOTS('',3,(#208098,#208099,#208100,#208101,
#208102,#208103,#208104,#208105,#208106,#208107,#208108,#208109,#208110,
#208111,#208112,#208113,#208114,#208115,#208116,#208117,#208118,#208119,
#208120,#208121,#208122,#208123,#208124,#208125,#208126,#208127,#208128,
#208129,#208130,#208131,#208132,#208133,#208134,#208135,#208136,#208137,
#208138,#208139,#208140,#208141,#208142,#208143,#208144,#208145,#208146,
#208147,#208148,#208149,#208150,#208151,#208152,#208153,#208154,#208155,
#208156,#208157,#208158,#208159,#208160,#208161,#208162,#208163,#208164,
#208165,#208166,#208167,#208168,#208169,#208170,#208171,#208172,#208173,
#208174,#208175,#208176,#208177),.UNSPECIFIED.,.F.,.F.,(4,2,2,2,2,2,2,2,
2,2,2,2,2,2,2,2,2,2,2,2,2,2,2,2,2,2,2,2,2,2,2,2,2,2,2,2,2,2,2,4),(-15.3427013025877,
-15.308377083126,-15.1198299572003,-15.0058773390422,-14.7827804020896,
-14.5479713358685,-14.3128246478954,-14.1989229240919,-13.936125651035,
-13.7072754352123,-13.5929916628281,-13.3689291282708,-13.1682327373279,
-13.0533139372504,-12.7176624551363,-12.6035535375263,-12.3792784911725,
-12.1545198581629,-11.9200025711672,-11.6892296049746,-11.509552355854,
-11.3953619097248,-11.1654843733141,-10.9653174025646,-10.7372355087874,
-10.5246262139959,-10.2996083571961,-10.1000341502175,-9.87582954799773,
-9.76159792532465,-9.53286039336265,-9.30541050113956,-9.08104214635054,
-8.96713906917654,-8.73727439389497,-8.50274606740872,-8.27841007432963,
-8.16435618488069,-7.93445330201098,-7.89546626363725),.UNSPECIFIED.);
#30425=B_SPLINE_CURVE_WITH_KNOTS('',3,(#208182,#208183,#208184,#208185,
#208186,#208187,#208188,#208189,#208190,#208191,#208192,#208193,#208194,
#208195,#208196,#208197,#208198,#208199,#208200,#208201,#208202,#208203,
#208204,#208205,#208206,#208207,#208208,#208209,#208210,#208211,#208212,
#208213,#208214,#208215,#208216,#208217,#208218,#208219,#208220,#208221,
#208222,#208223,#208224,#208225,#208226,#208227,#208228,#208229,#208230,
#208231,#208232,#208233,#208234,#208235,#208236,#208237,#208238,#208239,
#208240,#208241,#208242,#208243,#208244,#208245,#208246,#208247,#208248,
#208249,#208250,#208251,#208252,#208253,#208254,#208255,#208256,#208257),
 .UNSPECIFIED.,.F.,.F.,(4,2,2,2,2,2,2,2,2,2,2,2,2,2,2,2,2,2,2,2,2,2,2,2,
2,2,2,2,2,2,2,2,2,2,2,2,2,4),(-22.342212772346,-22.0873250974015,-21.8590935717735,
-21.7442773051237,-21.5202809959495,-21.2856618803179,-21.0576420432068,
-20.8981008541047,-20.6717097349625,-20.5014524842998,-20.3863957461922,
-20.05201737793,-19.9378145342768,-19.7146260410002,-19.4900223022936,-19.2551146528616,
-19.1409019380648,-18.9170712445363,-18.6927764342657,-18.4576614111678,
-18.2290862188997,-18.0472275704511,-17.9332151496194,-17.7100946558276,
-17.4858717510111,-17.2679229347136,-17.1536153204947,-16.8551315088828,
-16.7410621886897,-16.4741067334556,-16.3596892939691,-16.0508381737592,
-15.9367797235592,-15.654535714996,-15.4246277315006,-15.310679005235,-15.0862764825703,
-14.8946700477258),.UNSPECIFIED.);
#30426=B_SPLINE_CURVE_WITH_KNOTS('',3,(#208258,#208259,#208260,#208261,
#208262,#208263,#208264,#208265,#208266,#208267,#208268,#208269,#208270,
#208271,#208272,#208273,#208274,#208275,#208276,#208277,#208278,#208279,
#208280,#208281,#208282,#208283,#208284,#208285,#208286,#208287,#208288,
#208289,#208290,#208291,#208292,#208293,#208294,#208295,#208296,#208297,
#208298,#208299,#208300,#208301,#208302,#208303,#208304,#208305,#208306,
#208307,#208308,#208309,#208310,#208311,#208312,#208313,#208314,#208315,
#208316,#208317,#208318,#208319,#208320,#208321,#208322,#208323,#208324,
#208325,#208326,#208327,#208328,#208329,#208330,#208331,#208332,#208333,
#208334,#208335),.UNSPECIFIED.,.F.,.F.,(4,2,2,2,2,2,2,2,2,2,2,2,2,2,2,2,
2,2,2,2,2,2,2,2,2,2,2,2,2,2,2,2,2,2,2,2,2,2,4),(-7.89546626363725,-7.69990956786955,
-7.47567575446496,-7.3615016075955,-7.13198331357449,-6.86609849690881,
-6.75212893118196,-6.54990280206718,-6.32194913420725,-6.07666857325898,
-5.8525875973681,-5.6246458581589,-5.51001025855811,-5.22814394054347,-5.11358386940624,
-4.8533923353295,-4.73932613652158,-4.40650160285151,-4.29116066157497,
-4.10963949560704,-3.88487417100665,-3.68607608359745,-3.46186854734996,
-3.34774564045541,-3.1194968319031,-2.90576828195544,-2.68074515135746,
-2.44588963266135,-2.33163405919186,-2.0969520638675,-1.87218683011271,
-1.64853553127989,-1.53433709317659,-1.20205134984514,-1.08724650032732,
-0.913804339188073,-0.687370374613069,-0.51437072350683,-0.448073224698156),
 .UNSPECIFIED.);
#30427=B_SPLINE_CURVE_WITH_KNOTS('',3,(#208343,#208344,#208345,#208346),
 .UNSPECIFIED.,.F.,.F.,(4,4),(0.,0.000776497202964865),.UNSPECIFIED.);
#30428=B_SPLINE_CURVE_WITH_KNOTS('',3,(#208348,#208349,#208350,#208351,
#208352,#208353,#208354,#208355,#208356,#208357,#208358,#208359,#208360,
#208361,#208362,#208363,#208364,#208365,#208366,#208367,#208368,#208369,
#208370,#208371,#208372,#208373,#208374,#208375,#208376,#208377),
 .UNSPECIFIED.,.F.,.F.,(4,2,2,2,2,2,2,2,2,2,2,2,2,2,4),(-2.58819132413446,
-2.36273572464036,-2.13741551586263,-1.98563553180927,-1.79408322231075,
-1.60046605723319,-1.40804760753452,-1.31130466449971,-1.11849752052555,
-0.921488213499352,-0.727078362402644,-0.545763875761525,-0.273849840655809,
-0.136429802224172,-1.19577251067637E-5),.UNSPECIFIED.);
#30429=B_SPLINE_CURVE_WITH_KNOTS('',3,(#208379,#208380,#208381,#208382,
#208383,#208384,#208385,#208386,#208387,#208388,#208389,#208390,#208391,
#208392,#208393,#208394,#208395,#208396,#208397,#208398,#208399,#208400,
#208401,#208402,#208403,#208404,#208405,#208406,#208407,#208408,#208409,
#208410,#208411,#208412),.UNSPECIFIED.,.F.,.F.,(4,2,2,2,2,2,2,2,2,2,2,2,
2,2,2,2,4),(-2.54573725987018,-2.37476608201991,-2.20211346082218,-2.08770172421983,
-1.93349297075943,-1.75019087472518,-1.56693226938438,-1.47443768915391,
-1.29039242591634,-1.19762811175987,-1.0130459107736,-0.825229741583941,
-0.638712708813757,-0.479166346939911,-0.240379360899738,-0.119773973838457,
-2.99430650133206E-6),.UNSPECIFIED.);
#30430=B_SPLINE_CURVE_WITH_KNOTS('',3,(#208415,#208416,#208417,#208418,
#208419,#208420,#208421,#208422,#208423,#208424,#208425,#208426,#208427,
#208428,#208429,#208430,#208431,#208432,#208433,#208434,#208435,#208436,
#208437,#208438,#208439,#208440,#208441,#208442,#208443,#208444,#208445,
#208446,#208447,#208448,#208449,#208450,#208451),.UNSPECIFIED.,.F.,.F.,
(4,3,3,3,3,3,3,3,3,3,3,3,4),(0.,0.0940528831804072,0.188071722346433,0.282046558286573,
0.375986938965022,0.469884151166603,0.5,0.59354846011734,0.686978341974529,
0.780242306989359,0.873402721161719,0.966421835499807,0.999999946312435),
 .UNSPECIFIED.);
#30431=B_SPLINE_CURVE_WITH_KNOTS('',3,(#208454,#208455,#208456,#208457,
#208458,#208459,#208460,#208461,#208462,#208463,#208464,#208465),
 .UNSPECIFIED.,.F.,.F.,(4,2,2,2,2,4),(1.4160226947081E-5,0.103268302452664,
0.209393167484997,0.42464682943301,0.531127353777131,0.94850884172664),
 .UNSPECIFIED.);
#30432=B_SPLINE_CURVE_WITH_KNOTS('',3,(#208474,#208475,#208476,#208477,
#208478,#208479,#208480,#208481),.UNSPECIFIED.,.F.,.F.,(4,2,2,4),(-0.448073224698156,
-0.259160404724375,-0.130320776825101,-0.000536776125191383),
 .UNSPECIFIED.);
#30433=B_SPLINE_CURVE_WITH_KNOTS('',3,(#208482,#208483,#208484,#208485,
#208486,#208487,#208488,#208489),.UNSPECIFIED.,.F.,.F.,(4,2,2,4),(-22.7900378045853,
-22.4589932577425,-22.3488734903167,-22.342212772346),.UNSPECIFIED.);
#30434=B_SPLINE_CURVE_WITH_KNOTS('',3,(#208492,#208493,#208494,#208495,
#208496,#208497,#208498,#208499,#208500,#208501,#208502,#208503,#208504,
#208505,#208506,#208507,#208508,#208509,#208510,#208511,#208512,#208513,
#208514,#208515,#208516,#208517,#208518,#208519,#208520,#208521,#208522,
#208523),.UNSPECIFIED.,.F.,.F.,(4,2,2,2,2,2,2,2,2,2,2,2,2,2,2,4),(-2.78095249520184,
-2.67548166760889,-2.4524117649796,-2.33820932010235,-1.99663964164419,
-1.88152145310964,-1.68782733522852,-1.46342179217326,-1.34957851491786,
-1.1195579922506,-0.885063164301947,-0.66070119563241,-0.497943683992526,
-0.25136918885441,-0.126361115412786,-0.000333910245350815),
 .UNSPECIFIED.);
#30435=B_SPLINE_CURVE_WITH_KNOTS('',3,(#208526,#208527,#208528,#208529,
#208530,#208531,#208532,#208533,#208534,#208535,#208536,#208537,#208538,
#208539,#208540,#208541,#208542,#208543,#208544,#208545,#208546,#208547,
#208548,#208549,#208550,#208551,#208552,#208553,#208554,#208555,#208556,
#208557),.UNSPECIFIED.,.F.,.F.,(4,2,2,2,2,2,2,2,2,2,2,2,2,2,2,4),(-24.6744529274319,
-24.5441174497078,-24.4149402545385,-24.1589241813401,-23.9872705046797,
-23.7608090756699,-23.5877304959073,-23.4729377236922,-23.1408069622114,
-23.0266185261872,-22.8029811384122,-22.5782347091128,-22.3435721538024,
-22.229327493513,-22.0051981112948,-21.8941006277626),.UNSPECIFIED.);
#30436=B_SPLINE_CURVE_WITH_KNOTS('',3,(#208561,#208562,#208563,#208564,
#208565,#208566,#208567,#208568,#208569,#208570,#208571),.UNSPECIFIED.,
 .F.,.F.,(4,2,3,2,4),(-0.707920522022904,-0.389439958817395,0.,0.389439958817396,
0.707920522023273),.UNSPECIFIED.);
#30437=B_SPLINE_CURVE_WITH_KNOTS('',3,(#208575,#208576,#208577,#208578,
#208579,#208580,#208581,#208582,#208583,#208584,#208585),.UNSPECIFIED.,
 .F.,.F.,(4,2,3,2,4),(-0.704027076636135,-0.390169294707907,0.,0.390169294707907,
0.573011129927055),.UNSPECIFIED.);
#30438=B_SPLINE_CURVE_WITH_KNOTS('',3,(#208587,#208588,#208589,#208590),
 .UNSPECIFIED.,.F.,.F.,(4,4),(0.573011129927055,0.704038599815001),
 .UNSPECIFIED.);
#30439=B_SPLINE_CURVE_WITH_KNOTS('',3,(#208596,#208597,#208598,#208599,
#208600,#208601,#208602,#208603,#208604,#208605,#208606,#208607,#208608,
#208609,#208610,#208611,#208612,#208613,#208614,#208615,#208616,#208617,
#208618,#208619,#208620,#208621,#208622,#208623,#208624,#208625,#208626,
#208627,#208628,#208629,#208630,#208631),.UNSPECIFIED.,.F.,.F.,(4,2,2,2,
2,2,2,2,2,2,2,2,2,2,2,2,2,4),(-2.69278601163599,-2.48949828257243,-2.28229533337829,
-2.14458879630755,-1.96754811547389,-1.79103983134423,-1.61387421528426,
-1.43688712002345,-1.34835665175354,-1.25978242305215,-1.08286142570342,
-0.905901114542216,-0.728942624529302,-0.640388431956018,-0.480377748967097,
-0.240145438538195,-0.120091889664005,-0.000154281172380586),
 .UNSPECIFIED.);
#30440=B_SPLINE_CURVE_WITH_KNOTS('',3,(#208632,#208633,#208634,#208635,
#208636,#208637,#208638,#208639,#208640,#208641,#208642,#208643,#208644,
#208645,#208646,#208647,#208648,#208649,#208650,#208651,#208652,#208653,
#208654,#208655,#208656,#208657,#208658,#208659,#208660,#208661,#208662,
#208663),.UNSPECIFIED.,.F.,.F.,(4,2,2,2,2,2,2,2,2,2,2,2,2,2,2,4),(-2.46530051632041,
-2.26819680103668,-2.0711954618087,-1.93999090652036,-1.76308472873804,
-1.58642929790919,-1.40948483540281,-1.23270430940088,-1.05614800855081,
-0.879169642198454,-0.70232687435545,-0.525413854333788,-0.394197725784304,
-0.197144745652711,-0.098600755514457,-0.00026354035724065),
 .UNSPECIFIED.);
#30441=B_SPLINE_CURVE_WITH_KNOTS('',3,(#208665,#208666,#208667,#208668,
#208669,#208670,#208671,#208672,#208673,#208674,#208675,#208676,#208677,
#208678,#208679,#208680,#208681,#208682,#208683,#208684,#208685,#208686,
#208687,#208688,#208689,#208690),.UNSPECIFIED.,.F.,.F.,(4,2,2,2,2,2,2,2,
2,2,2,2,4),(0.000318650702430989,0.313346654756281,0.619041496227019,0.795573539849274,
0.972003501309865,1.14847338462624,1.32604214603395,1.68155740636289,1.85805892632572,
2.01000672201703,2.23835919370013,2.35285672004845,2.46729888736451),
 .UNSPECIFIED.);
#30442=B_SPLINE_CURVE_WITH_KNOTS('',3,(#208691,#208692,#208693,#208694,
#208695,#208696,#208697,#208698,#208699,#208700,#208701,#208702,#208703,
#208704,#208705,#208706,#208707,#208708,#208709,#208710,#208711,#208712,
#208713,#208714,#208715,#208716,#208717,#208718,#208719,#208720,#208721,
#208722,#208723,#208724),.UNSPECIFIED.,.F.,.F.,(4,2,2,2,2,2,2,2,2,2,2,2,
2,2,2,2,4),(0.000172246164436567,0.137421022141082,0.274393772366344,0.548014374963287,
0.723403918543801,0.900115220230536,1.07657539273742,1.2530000195469,1.43023283105391,
1.78627983687558,1.87475797459756,2.05193109982066,2.14050606857681,2.31698437617588,
2.58688830258845,2.72343273743266,2.86001317919873),.UNSPECIFIED.);
#30443=B_SPLINE_CURVE_WITH_KNOTS('',3,(#208727,#208728,#208729,#208730,
#208731,#208732,#208733,#208734,#208735,#208736,#208737,#208738,#208739,
#208740,#208741,#208742,#208743,#208744,#208745,#208746,#208747,#208748,
#208749,#208750,#208751,#208752,#208753,#208754,#208755,#208756,#208757,
#208758,#208759,#208760),.UNSPECIFIED.,.F.,.F.,(4,2,2,2,2,2,2,2,2,2,2,2,
2,2,2,2,4),(-2.8604020772222,-2.72399588747906,-2.55750044548352,-2.37620089410916,
-2.22874860029063,-2.08275318086539,-1.92798249835796,-1.83854814703534,
-1.62320721676794,-1.45286930809083,-1.28281138427904,-1.1241953649196,
-0.967800004567202,-0.815712191339319,-0.636830671478215,-0.323116638129756,
-9.999999992516E-7),.UNSPECIFIED.);
#30444=B_SPLINE_CURVE_WITH_KNOTS('',3,(#208761,#208762,#208763,#208764,
#208765,#208766,#208767,#208768,#208769,#208770,#208771,#208772,#208773,
#208774,#208775,#208776,#208777,#208778,#208779,#208780,#208781,#208782,
#208783,#208784),.UNSPECIFIED.,.F.,.F.,(4,2,2,2,2,2,2,2,2,2,2,4),(-2.07371028241749,
-1.89670800669829,-1.71936907534134,-1.60400157839947,-1.44968076203279,
-1.09401343926072,-0.738422470297299,-0.650645320698835,-0.49885496807562,
-0.251161098077026,-0.127294929010069,-0.000361776623960997),
 .UNSPECIFIED.);
#30445=B_SPLINE_CURVE_WITH_KNOTS('',3,(#208786,#208787,#208788,#208789,
#208790,#208791,#208792,#208793,#208794,#208795,#208796,#208797,#208798,
#208799,#208800,#208801,#208802,#208803,#208804,#208805,#208806,#208807,
#208808,#208809,#208810,#208811),.UNSPECIFIED.,.F.,.F.,(4,2,2,2,2,2,2,2,
2,2,2,2,4),(0.000219774120001982,0.128265976878421,0.255769893159645,0.493856419136348,
0.651486942309498,0.821726852996698,1.03589976718762,1.25551703969407,1.39399885601373,
1.57317372451604,1.8211861086334,1.94515901785526,2.07223113354374),
 .UNSPECIFIED.);
#30446=B_SPLINE_CURVE_WITH_KNOTS('',3,(#208812,#208813,#208814,#208815,
#208816,#208817,#208818,#208819,#208820,#208821,#208822,#208823,#208824,
#208825,#208826,#208827,#208828,#208829,#208830,#208831,#208832,#208833,
#208834,#208835,#208836,#208837,#208838,#208839,#208840,#208841,#208842,
#208843,#208844,#208845),.UNSPECIFIED.,.F.,.F.,(4,2,2,2,2,2,2,2,2,2,2,2,
2,2,2,2,4),(-20.0267697459016,-19.7034013542535,-19.3891929917687,-19.2102906022386,
-19.0571883022074,-18.9019968771614,-18.7436220861097,-18.5735973213373,
-18.4032735363198,-18.1880846617368,-18.0986525161132,-17.9441161047557,
-17.7977744331096,-17.6503832691351,-17.4690817117426,-17.3026231029396,
-17.166235588483),.UNSPECIFIED.);
#30447=B_SPLINE_CURVE_WITH_KNOTS('',3,(#208848,#208849,#208850,#208851,
#208852,#208853,#208854,#208855,#208856,#208857,#208858,#208859,#208860,
#208861,#208862,#208863,#208864,#208865,#208866,#208867,#208868,#208869,
#208870,#208871,#208872,#208873,#208874,#208875,#208876,#208877,#208878,
#208879),.UNSPECIFIED.,.F.,.F.,(4,2,2,2,2,2,2,2,2,2,2,2,2,2,2,4),(-2.8610678083529,
-2.77118001727313,-2.62423597662898,-2.47550480424851,-2.17505208121599,
-1.8194196555836,-1.64521569280835,-1.4743719964416,-1.30309359694003,-1.1333766862558,
-0.917899747742497,-0.74777190157107,-0.576876204814989,-0.435632361078004,
-0.28735165256909,-9.99999999695689E-7),.UNSPECIFIED.);
#30448=B_SPLINE_CURVE_WITH_KNOTS('',3,(#208881,#208882,#208883,#208884,
#208885,#208886,#208887,#208888,#208889,#208890,#208891,#208892,#208893,
#208894,#208895,#208896,#208897,#208898,#208899,#208900,#208901,#208902),
 .UNSPECIFIED.,.F.,.F.,(4,2,2,2,2,2,2,2,2,2,4),(-1.6783918973356,-1.54864602744031,
-1.41972171226195,-1.17041428893027,-1.02310065652554,-0.854629785345839,
-0.705938566731539,-0.530158415550069,-0.26465166379874,-0.13428370906012,
-0.00063552929898788),.UNSPECIFIED.);
#30449=B_SPLINE_CURVE_WITH_KNOTS('',3,(#208904,#208905,#208906,#208907),
 .UNSPECIFIED.,.F.,.F.,(4,4),(0.,1.),.UNSPECIFIED.);
#30450=B_SPLINE_CURVE_WITH_KNOTS('',3,(#208909,#208910,#208911,#208912,
#208913,#208914,#208915,#208916,#208917,#208918,#208919,#208920,#208921,
#208922,#208923,#208924,#208925,#208926,#208927,#208928,#208929,#208930),
 .UNSPECIFIED.,.F.,.F.,(4,2,2,2,2,2,2,2,2,2,4),(0.000147978863487718,0.132665880139302,
0.264039836415925,0.521001553776919,0.701578774201878,0.83899587449096,
1.11207159356816,1.25225787140647,1.45962584134195,1.56800447112712,1.67810387049899),
 .UNSPECIFIED.);
#30451=B_SPLINE_CURVE_WITH_KNOTS('',3,(#208931,#208932,#208933,#208934,
#208935,#208936,#208937,#208938,#208939,#208940,#208941,#208942,#208943,
#208944,#208945,#208946,#208947,#208948,#208949,#208950,#208951,#208952,
#208953,#208954,#208955,#208956,#208957,#208958,#208959,#208960,#208961,
#208962),.UNSPECIFIED.,.F.,.F.,(4,2,2,2,2,2,2,2,2,2,2,2,2,2,2,4),(-20.0228897850774,
-19.7547732797997,-19.6058056189287,-19.4708760835207,-19.2549323436283,
-19.0852647002444,-18.8857336685939,-18.7179066463893,-18.5469453747283,
-18.3762608119982,-18.2022424489253,-17.8465788019333,-17.5488974776113,
-17.3980719908646,-17.2515164719589,-17.1620566513902),.UNSPECIFIED.);
#30452=B_SPLINE_CURVE_WITH_KNOTS('',3,(#208992,#208993,#208994,#208995,
#208996,#208997,#208998,#208999,#209000,#209001,#209002,#209003,#209004,
#209005,#209006,#209007,#209008,#209009,#209010),.UNSPECIFIED.,.F.,.F.,
(4,3,3,3,3,3,4),(0.,0.188384660261452,0.240000922766572,0.500001230410849,
0.760001538055127,0.945884007376155,0.999999610267735),.UNSPECIFIED.);
#30453=B_SPLINE_CURVE_WITH_KNOTS('',3,(#209013,#209014,#209015,#209016,
#209017,#209018,#209019,#209020,#209021,#209022,#209023,#209024,#209025,
#209026),.UNSPECIFIED.,.F.,.F.,(4,2,2,2,2,2,4),(0.000337787465763639,0.284976578385995,
0.575874331198097,0.935643861114864,1.30221214423588,1.60875324692267,1.91914645332358),
 .UNSPECIFIED.);
#30454=B_SPLINE_CURVE_WITH_KNOTS('',3,(#209297,#209298,#209299,#209300,
#209301,#209302,#209303,#209304,#209305,#209306,#209307,#209308,#209309,
#209310,#209311,#209312,#209313,#209314,#209315,#209316,#209317,#209318,
#209319,#209320,#209321,#209322,#209323,#209324,#209325,#209326,#209327,
#209328,#209329,#209330,#209331,#209332,#209333,#209334),.UNSPECIFIED.,
 .F.,.F.,(4,2,2,2,2,2,2,2,2,2,2,2,2,2,2,2,2,2,4),(-25.3605959634744,-25.2299176631067,
-25.1016543086936,-24.859881463169,-24.6979355907445,-24.3835783247934,
-24.2847913992405,-23.9723612276356,-23.8735088087347,-23.5593401804643,
-23.4605396458714,-23.1477400987566,-22.9907821446129,-22.8912511255084,
-22.4856054757622,-22.1082880433666,-21.9057075956864,-21.7029412164806,
-21.689764260827),.UNSPECIFIED.);
#30455=B_SPLINE_CURVE_WITH_KNOTS('',3,(#209604,#209605,#209606,#209607,
#209608,#209609),.UNSPECIFIED.,.F.,.F.,(4,2,4),(1.30310740020753E-6,0.0653973385639156,
0.130262424727681),.UNSPECIFIED.);
#30456=B_SPLINE_CURVE_WITH_KNOTS('',3,(#209638,#209639,#209640,#209641,
#209642,#209643),.UNSPECIFIED.,.F.,.F.,(4,2,4),(-0.0180566566914832,-0.00903372775874852,
-8.36277988998135E-7),.UNSPECIFIED.);
#30457=B_SPLINE_CURVE_WITH_KNOTS('',3,(#209645,#209646,#209647,#209648,
#209649,#209650),.UNSPECIFIED.,.F.,.F.,(4,2,4),(-0.0180610510695298,-0.00903269966892605,
-5.26550410692647E-6),.UNSPECIFIED.);
#30458=B_SPLINE_CURVE_WITH_KNOTS('',3,(#209679,#209680,#209681,#209682,
#209683,#209684),.UNSPECIFIED.,.F.,.F.,(4,2,4),(0.000679919887194027,0.0656077343225083,
0.130948244492649),.UNSPECIFIED.);
#30459=B_SPLINE_CURVE_WITH_KNOTS('',3,(#210299,#210300,#210301,#210302,
#210303,#210304),.UNSPECIFIED.,.F.,.F.,(4,2,4),(1.37679443180464E-6,0.132788624167646,
0.261946710422712),.UNSPECIFIED.);
#30460=B_SPLINE_CURVE_WITH_KNOTS('',3,(#210305,#210306,#210307,#210308,
#210309,#210310),.UNSPECIFIED.,.F.,.F.,(4,2,4),(9.69834488243248E-6,0.0602748062235942,
0.119740503039534),.UNSPECIFIED.);
#30461=B_SPLINE_CURVE_WITH_KNOTS('',3,(#210323,#210324,#210325,#210326,
#210327,#210328,#210329,#210330,#210331,#210332),.UNSPECIFIED.,.F.,.F.,
(4,2,2,2,4),(2.46055889067629,2.77696986044635,3.16672845187631,3.55648704330627,
3.87289801307632),.UNSPECIFIED.);
#30462=B_SPLINE_CURVE_WITH_KNOTS('',3,(#210334,#210335,#210336,#210337,
#210338,#210339),.UNSPECIFIED.,.F.,.F.,(4,2,4),(3.76834231838167E-5,0.27701452139551,
0.555926380958724),.UNSPECIFIED.);
#30463=B_SPLINE_CURVE_WITH_KNOTS('',3,(#210369,#210370,#210371,#210372,
#210373,#210374,#210375,#210376,#210377,#210378,#210379,#210380,#210381,
#210382,#210383,#210384,#210385,#210386,#210387),.UNSPECIFIED.,.F.,.F.,
(4,3,3,3,3,3,4),(0.,0.176916349750736,0.240000637218415,0.500000956530079,
0.760001275841745,0.935051760779978,0.999999692665182),.UNSPECIFIED.);
#30464=B_SPLINE_CURVE_WITH_KNOTS('',3,(#210390,#210391,#210392,#210393,
#210394,#210395,#210396,#210397,#210398,#210399,#210400,#210401,#210402,
#210403),.UNSPECIFIED.,.F.,.F.,(4,2,2,2,2,2,4),(0.000167093672002118,0.369844031545408,
0.745935182508687,1.21004916822787,1.6809812805177,2.07272751301276,2.4680790456475),
 .UNSPECIFIED.);
#30465=B_SPLINE_CURVE_WITH_KNOTS('',3,(#210545,#210546,#210547,#210548,
#210549,#210550,#210551,#210552,#210553,#210554,#210555,#210556,#210557,
#210558,#210559,#210560,#210561,#210562,#210563,#210564,#210565,#210566,
#210567,#210568,#210569,#210570,#210571,#210572,#210573,#210574,#210575,
#210576,#210577,#210578,#210579,#210580,#210581,#210582,#210583,#210584,
#210585,#210586,#210587,#210588,#210589,#210590,#210591,#210592,#210593,
#210594,#210595,#210596,#210597,#210598,#210599,#210600,#210601,#210602,
#210603,#210604,#210605,#210606,#210607,#210608,#210609,#210610,#210611,
#210612,#210613,#210614,#210615,#210616,#210617,#210618,#210619,#210620,
#210621,#210622,#210623,#210624,#210625,#210626,#210627,#210628,#210629,
#210630,#210631,#210632,#210633,#210634,#210635,#210636,#210637,#210638,
#210639,#210640,#210641,#210642,#210643,#210644,#210645,#210646,#210647,
#210648,#210649,#210650,#210651,#210652,#210653,#210654,#210655,#210656,
#210657,#210658,#210659,#210660,#210661,#210662,#210663,#210664,#210665,
#210666,#210667,#210668,#210669,#210670,#210671,#210672,#210673,#210674,
#210675,#210676,#210677,#210678,#210679,#210680,#210681,#210682,#210683,
#210684,#210685,#210686,#210687,#210688,#210689,#210690,#210691,#210692,
#210693,#210694,#210695,#210696,#210697,#210698,#210699,#210700,#210701,
#210702,#210703,#210704,#210705,#210706,#210707,#210708,#210709,#210710,
#210711,#210712,#210713,#210714,#210715,#210716,#210717,#210718,#210719,
#210720,#210721,#210722,#210723,#210724,#210725,#210726,#210727,#210728,
#210729,#210730,#210731,#210732,#210733,#210734,#210735,#210736,#210737,
#210738,#210739,#210740,#210741,#210742,#210743,#210744,#210745,#210746,
#210747,#210748,#210749,#210750),.UNSPECIFIED.,.F.,.F.,(4,2,2,2,2,2,2,2,
2,2,2,2,2,2,2,2,2,2,2,2,2,2,2,2,2,2,2,2,2,2,2,2,2,2,2,2,2,2,2,2,2,2,2,2,
2,2,2,2,2,2,2,2,2,2,2,2,2,2,2,2,2,2,2,2,2,2,2,2,2,2,2,2,2,2,2,2,2,2,2,2,
2,2,2,2,2,2,2,2,2,2,2,2,2,2,2,2,2,2,2,2,2,2,4),(0.00107990835998589,0.0329071537590182,
0.195893328033104,0.355153898355014,0.434988215509004,0.642816516674076,
0.737569287381765,0.908716883124716,0.993153014695592,1.18963661548505,
1.28754502534697,1.47339632996793,1.55811137750697,1.76173951263956,1.85370473288822,
2.02895304659489,2.11938121696687,2.33665348563873,2.4229728740814,2.59661267496729,
2.68840363087139,2.90216045936439,2.98711838103119,3.1734242939562,3.26349749387919,
3.45824610570519,3.54619696517821,3.73710767095252,3.83188019060896,4.03301640764842,
4.1174764626154,4.30305199918925,4.40238831686129,4.60868154531538,4.68987410516886,
4.87477538174019,4.97656143336439,5.17614663824206,5.25912879747928,5.44612356898342,
5.55060337109826,5.7420288787186,5.82728553412066,6.01648422296294,6.12403067649721,
6.30698556070633,6.39486121220803,6.59463365048308,6.70174065578835,6.86827502056953,
6.957226649254,7.16281963592479,7.27369262076292,7.43009960965057,7.5220123839873,
7.70970084821241,7.83380812566714,7.98940531492064,8.08401416975494,8.26759687546506,
8.40024551700738,8.54235987947,8.63766384309952,8.81511758034529,9.02203998410492,
9.12411504839395,9.27578319432331,9.43003056609417,9.6064767873789,9.70887427476012,
9.85136721032997,10.0286666133371,10.1832040076769,10.2906557504572,10.4409835687639,
10.7071639933474,10.8497640564256,11.0174209495745,11.3445265446232,11.4731243770269,
11.6129658838983,11.9583938225873,12.0723592156197,12.2439881908159,12.4769173317724,
12.6198592275825,12.7939302219618,13.0253846296432,13.188025339889,13.3844928168393,
13.6178785486688,13.7866824791461,14.047968468405,14.5213773907695,14.7566219201825,
14.8883214848249,15.2208691883029,15.4554942000865,15.9304221828407,16.0434638694231,
16.5048987708617,16.8936209742175,17.2855462784105),.UNSPECIFIED.);
#30466=B_SPLINE_CURVE_WITH_KNOTS('',3,(#210752,#210753,#210754,#210755,
#210756,#210757,#210758,#210759,#210760,#210761,#210762,#210763,#210764,
#210765,#210766,#210767,#210768,#210769,#210770,#210771,#210772,#210773,
#210774,#210775,#210776,#210777,#210778,#210779,#210780,#210781,#210782,
#210783,#210784,#210785,#210786,#210787,#210788,#210789,#210790,#210791,
#210792,#210793,#210794,#210795,#210796,#210797,#210798,#210799,#210800,
#210801,#210802,#210803,#210804,#210805,#210806,#210807,#210808,#210809,
#210810,#210811,#210812,#210813,#210814,#210815,#210816,#210817,#210818,
#210819,#210820,#210821,#210822,#210823,#210824,#210825,#210826,#210827,
#210828,#210829,#210830,#210831,#210832,#210833,#210834,#210835,#210836),
 .UNSPECIFIED.,.F.,.F.,(4,3,3,3,3,3,3,3,3,3,3,3,3,3,3,3,3,3,3,3,3,3,3,3,
3,3,3,3,4),(0.,0.047552339646909,0.0945933459078274,0.141741666696633,0.18879608789237,
0.236701745213095,0.246392852639966,0.250474334099904,0.297627468266538,
0.344829936104484,0.380418717175272,0.427580266713761,0.474808467386502,
0.496867832817848,0.502907306283412,0.549192807164965,0.595728951546223,
0.642323912201335,0.688682512723011,0.723451463114268,0.738537131268896,
0.747378843505563,0.752846656310363,0.801913023150851,0.827758314288039,
0.876702333074763,0.925834305036086,0.974954869278943,0.999217082393029),
 .UNSPECIFIED.);
#30467=B_SPLINE_CURVE_WITH_KNOTS('',3,(#210838,#210839,#210840,#210841),
 .UNSPECIFIED.,.F.,.F.,(4,4),(-0.000244606540981952,0.),.UNSPECIFIED.);
#30468=B_SPLINE_CURVE_WITH_KNOTS('',3,(#210842,#210843,#210844,#210845,
#210846,#210847,#210848,#210849,#210850,#210851,#210852,#210853,#210854,
#210855,#210856,#210857,#210858,#210859,#210860,#210861,#210862,#210863,
#210864,#210865,#210866,#210867,#210868,#210869,#210870,#210871,#210872,
#210873,#210874,#210875,#210876,#210877,#210878,#210879,#210880,#210881,
#210882,#210883,#210884,#210885,#210886,#210887,#210888,#210889,#210890,
#210891,#210892,#210893,#210894,#210895,#210896,#210897,#210898,#210899,
#210900,#210901,#210902,#210903,#210904,#210905,#210906,#210907,#210908,
#210909,#210910,#210911,#210912,#210913,#210914,#210915,#210916,#210917,
#210918,#210919,#210920,#210921,#210922,#210923,#210924,#210925,#210926,
#210927,#210928,#210929,#210930,#210931,#210932,#210933,#210934,#210935,
#210936,#210937,#210938,#210939,#210940,#210941,#210942,#210943,#210944,
#210945,#210946,#210947,#210948,#210949,#210950,#210951,#210952,#210953,
#210954,#210955,#210956,#210957,#210958,#210959,#210960,#210961,#210962,
#210963,#210964,#210965,#210966,#210967,#210968,#210969,#210970,#210971,
#210972,#210973,#210974,#210975,#210976,#210977,#210978,#210979,#210980,
#210981,#210982,#210983,#210984,#210985,#210986,#210987,#210988,#210989,
#210990,#210991,#210992,#210993,#210994,#210995,#210996,#210997,#210998,
#210999,#211000,#211001,#211002,#211003,#211004,#211005,#211006,#211007,
#211008,#211009,#211010,#211011,#211012,#211013,#211014,#211015,#211016,
#211017,#211018,#211019),.UNSPECIFIED.,.F.,.F.,(4,2,2,2,2,2,2,2,2,2,2,2,
2,2,2,2,2,2,2,2,2,2,2,2,2,2,2,2,2,2,2,2,2,2,2,2,2,2,2,2,2,2,2,2,2,2,2,2,
2,2,2,2,2,2,2,2,2,2,2,2,2,2,2,2,2,2,2,2,2,2,2,2,2,2,2,2,2,2,2,2,2,2,2,2,
2,2,2,2,4),(-17.8874346104741,-17.5294919406818,-17.186048243618,-16.9295394703044,
-16.8092492886893,-16.1896824714199,-15.8340272539635,-15.2083864407959,
-14.9204681111906,-14.3899595901558,-14.1556344485288,-13.9783598067019,
-13.7492496008297,-13.5994074640869,-13.4666029323457,-13.36660794238,-13.154214154486,
-12.9906873703296,-12.887536511039,-12.7359106835424,-12.5879560881589,
-12.4262389067138,-12.325210118249,-12.1497599741407,-12.0316602780003,
-11.844332676878,-11.7509492084952,-11.5889580967691,-11.4836693199961,
-11.2966545631598,-11.192487027676,-11.0521608686276,-10.9450814860788,
-10.7612433258855,-10.6366324078592,-10.4865596856504,-10.346504062992,
-10.1283588143909,-10.0182524554306,-9.89616481205125,-9.58905421185916,
-9.07549190179132,-8.68076130995556,-8.46605691773842,-8.01018323272566,
-7.6210762100739,-7.24137219648118,-6.65939456135951,-6.42566825698983,
-6.19571944234743,-5.93321022345773,-5.81507259108846,-5.6394297626821,
-5.45310433689612,-5.2600764092861,-5.15380952310406,-5.03637349809631,
-4.82334403415801,-4.68443024678171,-4.54527121636483,-4.4172699568073,
-4.24519534314461,-4.1387700467407,-4.00127907201438,-3.88561719144662,
-3.73605126424484,-3.64032051175329,-3.46696552173688,-3.36568283466442,
-3.21304464574596,-3.10894067512593,-2.93016448528719,-2.83463383876123,
-2.67405588966363,-2.53885135281782,-2.39350009266653,-2.2994834121646,
-2.13842813199443,-1.95939869234199,-1.82841008968958,-1.69294839797772,
-1.5518629856045,-1.33346072700906,-1.18729433138863,-0.994382017820723,
-0.767650200558565,-0.680987224726351,-0.341206102852212,-0.000193437912456803),
 .UNSPECIFIED.);
#30469=B_SPLINE_CURVE_WITH_KNOTS('',3,(#211289,#211290,#211291,#211292,
#211293,#211294),.UNSPECIFIED.,.F.,.F.,(4,2,4),(-0.131003728994287,-0.0656099055372978,
-3.86587579667962E-6),.UNSPECIFIED.);
#30470=B_SPLINE_CURVE_WITH_KNOTS('',3,(#211296,#211297,#211298,#211299,
#211300,#211301,#211302,#211303,#211304,#211305,#211306,#211307,#211308,
#211309,#211310,#211311,#211312,#211313,#211314,#211315,#211316,#211317,
#211318,#211319,#211320,#211321,#211322,#211323,#211324,#211325,#211326,
#211327,#211328,#211329,#211330,#211331,#211332,#211333,#211334,#211335,
#211336,#211337,#211338,#211339,#211340,#211341,#211342,#211343,#211344,
#211345,#211346,#211347,#211348,#211349,#211350,#211351,#211352,#211353),
 .UNSPECIFIED.,.F.,.F.,(4,2,2,2,2,2,2,2,2,2,2,2,2,2,2,2,2,2,2,2,2,2,2,2,
2,2,2,2,4),(-6.15860212849669,-6.06515038114135,-5.83681474701059,-5.60593974251633,
-5.31433449222845,-5.18909714071076,-4.9413569458906,-4.68314415669207,
-4.55804547761989,-4.30742774828901,-4.06523839474389,-3.80702431616562,
-3.68220920617004,-3.43109416439227,-3.17048590815028,-2.91233401200879,
-2.78665746308759,-2.52874309402958,-2.25501193498755,-2.13006946787647,
-1.75457334893578,-1.62820215757801,-1.43603946055039,-1.20517175944087,
-0.920799061189383,-0.807044726910511,-0.445490300674665,-0.334664291987655,
-3.49174065404852E-5),.UNSPECIFIED.);
#30471=B_SPLINE_CURVE_WITH_KNOTS('',3,(#211382,#211383,#211384,#211385,
#211386,#211387),.UNSPECIFIED.,.F.,.F.,(4,2,4),(-0.0180614175475543,-0.00903747414230311,
-8.04914190790971E-7),.UNSPECIFIED.);
#30472=B_SPLINE_CURVE_WITH_KNOTS('',3,(#211388,#211389,#211390,#211391,
#211392,#211393,#211394,#211395,#211396,#211397,#211398,#211399,#211400,
#211401),.UNSPECIFIED.,.F.,.F.,(4,2,2,2,2,2,4),(1.00000038869935E-6,0.377507126467116,
0.760172295625594,1.01061719312917,1.51716116734711,1.76732387692719,2.02167921549907),
 .UNSPECIFIED.);
#30473=B_SPLINE_CURVE_WITH_KNOTS('',3,(#211403,#211404,#211405,#211406,
#211407,#211408),.UNSPECIFIED.,.F.,.F.,(4,2,4),(-0.0180670199973744,-0.00903616121666639,
-6.43699294978515E-6),.UNSPECIFIED.);
#30474=B_SPLINE_CURVE_WITH_KNOTS('',3,(#211437,#211438,#211439,#211440,
#211441,#211442),.UNSPECIFIED.,.F.,.F.,(4,2,4),(-0.131007272486104,-0.0654519130722608,
-7.32542528862561E-6),.UNSPECIFIED.);
#30475=B_SPLINE_CURVE_WITH_KNOTS('',3,(#211711,#211712,#211713,#211714,
#211715,#211716,#211717,#211718,#211719,#211720,#211721,#211722,#211723,
#211724,#211725,#211726,#211727,#211728,#211729,#211730,#211731,#211732,
#211733,#211734,#211735,#211736,#211737,#211738,#211739,#211740,#211741,
#211742,#211743,#211744,#211745,#211746,#211747,#211748,#211749,#211750,
#211751,#211752,#211753,#211754,#211755,#211756,#211757,#211758,#211759,
#211760,#211761,#211762,#211763,#211764,#211765,#211766,#211767,#211768,
#211769,#211770,#211771,#211772,#211773,#211774,#211775,#211776,#211777,
#211778,#211779,#211780,#211781,#211782,#211783,#211784,#211785,#211786,
#211787,#211788),.UNSPECIFIED.,.F.,.F.,(4,2,2,2,2,2,2,2,2,2,2,2,2,2,2,2,
2,2,2,2,2,2,2,2,2,2,2,2,2,2,2,2,2,2,2,2,2,2,4),(-20.9312459291626,-20.8238269097937,
-20.5931648525945,-20.3353373519583,-20.1701043049685,-19.9383799110844,
-19.702397418043,-19.451963635314,-19.3267742859618,-19.0685720740393,-18.8337543042022,
-18.5759062577988,-18.4504717029174,-18.1922860321218,-17.9373418768597,
-17.6863787711074,-17.5614775151041,-17.3032678569112,-17.0594109215148,
-16.8087504776042,-16.6471745738218,-16.4156901290353,-16.1896876711962,
-16.0642108166878,-15.7633972745444,-15.5054078770155,-15.3311008092168,
-15.0986958752912,-14.8699701821476,-14.6121430096181,-14.4868124487622,
-14.2286099369188,-13.9920525360736,-13.7605761499709,-13.5444790500576,
-13.3280590731181,-13.0965913797703,-12.8599164248024,-12.7553611554937),
 .UNSPECIFIED.);
#30476=B_SPLINE_CURVE_WITH_KNOTS('',3,(#212200,#212201,#212202,#212203,
#212204,#212205),.UNSPECIFIED.,.F.,.F.,(4,2,4),(-0.344875729523264,-0.172579825677985,
-3.94566552320122E-5),.UNSPECIFIED.);
#30477=B_SPLINE_CURVE_WITH_KNOTS('',3,(#212206,#212207,#212208,#212209),
 .UNSPECIFIED.,.F.,.F.,(4,4),(-0.000257082057276752,0.),.UNSPECIFIED.);
#30478=B_SPLINE_CURVE_WITH_KNOTS('',3,(#212621,#212622,#212623,#212624,
#212625,#212626),.UNSPECIFIED.,.F.,.F.,(4,2,4),(-0.344703474824345,-0.172091835354049,
-0.00130738802397509),.UNSPECIFIED.);
#30479=B_SPLINE_CURVE_WITH_KNOTS('',3,(#212627,#212628,#212629,#212630),
 .UNSPECIFIED.,.F.,.F.,(4,4),(-0.00138054251324295,0.),.UNSPECIFIED.);
#30480=B_SPLINE_CURVE_WITH_KNOTS('',3,(#212657,#212658,#212659,#212660,
#212661,#212662),.UNSPECIFIED.,.F.,.F.,(4,2,4),(0.000411407934210648,0.132395690524123,
0.265296797891605),.UNSPECIFIED.);
#30481=B_SPLINE_CURVE_WITH_KNOTS('',3,(#212665,#212666,#212667,#212668),
 .UNSPECIFIED.,.F.,.F.,(4,4),(0.,0.000434666445632145),.UNSPECIFIED.);
#30482=B_SPLINE_CURVE_WITH_KNOTS('',3,(#212670,#212671,#212672,#212673,
#212674,#212675,#212676,#212677,#212678,#212679,#212680,#212681,#212682,
#212683,#212684,#212685,#212686,#212687,#212688,#212689,#212690,#212691),
 .UNSPECIFIED.,.F.,.F.,(4,2,2,2,2,2,2,2,2,2,4),(0.,0.144173778921579,0.288103676995469,
0.573727861047774,0.772563733388318,1.17379786176643,1.57506737125788,1.77392881725764,
1.91671525972644,2.13148394854954,2.34639580468694),.UNSPECIFIED.);
#30483=B_SPLINE_CURVE_WITH_KNOTS('',3,(#212692,#212693,#212694,#212695),
 .UNSPECIFIED.,.F.,.F.,(4,4),(4.93459806199749E-5,5.07374035525052E-5),
 .UNSPECIFIED.);
#30484=B_SPLINE_CURVE_WITH_KNOTS('',3,(#212774,#212775,#212776,#212777,
#212778,#212779,#212780,#212781,#212782,#212783),.UNSPECIFIED.,.F.,.F.,
(4,2,2,2,4),(2.44487072892702,2.76003095423418,3.15004164386436,3.54005233349455,
3.85521255880171),.UNSPECIFIED.);
#33524=CIRCLE('',#85969,10.25);
#33525=CIRCLE('',#85970,10.25);
#33526=CIRCLE('',#85979,13.);
#33527=CIRCLE('',#85981,13.);
#33528=CIRCLE('',#85989,13.);
#33529=CIRCLE('',#85990,13.);
#33530=CIRCLE('',#85992,12.00000442428);
#33531=CIRCLE('',#86002,9.08769033371916);
#33532=CIRCLE('',#86004,4.9028521085786);
#33533=CIRCLE('',#86012,10.25);
#33534=CIRCLE('',#86013,9.250003127107);
#33535=CIRCLE('',#86015,10.25);
#33536=CIRCLE('',#86021,11.4812930575157);
#33537=CIRCLE('',#86024,9.08769033371916);
#33538=CIRCLE('',#86029,66.65911415553);
#33539=CIRCLE('',#86030,66.65911415553);
#33540=CIRCLE('',#86031,67.66415225213);
#33541=CIRCLE('',#86033,68.);
#33542=CIRCLE('',#86034,67.66415225213);
#33543=CIRCLE('',#86039,10.5);
#33544=CIRCLE('',#86040,10.5);
#33545=CIRCLE('',#86041,10.5);
#33546=CIRCLE('',#86043,11.0000062575399);
#33547=CIRCLE('',#86047,7.75);
#33548=CIRCLE('',#86049,7.75);
#33549=CIRCLE('',#86051,8.249994983965);
#33550=CIRCLE('',#86055,66.65911415553);
#33551=CIRCLE('',#86056,67.);
#40749=VERTEX_POINT('',#203968);
#40750=VERTEX_POINT('',#203969);
#40751=VERTEX_POINT('',#203971);
#40752=VERTEX_POINT('',#204036);
#40753=VERTEX_POINT('',#204038);
#40754=VERTEX_POINT('',#204041);
#40755=VERTEX_POINT('',#204064);
#40756=VERTEX_POINT('',#204077);
#40757=VERTEX_POINT('',#204088);
#40758=VERTEX_POINT('',#204090);
#40759=VERTEX_POINT('',#204101);
#40760=VERTEX_POINT('',#204139);
#40761=VERTEX_POINT('',#204140);
#40762=VERTEX_POINT('',#204281);
#40763=VERTEX_POINT('',#204282);
#40764=VERTEX_POINT('',#204415);
#40765=VERTEX_POINT('',#204416);
#40766=VERTEX_POINT('',#204418);
#40767=VERTEX_POINT('',#204552);
#40768=VERTEX_POINT('',#204553);
#40769=VERTEX_POINT('',#204623);
#40770=VERTEX_POINT('',#204691);
#40771=VERTEX_POINT('',#204692);
#40772=VERTEX_POINT('',#204829);
#40773=VERTEX_POINT('',#204830);
#40774=VERTEX_POINT('',#204965);
#40775=VERTEX_POINT('',#204966);
#40776=VERTEX_POINT('',#204968);
#40777=VERTEX_POINT('',#205094);
#40778=VERTEX_POINT('',#205095);
#40779=VERTEX_POINT('',#205097);
#40780=VERTEX_POINT('',#205108);
#40781=VERTEX_POINT('',#205109);
#40782=VERTEX_POINT('',#205175);
#40783=VERTEX_POINT('',#205177);
#40784=VERTEX_POINT('',#205182);
#40785=VERTEX_POINT('',#205242);
#40786=VERTEX_POINT('',#205243);
#40787=VERTEX_POINT('',#205245);
#40788=VERTEX_POINT('',#205385);
#40789=VERTEX_POINT('',#205386);
#40790=VERTEX_POINT('',#205466);
#40791=VERTEX_POINT('',#205550);
#40792=VERTEX_POINT('',#205551);
#40793=VERTEX_POINT('',#205710);
#40794=VERTEX_POINT('',#205711);
#40795=VERTEX_POINT('',#205713);
#40796=VERTEX_POINT('',#205877);
#40797=VERTEX_POINT('',#205878);
#40798=VERTEX_POINT('',#205958);
#40799=VERTEX_POINT('',#206042);
#40800=VERTEX_POINT('',#206043);
#40801=VERTEX_POINT('',#206202);
#40802=VERTEX_POINT('',#206203);
#40803=VERTEX_POINT('',#206206);
#40804=VERTEX_POINT('',#206208);
#40805=VERTEX_POINT('',#206215);
#40806=VERTEX_POINT('',#206217);
#40807=VERTEX_POINT('',#206224);
#40808=VERTEX_POINT('',#206226);
#40809=VERTEX_POINT('',#206302);
#40810=VERTEX_POINT('',#206304);
#40811=VERTEX_POINT('',#206309);
#40812=VERTEX_POINT('',#206356);
#40813=VERTEX_POINT('',#206417);
#40814=VERTEX_POINT('',#206418);
#40815=VERTEX_POINT('',#206420);
#40816=VERTEX_POINT('',#206425);
#40817=VERTEX_POINT('',#206438);
#40818=VERTEX_POINT('',#206453);
#40819=VERTEX_POINT('',#206520);
#40820=VERTEX_POINT('',#206587);
#40821=VERTEX_POINT('',#206588);
#40822=VERTEX_POINT('',#206735);
#40823=VERTEX_POINT('',#206736);
#40824=VERTEX_POINT('',#206879);
#40825=VERTEX_POINT('',#206880);
#40826=VERTEX_POINT('',#206882);
#40827=VERTEX_POINT('',#206887);
#40828=VERTEX_POINT('',#206896);
#40829=VERTEX_POINT('',#206907);
#40830=VERTEX_POINT('',#206974);
#40831=VERTEX_POINT('',#207041);
#40832=VERTEX_POINT('',#207042);
#40833=VERTEX_POINT('',#207169);
#40834=VERTEX_POINT('',#207170);
#40835=VERTEX_POINT('',#207315);
#40836=VERTEX_POINT('',#207316);
#40837=VERTEX_POINT('',#207318);
#40838=VERTEX_POINT('',#207323);
#40839=VERTEX_POINT('',#207332);
#40840=VERTEX_POINT('',#207333);
#40841=VERTEX_POINT('',#207335);
#40842=VERTEX_POINT('',#207410);
#40843=VERTEX_POINT('',#207485);
#40844=VERTEX_POINT('',#207486);
#40845=VERTEX_POINT('',#207643);
#40846=VERTEX_POINT('',#207644);
#40847=VERTEX_POINT('',#207801);
#40848=VERTEX_POINT('',#207802);
#40849=VERTEX_POINT('',#207804);
#40850=VERTEX_POINT('',#207809);
#40851=VERTEX_POINT('',#207834);
#40852=VERTEX_POINT('',#207859);
#40853=VERTEX_POINT('',#207936);
#40854=VERTEX_POINT('',#208017);
#40855=VERTEX_POINT('',#208018);
#40856=VERTEX_POINT('',#208179);
#40857=VERTEX_POINT('',#208180);
#40858=VERTEX_POINT('',#208337);
#40859=VERTEX_POINT('',#208338);
#40860=VERTEX_POINT('',#208340);
#40861=VERTEX_POINT('',#208342);
#40862=VERTEX_POINT('',#208347);
#40863=VERTEX_POINT('',#208378);
#40864=VERTEX_POINT('',#208413);
#40865=VERTEX_POINT('',#208453);
#40866=VERTEX_POINT('',#208468);
#40867=VERTEX_POINT('',#208470);
#40868=VERTEX_POINT('',#208491);
#40869=VERTEX_POINT('',#208524);
#40870=VERTEX_POINT('',#208559);
#40871=VERTEX_POINT('',#208560);
#40872=VERTEX_POINT('',#208572);
#40873=VERTEX_POINT('',#208574);
#40874=VERTEX_POINT('',#208586);
#40875=VERTEX_POINT('',#208593);
#40876=VERTEX_POINT('',#208595);
#40877=VERTEX_POINT('',#208664);
#40878=VERTEX_POINT('',#208726);
#40879=VERTEX_POINT('',#208785);
#40880=VERTEX_POINT('',#208847);
#40881=VERTEX_POINT('',#208880);
#40882=VERTEX_POINT('',#208903);
#40883=VERTEX_POINT('',#208908);
#40884=VERTEX_POINT('',#208991);
#40885=VERTEX_POINT('',#209011);
#40886=VERTEX_POINT('',#209295);
#40887=VERTEX_POINT('',#210312);
#40888=VERTEX_POINT('',#210313);
#40889=VERTEX_POINT('',#210315);
#40890=VERTEX_POINT('',#210321);
#40891=VERTEX_POINT('',#210368);
#40892=VERTEX_POINT('',#210388);
#40893=VERTEX_POINT('',#210544);
#40894=VERTEX_POINT('',#210751);
#40895=VERTEX_POINT('',#210837);
#40896=VERTEX_POINT('',#211288);
#40897=VERTEX_POINT('',#212199);
#40898=VERTEX_POINT('',#212620);
#40899=VERTEX_POINT('',#212632);
#40900=VERTEX_POINT('',#212633);
#40901=VERTEX_POINT('',#212635);
#40902=VERTEX_POINT('',#212640);
#40903=VERTEX_POINT('',#212646);
#40904=VERTEX_POINT('',#212649);
#40905=VERTEX_POINT('',#212653);
#40906=VERTEX_POINT('',#212664);
#40907=VERTEX_POINT('',#212669);
#40908=VERTEX_POINT('',#212773);
#52001=EDGE_CURVE('',#40749,#40750,#9646,.T.);
#52002=EDGE_CURVE('',#40749,#40751,#30340,.F.);
#52003=EDGE_CURVE('',#40751,#40752,#9647,.T.);
#52004=EDGE_CURVE('',#40752,#40753,#33524,.T.);
#52005=EDGE_CURVE('',#40753,#40752,#33525,.T.);
#52006=EDGE_CURVE('',#40751,#40754,#30341,.F.);
#52007=EDGE_CURVE('',#40754,#40755,#30342,.T.);
#52008=EDGE_CURVE('',#40755,#40756,#30343,.T.);
#52009=EDGE_CURVE('',#40756,#40757,#9648,.T.);
#52010=EDGE_CURVE('',#40757,#40758,#30344,.T.);
#52011=EDGE_CURVE('',#40758,#40759,#30345,.T.);
#52012=EDGE_CURVE('',#40759,#40750,#30346,.F.);
#52013=EDGE_CURVE('',#40760,#40761,#9649,.T.);
#52014=EDGE_CURVE('',#40760,#40749,#30347,.F.);
#52015=EDGE_CURVE('',#40750,#40761,#30348,.F.);
#52016=EDGE_CURVE('',#40762,#40763,#9650,.T.);
#52017=EDGE_CURVE('',#40762,#40760,#30349,.F.);
#52018=EDGE_CURVE('',#40761,#40763,#30350,.F.);
#52019=EDGE_CURVE('',#40764,#40765,#9651,.T.);
#52020=EDGE_CURVE('',#40764,#40766,#30351,.F.);
#52021=EDGE_CURVE('',#40766,#40762,#30352,.F.);
#52022=EDGE_CURVE('',#40763,#40765,#30353,.F.);
#52023=EDGE_CURVE('',#40767,#40768,#9652,.T.);
#52024=EDGE_CURVE('',#40767,#40764,#30354,.F.);
#52025=EDGE_CURVE('',#40765,#40769,#30355,.F.);
#52026=EDGE_CURVE('',#40769,#40768,#30356,.F.);
#52027=EDGE_CURVE('',#40770,#40771,#9653,.T.);
#52028=EDGE_CURVE('',#40770,#40767,#30357,.F.);
#52029=EDGE_CURVE('',#40768,#40771,#30358,.F.);
#52030=EDGE_CURVE('',#40772,#40773,#9654,.T.);
#52031=EDGE_CURVE('',#40772,#40770,#30359,.F.);
#52032=EDGE_CURVE('',#40771,#40773,#30360,.F.);
#52033=EDGE_CURVE('',#40774,#40775,#9655,.T.);
#52034=EDGE_CURVE('',#40774,#40776,#30361,.T.);
#52035=EDGE_CURVE('',#40776,#40772,#30362,.F.);
#52036=EDGE_CURVE('',#40773,#40775,#30363,.F.);
#52037=EDGE_CURVE('',#40777,#40778,#9656,.T.);
#52038=EDGE_CURVE('',#40777,#40779,#30364,.T.);
#52039=EDGE_CURVE('',#40778,#40779,#33526,.T.);
#52040=EDGE_CURVE('',#40780,#40781,#9657,.T.);
#52041=EDGE_CURVE('',#40780,#40777,#30365,.T.);
#52042=EDGE_CURVE('',#40782,#40778,#33527,.T.);
#52043=EDGE_CURVE('',#40782,#40783,#30366,.T.);
#52044=EDGE_CURVE('',#40783,#40784,#30367,.T.);
#52045=EDGE_CURVE('',#40784,#40781,#30368,.F.);
#52046=EDGE_CURVE('',#40785,#40786,#9658,.T.);
#52047=EDGE_CURVE('',#40785,#40787,#30369,.T.);
#52048=EDGE_CURVE('',#40787,#40780,#30370,.T.);
#52049=EDGE_CURVE('',#40781,#40786,#30371,.F.);
#52050=EDGE_CURVE('',#40788,#40789,#9659,.T.);
#52051=EDGE_CURVE('',#40788,#40785,#30372,.T.);
#52052=EDGE_CURVE('',#40786,#40790,#30373,.F.);
#52053=EDGE_CURVE('',#40790,#40789,#30374,.F.);
#52054=EDGE_CURVE('',#40791,#40792,#9660,.T.);
#52055=EDGE_CURVE('',#40791,#40788,#30375,.T.);
#52056=EDGE_CURVE('',#40789,#40792,#30376,.F.);
#52057=EDGE_CURVE('',#40793,#40794,#9661,.T.);
#52058=EDGE_CURVE('',#40793,#40795,#30377,.F.);
#52059=EDGE_CURVE('',#40795,#40791,#30378,.T.);
#52060=EDGE_CURVE('',#40792,#40794,#30379,.F.);
#52061=EDGE_CURVE('',#40796,#40797,#9662,.T.);
#52062=EDGE_CURVE('',#40796,#40793,#30380,.F.);
#52063=EDGE_CURVE('',#40794,#40798,#30381,.F.);
#52064=EDGE_CURVE('',#40798,#40797,#30382,.F.);
#52065=EDGE_CURVE('',#40799,#40800,#9663,.T.);
#52066=EDGE_CURVE('',#40799,#40796,#30383,.F.);
#52067=EDGE_CURVE('',#40797,#40800,#30384,.F.);
#52068=EDGE_CURVE('',#40801,#40802,#33528,.T.);
#52069=EDGE_CURVE('',#40802,#40801,#33529,.T.);
#52070=EDGE_CURVE('',#40801,#40803,#9664,.T.);
#52071=EDGE_CURVE('',#40803,#40804,#30385,.T.);
#52072=EDGE_CURVE('',#40805,#40804,#9665,.T.);
#52073=EDGE_CURVE('',#40805,#40806,#30386,.T.);
#52074=EDGE_CURVE('',#40806,#40807,#9666,.T.);
#52075=EDGE_CURVE('',#40807,#40808,#30387,.F.);
#52076=EDGE_CURVE('',#40808,#40803,#30388,.T.);
#52077=EDGE_CURVE('',#40778,#40809,#9667,.T.);
#52078=EDGE_CURVE('',#40810,#40779,#30389,.T.);
#52079=EDGE_CURVE('',#40811,#40810,#30390,.F.);
#52080=EDGE_CURVE('',#40812,#40811,#33530,.T.);
#52081=EDGE_CURVE('',#40812,#40809,#30391,.T.);
#52082=EDGE_CURVE('',#40813,#40814,#9668,.T.);
#52083=EDGE_CURVE('',#40815,#40813,#30392,.F.);
#52084=EDGE_CURVE('',#40816,#40815,#30393,.T.);
#52085=EDGE_CURVE('',#40817,#40816,#9669,.T.);
#52086=EDGE_CURVE('',#40817,#40814,#30394,.T.);
#52087=EDGE_CURVE('',#40814,#40818,#30395,.T.);
#52088=EDGE_CURVE('',#40819,#40818,#9670,.T.);
#52089=EDGE_CURVE('',#40813,#40819,#30396,.F.);
#52090=EDGE_CURVE('',#40820,#40821,#9671,.T.);
#52091=EDGE_CURVE('',#40819,#40820,#30397,.F.);
#52092=EDGE_CURVE('',#40818,#40821,#30398,.T.);
#52093=EDGE_CURVE('',#40822,#40823,#9672,.T.);
#52094=EDGE_CURVE('',#40820,#40822,#30399,.F.);
#52095=EDGE_CURVE('',#40821,#40823,#30400,.T.);
#52096=EDGE_CURVE('',#40824,#40825,#9673,.T.);
#52097=EDGE_CURVE('',#40826,#40824,#30401,.F.);
#52098=EDGE_CURVE('',#40827,#40826,#30402,.T.);
#52099=EDGE_CURVE('',#40828,#40827,#9674,.T.);
#52100=EDGE_CURVE('',#40828,#40825,#30403,.T.);
#52101=EDGE_CURVE('',#40825,#40829,#30404,.T.);
#52102=EDGE_CURVE('',#40830,#40829,#9675,.T.);
#52103=EDGE_CURVE('',#40824,#40830,#30405,.F.);
#52104=EDGE_CURVE('',#40831,#40832,#9676,.T.);
#52105=EDGE_CURVE('',#40830,#40831,#30406,.F.);
#52106=EDGE_CURVE('',#40829,#40832,#30407,.T.);
#52107=EDGE_CURVE('',#40833,#40834,#9677,.T.);
#52108=EDGE_CURVE('',#40831,#40833,#30408,.F.);
#52109=EDGE_CURVE('',#40832,#40834,#30409,.T.);
#52110=EDGE_CURVE('',#40835,#40836,#9678,.T.);
#52111=EDGE_CURVE('',#40837,#40835,#30410,.T.);
#52112=EDGE_CURVE('',#40838,#40837,#30411,.T.);
#52113=EDGE_CURVE('',#40836,#40838,#33531,.T.);
#52114=EDGE_CURVE('',#40839,#40840,#9679,.T.);
#52115=EDGE_CURVE('',#40839,#40841,#30412,.T.);
#52116=EDGE_CURVE('',#40841,#40842,#33532,.T.);
#52117=EDGE_CURVE('',#40840,#40842,#30413,.F.);
#52118=EDGE_CURVE('',#40843,#40844,#9680,.T.);
#52119=EDGE_CURVE('',#40843,#40839,#30414,.T.);
#52120=EDGE_CURVE('',#40844,#40840,#30415,.F.);
#52121=EDGE_CURVE('',#40845,#40846,#9681,.T.);
#52122=EDGE_CURVE('',#40845,#40843,#30416,.T.);
#52123=EDGE_CURVE('',#40846,#40844,#30417,.F.);
#52124=EDGE_CURVE('',#40847,#40848,#9682,.T.);
#52125=EDGE_CURVE('',#40847,#40849,#30418,.T.);
#52126=EDGE_CURVE('',#40849,#40850,#30419,.T.);
#52127=EDGE_CURVE('',#40850,#40851,#9683,.T.);
#52128=EDGE_CURVE('',#40848,#40851,#30420,.T.);
#52129=EDGE_CURVE('',#40852,#40848,#30421,.F.);
#52130=EDGE_CURVE('',#40853,#40852,#9684,.T.);
#52131=EDGE_CURVE('',#40853,#40847,#30422,.T.);
#52132=EDGE_CURVE('',#40854,#40855,#9685,.T.);
#52133=EDGE_CURVE('',#40854,#40853,#30423,.T.);
#52134=EDGE_CURVE('',#40855,#40852,#30424,.F.);
#52135=EDGE_CURVE('',#40856,#40857,#9686,.T.);
#52136=EDGE_CURVE('',#40856,#40854,#30425,.T.);
#52137=EDGE_CURVE('',#40857,#40855,#30426,.F.);
#52138=EDGE_CURVE('',#40858,#40859,#9687,.T.);
#52139=EDGE_CURVE('',#40858,#40860,#33533,.T.);
#52140=EDGE_CURVE('',#40860,#40861,#30427,.T.);
#52141=EDGE_CURVE('',#40862,#40861,#30428,.T.);
#52142=EDGE_CURVE('',#40863,#40862,#30429,.T.);
#52143=EDGE_CURVE('',#40864,#40863,#33534,.T.);
#52144=EDGE_CURVE('',#40864,#40859,#30430,.T.);
#52145=EDGE_CURVE('',#40859,#40865,#30431,.T.);
#52146=EDGE_CURVE('',#40865,#40858,#33535,.T.);
#52147=EDGE_CURVE('',#40866,#40866,#2697,.T.);
#52148=EDGE_CURVE('',#40866,#40867,#9688,.T.);
#52149=EDGE_CURVE('',#40867,#40867,#2698,.T.);
#52150=EDGE_CURVE('',#40842,#40857,#30432,.F.);
#52151=EDGE_CURVE('',#40841,#40856,#30433,.T.);
#52152=EDGE_CURVE('',#40868,#40846,#30434,.F.);
#52153=EDGE_CURVE('',#40869,#40868,#33536,.T.);
#52154=EDGE_CURVE('',#40869,#40845,#30435,.T.);
#52155=EDGE_CURVE('',#40870,#40871,#30436,.T.);
#52156=EDGE_CURVE('',#40871,#40872,#9689,.T.);
#52157=EDGE_CURVE('',#40872,#40873,#30437,.T.);
#52158=EDGE_CURVE('',#40873,#40874,#30438,.T.);
#52159=EDGE_CURVE('',#40870,#40874,#9690,.T.);
#52160=EDGE_CURVE('',#40875,#40836,#33537,.T.);
#52161=EDGE_CURVE('',#40875,#40876,#30439,.T.);
#52162=EDGE_CURVE('',#40876,#40828,#30440,.T.);
#52163=EDGE_CURVE('',#40877,#40827,#30441,.T.);
#52164=EDGE_CURVE('',#40835,#40877,#30442,.T.);
#52165=EDGE_CURVE('',#40834,#40878,#30443,.T.);
#52166=EDGE_CURVE('',#40878,#40817,#30444,.T.);
#52167=EDGE_CURVE('',#40879,#40816,#30445,.T.);
#52168=EDGE_CURVE('',#40833,#40879,#30446,.F.);
#52169=EDGE_CURVE('',#40823,#40880,#30447,.T.);
#52170=EDGE_CURVE('',#40880,#40881,#30448,.T.);
#52171=EDGE_CURVE('',#40881,#40882,#30449,.T.);
#52172=EDGE_CURVE('',#40883,#40882,#30450,.T.);
#52173=EDGE_CURVE('',#40822,#40883,#30451,.F.);
#52174=EDGE_CURVE('',#40881,#40884,#30452,.T.);
#52175=EDGE_CURVE('',#40884,#40885,#9691,.T.);
#52176=EDGE_CURVE('',#40882,#40885,#30453,.T.);
#52177=EDGE_CURVE('',#40886,#40828,#9692,.T.);
#52178=EDGE_CURVE('',#40775,#40886,#30454,.F.);
#52179=EDGE_CURVE('',#40769,#40817,#9693,.T.);
#52180=EDGE_CURVE('',#40759,#40881,#30455,.T.);
#52181=EDGE_CURVE('',#40757,#40884,#30456,.T.);
#52182=EDGE_CURVE('',#40885,#40756,#30457,.T.);
#52183=EDGE_CURVE('',#40882,#40754,#30458,.T.);
#52184=EDGE_CURVE('',#40816,#40766,#9694,.T.);
#52185=EDGE_CURVE('',#40827,#40776,#9695,.T.);
#52186=EDGE_CURVE('',#40863,#40875,#30459,.T.);
#52187=EDGE_CURVE('',#40886,#40860,#30460,.T.);
#52188=EDGE_CURVE('',#40887,#40888,#9696,.T.);
#52189=EDGE_CURVE('',#40889,#40887,#33538,.T.);
#52190=EDGE_CURVE('',#40870,#40889,#33539,.T.);
#52191=EDGE_CURVE('',#40888,#40874,#33540,.T.);
#52192=EDGE_CURVE('',#40802,#40873,#33541,.T.);
#52193=EDGE_CURVE('',#40872,#40890,#33542,.T.);
#52194=EDGE_CURVE('',#40888,#40890,#30461,.T.);
#52195=EDGE_CURVE('',#40809,#40782,#30462,.T.);
#52196=EDGE_CURVE('',#40850,#40891,#30463,.T.);
#52197=EDGE_CURVE('',#40891,#40892,#9697,.T.);
#52198=EDGE_CURVE('',#40851,#40892,#30464,.T.);
#52199=EDGE_CURVE('',#40893,#40868,#30465,.T.);
#52200=EDGE_CURVE('',#40894,#40893,#30466,.T.);
#52201=EDGE_CURVE('',#40894,#40895,#30467,.T.);
#52202=EDGE_CURVE('',#40895,#40869,#30468,.T.);
#52203=EDGE_CURVE('',#40896,#40850,#30469,.T.);
#52204=EDGE_CURVE('',#40795,#40841,#9698,.T.);
#52205=EDGE_CURVE('',#40896,#40799,#30470,.F.);
#52206=EDGE_CURVE('',#40805,#40891,#30471,.T.);
#52207=EDGE_CURVE('',#40806,#40896,#30472,.T.);
#52208=EDGE_CURVE('',#40892,#40804,#30473,.T.);
#52209=EDGE_CURVE('',#40851,#40808,#30474,.T.);
#52210=EDGE_CURVE('',#40800,#40807,#30475,.F.);
#52211=EDGE_CURVE('',#40842,#40798,#9699,.T.);
#52212=EDGE_CURVE('',#40868,#40790,#9700,.T.);
#52213=EDGE_CURVE('',#40897,#40812,#30476,.T.);
#52214=EDGE_CURVE('',#40897,#40893,#30477,.T.);
#52215=EDGE_CURVE('',#40787,#40869,#9701,.T.);
#52216=EDGE_CURVE('',#40898,#40895,#30478,.T.);
#52217=EDGE_CURVE('',#40898,#40811,#30479,.T.);
#52218=EDGE_CURVE('',#40899,#40900,#33543,.T.);
#52219=EDGE_CURVE('',#40899,#40901,#9702,.T.);
#52220=EDGE_CURVE('',#40901,#40901,#33544,.T.);
#52221=EDGE_CURVE('',#40900,#40899,#33545,.T.);
#52222=EDGE_CURVE('',#40900,#40902,#9703,.T.);
#52223=EDGE_CURVE('',#40902,#40902,#33546,.T.);
#52224=EDGE_CURVE('',#40903,#40903,#33547,.T.);
#52225=EDGE_CURVE('',#40903,#40904,#9704,.T.);
#52226=EDGE_CURVE('',#40904,#40904,#33548,.T.);
#52227=EDGE_CURVE('',#40904,#40905,#9705,.T.);
#52228=EDGE_CURVE('',#40905,#40905,#33549,.T.);
#52229=EDGE_CURVE('',#40838,#40864,#30480,.T.);
#52230=EDGE_CURVE('',#40865,#40906,#30481,.T.);
#52231=EDGE_CURVE('',#40906,#40907,#30482,.T.);
#52232=EDGE_CURVE('',#40907,#40774,#30483,.T.);
#52233=EDGE_CURVE('',#40908,#40887,#30484,.T.);
#52234=EDGE_CURVE('',#40908,#40871,#33550,.T.);
#52235=EDGE_CURVE('',#40889,#40753,#33551,.T.);
#52236=EDGE_CURVE('',#40908,#40890,#9706,.T.);
#74337=ORIENTED_EDGE('',*,*,#52001,.F.);
#74338=ORIENTED_EDGE('',*,*,#52002,.T.);
#74339=ORIENTED_EDGE('',*,*,#52003,.T.);
#74340=ORIENTED_EDGE('',*,*,#52004,.T.);
#74341=ORIENTED_EDGE('',*,*,#52005,.T.);
#74342=ORIENTED_EDGE('',*,*,#52003,.F.);
#74343=ORIENTED_EDGE('',*,*,#52006,.T.);
#74344=ORIENTED_EDGE('',*,*,#52007,.T.);
#74345=ORIENTED_EDGE('',*,*,#52008,.T.);
#74346=ORIENTED_EDGE('',*,*,#52009,.T.);
#74347=ORIENTED_EDGE('',*,*,#52010,.T.);
#74348=ORIENTED_EDGE('',*,*,#52011,.T.);
#74349=ORIENTED_EDGE('',*,*,#52012,.T.);
#74350=ORIENTED_EDGE('',*,*,#52013,.F.);
#74351=ORIENTED_EDGE('',*,*,#52014,.T.);
#74352=ORIENTED_EDGE('',*,*,#52001,.T.);
#74353=ORIENTED_EDGE('',*,*,#52015,.T.);
#74354=ORIENTED_EDGE('',*,*,#52016,.F.);
#74355=ORIENTED_EDGE('',*,*,#52017,.T.);
#74356=ORIENTED_EDGE('',*,*,#52013,.T.);
#74357=ORIENTED_EDGE('',*,*,#52018,.T.);
#74358=ORIENTED_EDGE('',*,*,#52019,.F.);
#74359=ORIENTED_EDGE('',*,*,#52020,.T.);
#74360=ORIENTED_EDGE('',*,*,#52021,.T.);
#74361=ORIENTED_EDGE('',*,*,#52016,.T.);
#74362=ORIENTED_EDGE('',*,*,#52022,.T.);
#74363=ORIENTED_EDGE('',*,*,#52023,.F.);
#74364=ORIENTED_EDGE('',*,*,#52024,.T.);
#74365=ORIENTED_EDGE('',*,*,#52019,.T.);
#74366=ORIENTED_EDGE('',*,*,#52025,.T.);
#74367=ORIENTED_EDGE('',*,*,#52026,.T.);
#74368=ORIENTED_EDGE('',*,*,#52027,.F.);
#74369=ORIENTED_EDGE('',*,*,#52028,.T.);
#74370=ORIENTED_EDGE('',*,*,#52023,.T.);
#74371=ORIENTED_EDGE('',*,*,#52029,.T.);
#74372=ORIENTED_EDGE('',*,*,#52030,.F.);
#74373=ORIENTED_EDGE('',*,*,#52031,.T.);
#74374=ORIENTED_EDGE('',*,*,#52027,.T.);
#74375=ORIENTED_EDGE('',*,*,#52032,.T.);
#74376=ORIENTED_EDGE('',*,*,#52033,.F.);
#74377=ORIENTED_EDGE('',*,*,#52034,.T.);
#74378=ORIENTED_EDGE('',*,*,#52035,.T.);
#74379=ORIENTED_EDGE('',*,*,#52030,.T.);
#74380=ORIENTED_EDGE('',*,*,#52036,.T.);
#74381=ORIENTED_EDGE('',*,*,#52037,.F.);
#74382=ORIENTED_EDGE('',*,*,#52038,.T.);
#74383=ORIENTED_EDGE('',*,*,#52039,.F.);
#74384=ORIENTED_EDGE('',*,*,#52040,.F.);
#74385=ORIENTED_EDGE('',*,*,#52041,.T.);
#74386=ORIENTED_EDGE('',*,*,#52037,.T.);
#74387=ORIENTED_EDGE('',*,*,#52042,.F.);
#74388=ORIENTED_EDGE('',*,*,#52043,.T.);
#74389=ORIENTED_EDGE('',*,*,#52044,.T.);
#74390=ORIENTED_EDGE('',*,*,#52045,.T.);
#74391=ORIENTED_EDGE('',*,*,#52046,.F.);
#74392=ORIENTED_EDGE('',*,*,#52047,.T.);
#74393=ORIENTED_EDGE('',*,*,#52048,.T.);
#74394=ORIENTED_EDGE('',*,*,#52040,.T.);
#74395=ORIENTED_EDGE('',*,*,#52049,.T.);
#74396=ORIENTED_EDGE('',*,*,#52050,.F.);
#74397=ORIENTED_EDGE('',*,*,#52051,.T.);
#74398=ORIENTED_EDGE('',*,*,#52046,.T.);
#74399=ORIENTED_EDGE('',*,*,#52052,.T.);
#74400=ORIENTED_EDGE('',*,*,#52053,.T.);
#74401=ORIENTED_EDGE('',*,*,#52054,.F.);
#74402=ORIENTED_EDGE('',*,*,#52055,.T.);
#74403=ORIENTED_EDGE('',*,*,#52050,.T.);
#74404=ORIENTED_EDGE('',*,*,#52056,.T.);
#74405=ORIENTED_EDGE('',*,*,#52057,.F.);
#74406=ORIENTED_EDGE('',*,*,#52058,.T.);
#74407=ORIENTED_EDGE('',*,*,#52059,.T.);
#74408=ORIENTED_EDGE('',*,*,#52054,.T.);
#74409=ORIENTED_EDGE('',*,*,#52060,.T.);
#74410=ORIENTED_EDGE('',*,*,#52061,.F.);
#74411=ORIENTED_EDGE('',*,*,#52062,.T.);
#74412=ORIENTED_EDGE('',*,*,#52057,.T.);
#74413=ORIENTED_EDGE('',*,*,#52063,.T.);
#74414=ORIENTED_EDGE('',*,*,#52064,.T.);
#74415=ORIENTED_EDGE('',*,*,#52065,.F.);
#74416=ORIENTED_EDGE('',*,*,#52066,.T.);
#74417=ORIENTED_EDGE('',*,*,#52061,.T.);
#74418=ORIENTED_EDGE('',*,*,#52067,.T.);
#74419=ORIENTED_EDGE('',*,*,#52068,.T.);
#74420=ORIENTED_EDGE('',*,*,#52069,.T.);
#74421=ORIENTED_EDGE('',*,*,#52070,.T.);
#74422=ORIENTED_EDGE('',*,*,#52071,.T.);
#74423=ORIENTED_EDGE('',*,*,#52072,.F.);
#74424=ORIENTED_EDGE('',*,*,#52073,.T.);
#74425=ORIENTED_EDGE('',*,*,#52074,.T.);
#74426=ORIENTED_EDGE('',*,*,#52075,.T.);
#74427=ORIENTED_EDGE('',*,*,#52076,.T.);
#74428=ORIENTED_EDGE('',*,*,#52070,.F.);
#74429=ORIENTED_EDGE('',*,*,#52077,.F.);
#74430=ORIENTED_EDGE('',*,*,#52039,.T.);
#74431=ORIENTED_EDGE('',*,*,#52078,.F.);
#74432=ORIENTED_EDGE('',*,*,#52079,.F.);
#74433=ORIENTED_EDGE('',*,*,#52080,.F.);
#74434=ORIENTED_EDGE('',*,*,#52081,.T.);
#74435=ORIENTED_EDGE('',*,*,#52082,.F.);
#74436=ORIENTED_EDGE('',*,*,#52083,.F.);
#74437=ORIENTED_EDGE('',*,*,#52084,.F.);
#74438=ORIENTED_EDGE('',*,*,#52085,.F.);
#74439=ORIENTED_EDGE('',*,*,#52086,.T.);
#74440=ORIENTED_EDGE('',*,*,#52087,.T.);
#74441=ORIENTED_EDGE('',*,*,#52088,.F.);
#74442=ORIENTED_EDGE('',*,*,#52089,.F.);
#74443=ORIENTED_EDGE('',*,*,#52082,.T.);
#74444=ORIENTED_EDGE('',*,*,#52090,.F.);
#74445=ORIENTED_EDGE('',*,*,#52091,.F.);
#74446=ORIENTED_EDGE('',*,*,#52088,.T.);
#74447=ORIENTED_EDGE('',*,*,#52092,.T.);
#74448=ORIENTED_EDGE('',*,*,#52093,.F.);
#74449=ORIENTED_EDGE('',*,*,#52094,.F.);
#74450=ORIENTED_EDGE('',*,*,#52090,.T.);
#74451=ORIENTED_EDGE('',*,*,#52095,.T.);
#74452=ORIENTED_EDGE('',*,*,#52096,.F.);
#74453=ORIENTED_EDGE('',*,*,#52097,.F.);
#74454=ORIENTED_EDGE('',*,*,#52098,.F.);
#74455=ORIENTED_EDGE('',*,*,#52099,.F.);
#74456=ORIENTED_EDGE('',*,*,#52100,.T.);
#74457=ORIENTED_EDGE('',*,*,#52101,.T.);
#74458=ORIENTED_EDGE('',*,*,#52102,.F.);
#74459=ORIENTED_EDGE('',*,*,#52103,.F.);
#74460=ORIENTED_EDGE('',*,*,#52096,.T.);
#74461=ORIENTED_EDGE('',*,*,#52104,.F.);
#74462=ORIENTED_EDGE('',*,*,#52105,.F.);
#74463=ORIENTED_EDGE('',*,*,#52102,.T.);
#74464=ORIENTED_EDGE('',*,*,#52106,.T.);
#74465=ORIENTED_EDGE('',*,*,#52107,.F.);
#74466=ORIENTED_EDGE('',*,*,#52108,.F.);
#74467=ORIENTED_EDGE('',*,*,#52104,.T.);
#74468=ORIENTED_EDGE('',*,*,#52109,.T.);
#74469=ORIENTED_EDGE('',*,*,#52110,.F.);
#74470=ORIENTED_EDGE('',*,*,#52111,.F.);
#74471=ORIENTED_EDGE('',*,*,#52112,.F.);
#74472=ORIENTED_EDGE('',*,*,#52113,.F.);
#74473=ORIENTED_EDGE('',*,*,#52114,.F.);
#74474=ORIENTED_EDGE('',*,*,#52115,.T.);
#74475=ORIENTED_EDGE('',*,*,#52116,.T.);
#74476=ORIENTED_EDGE('',*,*,#52117,.F.);
#74477=ORIENTED_EDGE('',*,*,#52118,.F.);
#74478=ORIENTED_EDGE('',*,*,#52119,.T.);
#74479=ORIENTED_EDGE('',*,*,#52114,.T.);
#74480=ORIENTED_EDGE('',*,*,#52120,.F.);
#74481=ORIENTED_EDGE('',*,*,#52121,.F.);
#74482=ORIENTED_EDGE('',*,*,#52122,.T.);
#74483=ORIENTED_EDGE('',*,*,#52118,.T.);
#74484=ORIENTED_EDGE('',*,*,#52123,.F.);
#74485=ORIENTED_EDGE('',*,*,#52124,.F.);
#74486=ORIENTED_EDGE('',*,*,#52125,.T.);
#74487=ORIENTED_EDGE('',*,*,#52126,.T.);
#74488=ORIENTED_EDGE('',*,*,#52127,.T.);
#74489=ORIENTED_EDGE('',*,*,#52128,.F.);
#74490=ORIENTED_EDGE('',*,*,#52129,.F.);
#74491=ORIENTED_EDGE('',*,*,#52130,.F.);
#74492=ORIENTED_EDGE('',*,*,#52131,.T.);
#74493=ORIENTED_EDGE('',*,*,#52124,.T.);
#74494=ORIENTED_EDGE('',*,*,#52132,.F.);
#74495=ORIENTED_EDGE('',*,*,#52133,.T.);
#74496=ORIENTED_EDGE('',*,*,#52130,.T.);
#74497=ORIENTED_EDGE('',*,*,#52134,.F.);
#74498=ORIENTED_EDGE('',*,*,#52135,.F.);
#74499=ORIENTED_EDGE('',*,*,#52136,.T.);
#74500=ORIENTED_EDGE('',*,*,#52132,.T.);
#74501=ORIENTED_EDGE('',*,*,#52137,.F.);
#74502=ORIENTED_EDGE('',*,*,#52138,.F.);
#74503=ORIENTED_EDGE('',*,*,#52139,.T.);
#74504=ORIENTED_EDGE('',*,*,#52140,.T.);
#74505=ORIENTED_EDGE('',*,*,#52141,.F.);
#74506=ORIENTED_EDGE('',*,*,#52142,.F.);
#74507=ORIENTED_EDGE('',*,*,#52143,.F.);
#74508=ORIENTED_EDGE('',*,*,#52144,.T.);
#74509=ORIENTED_EDGE('',*,*,#52138,.T.);
#74510=ORIENTED_EDGE('',*,*,#52145,.T.);
#74511=ORIENTED_EDGE('',*,*,#52146,.T.);
#74512=ORIENTED_EDGE('',*,*,#52147,.F.);
#74513=ORIENTED_EDGE('',*,*,#52148,.T.);
#74514=ORIENTED_EDGE('',*,*,#52149,.T.);
#74515=ORIENTED_EDGE('',*,*,#52148,.F.);
#74516=ORIENTED_EDGE('',*,*,#52135,.T.);
#74517=ORIENTED_EDGE('',*,*,#52150,.F.);
#74518=ORIENTED_EDGE('',*,*,#52116,.F.);
#74519=ORIENTED_EDGE('',*,*,#52151,.T.);
#74520=ORIENTED_EDGE('',*,*,#52121,.T.);
#74521=ORIENTED_EDGE('',*,*,#52152,.F.);
#74522=ORIENTED_EDGE('',*,*,#52153,.F.);
#74523=ORIENTED_EDGE('',*,*,#52154,.T.);
#74524=ORIENTED_EDGE('',*,*,#52155,.T.);
#74525=ORIENTED_EDGE('',*,*,#52156,.T.);
#74526=ORIENTED_EDGE('',*,*,#52157,.T.);
#74527=ORIENTED_EDGE('',*,*,#52158,.T.);
#74528=ORIENTED_EDGE('',*,*,#52159,.F.);
#74529=ORIENTED_EDGE('',*,*,#52110,.T.);
#74530=ORIENTED_EDGE('',*,*,#52160,.F.);
#74531=ORIENTED_EDGE('',*,*,#52161,.T.);
#74532=ORIENTED_EDGE('',*,*,#52162,.T.);
#74533=ORIENTED_EDGE('',*,*,#52099,.T.);
#74534=ORIENTED_EDGE('',*,*,#52163,.F.);
#74535=ORIENTED_EDGE('',*,*,#52164,.F.);
#74536=ORIENTED_EDGE('',*,*,#52107,.T.);
#74537=ORIENTED_EDGE('',*,*,#52165,.T.);
#74538=ORIENTED_EDGE('',*,*,#52166,.T.);
#74539=ORIENTED_EDGE('',*,*,#52085,.T.);
#74540=ORIENTED_EDGE('',*,*,#52167,.F.);
#74541=ORIENTED_EDGE('',*,*,#52168,.F.);
#74542=ORIENTED_EDGE('',*,*,#52093,.T.);
#74543=ORIENTED_EDGE('',*,*,#52169,.T.);
#74544=ORIENTED_EDGE('',*,*,#52170,.T.);
#74545=ORIENTED_EDGE('',*,*,#52171,.T.);
#74546=ORIENTED_EDGE('',*,*,#52172,.F.);
#74547=ORIENTED_EDGE('',*,*,#52173,.F.);
#74548=ORIENTED_EDGE('',*,*,#52174,.T.);
#74549=ORIENTED_EDGE('',*,*,#52175,.T.);
#74550=ORIENTED_EDGE('',*,*,#52176,.F.);
#74551=ORIENTED_EDGE('',*,*,#52171,.F.);
#74552=ORIENTED_EDGE('',*,*,#52100,.F.);
#74553=ORIENTED_EDGE('',*,*,#52177,.F.);
#74554=ORIENTED_EDGE('',*,*,#52178,.F.);
#74555=ORIENTED_EDGE('',*,*,#52036,.F.);
#74556=ORIENTED_EDGE('',*,*,#52032,.F.);
#74557=ORIENTED_EDGE('',*,*,#52029,.F.);
#74558=ORIENTED_EDGE('',*,*,#52026,.F.);
#74559=ORIENTED_EDGE('',*,*,#52179,.T.);
#74560=ORIENTED_EDGE('',*,*,#52166,.F.);
#74561=ORIENTED_EDGE('',*,*,#52165,.F.);
#74562=ORIENTED_EDGE('',*,*,#52109,.F.);
#74563=ORIENTED_EDGE('',*,*,#52106,.F.);
#74564=ORIENTED_EDGE('',*,*,#52101,.F.);
#74565=ORIENTED_EDGE('',*,*,#52086,.F.);
#74566=ORIENTED_EDGE('',*,*,#52179,.F.);
#74567=ORIENTED_EDGE('',*,*,#52025,.F.);
#74568=ORIENTED_EDGE('',*,*,#52022,.F.);
#74569=ORIENTED_EDGE('',*,*,#52018,.F.);
#74570=ORIENTED_EDGE('',*,*,#52015,.F.);
#74571=ORIENTED_EDGE('',*,*,#52012,.F.);
#74572=ORIENTED_EDGE('',*,*,#52180,.T.);
#74573=ORIENTED_EDGE('',*,*,#52170,.F.);
#74574=ORIENTED_EDGE('',*,*,#52169,.F.);
#74575=ORIENTED_EDGE('',*,*,#52095,.F.);
#74576=ORIENTED_EDGE('',*,*,#52092,.F.);
#74577=ORIENTED_EDGE('',*,*,#52087,.F.);
#74578=ORIENTED_EDGE('',*,*,#52181,.T.);
#74579=ORIENTED_EDGE('',*,*,#52174,.F.);
#74580=ORIENTED_EDGE('',*,*,#52180,.F.);
#74581=ORIENTED_EDGE('',*,*,#52011,.F.);
#74582=ORIENTED_EDGE('',*,*,#52010,.F.);
#74583=ORIENTED_EDGE('',*,*,#52009,.F.);
#74584=ORIENTED_EDGE('',*,*,#52182,.F.);
#74585=ORIENTED_EDGE('',*,*,#52175,.F.);
#74586=ORIENTED_EDGE('',*,*,#52181,.F.);
#74587=ORIENTED_EDGE('',*,*,#52007,.F.);
#74588=ORIENTED_EDGE('',*,*,#52183,.F.);
#74589=ORIENTED_EDGE('',*,*,#52176,.T.);
#74590=ORIENTED_EDGE('',*,*,#52182,.T.);
#74591=ORIENTED_EDGE('',*,*,#52008,.F.);
#74592=ORIENTED_EDGE('',*,*,#52021,.F.);
#74593=ORIENTED_EDGE('',*,*,#52184,.F.);
#74594=ORIENTED_EDGE('',*,*,#52084,.T.);
#74595=ORIENTED_EDGE('',*,*,#52083,.T.);
#74596=ORIENTED_EDGE('',*,*,#52089,.T.);
#74597=ORIENTED_EDGE('',*,*,#52091,.T.);
#74598=ORIENTED_EDGE('',*,*,#52094,.T.);
#74599=ORIENTED_EDGE('',*,*,#52173,.T.);
#74600=ORIENTED_EDGE('',*,*,#52172,.T.);
#74601=ORIENTED_EDGE('',*,*,#52183,.T.);
#74602=ORIENTED_EDGE('',*,*,#52006,.F.);
#74603=ORIENTED_EDGE('',*,*,#52002,.F.);
#74604=ORIENTED_EDGE('',*,*,#52014,.F.);
#74605=ORIENTED_EDGE('',*,*,#52017,.F.);
#74606=ORIENTED_EDGE('',*,*,#52035,.F.);
#74607=ORIENTED_EDGE('',*,*,#52185,.F.);
#74608=ORIENTED_EDGE('',*,*,#52098,.T.);
#74609=ORIENTED_EDGE('',*,*,#52097,.T.);
#74610=ORIENTED_EDGE('',*,*,#52103,.T.);
#74611=ORIENTED_EDGE('',*,*,#52105,.T.);
#74612=ORIENTED_EDGE('',*,*,#52108,.T.);
#74613=ORIENTED_EDGE('',*,*,#52168,.T.);
#74614=ORIENTED_EDGE('',*,*,#52167,.T.);
#74615=ORIENTED_EDGE('',*,*,#52184,.T.);
#74616=ORIENTED_EDGE('',*,*,#52020,.F.);
#74617=ORIENTED_EDGE('',*,*,#52024,.F.);
#74618=ORIENTED_EDGE('',*,*,#52028,.F.);
#74619=ORIENTED_EDGE('',*,*,#52031,.F.);
#74620=ORIENTED_EDGE('',*,*,#52177,.T.);
#74621=ORIENTED_EDGE('',*,*,#52162,.F.);
#74622=ORIENTED_EDGE('',*,*,#52161,.F.);
#74623=ORIENTED_EDGE('',*,*,#52186,.F.);
#74624=ORIENTED_EDGE('',*,*,#52142,.T.);
#74625=ORIENTED_EDGE('',*,*,#52141,.T.);
#74626=ORIENTED_EDGE('',*,*,#52140,.F.);
#74627=ORIENTED_EDGE('',*,*,#52187,.F.);
#74628=ORIENTED_EDGE('',*,*,#52188,.F.);
#74629=ORIENTED_EDGE('',*,*,#52189,.F.);
#74630=ORIENTED_EDGE('',*,*,#52190,.F.);
#74631=ORIENTED_EDGE('',*,*,#52159,.T.);
#74632=ORIENTED_EDGE('',*,*,#52191,.F.);
#74633=ORIENTED_EDGE('',*,*,#52068,.F.);
#74634=ORIENTED_EDGE('',*,*,#52069,.F.);
#74635=ORIENTED_EDGE('',*,*,#52192,.T.);
#74636=ORIENTED_EDGE('',*,*,#52157,.F.);
#74637=ORIENTED_EDGE('',*,*,#52193,.T.);
#74638=ORIENTED_EDGE('',*,*,#52194,.F.);
#74639=ORIENTED_EDGE('',*,*,#52191,.T.);
#74640=ORIENTED_EDGE('',*,*,#52158,.F.);
#74641=ORIENTED_EDGE('',*,*,#52192,.F.);
#74642=ORIENTED_EDGE('',*,*,#52077,.T.);
#74643=ORIENTED_EDGE('',*,*,#52195,.T.);
#74644=ORIENTED_EDGE('',*,*,#52042,.T.);
#74645=ORIENTED_EDGE('',*,*,#52196,.T.);
#74646=ORIENTED_EDGE('',*,*,#52197,.T.);
#74647=ORIENTED_EDGE('',*,*,#52198,.F.);
#74648=ORIENTED_EDGE('',*,*,#52127,.F.);
#74649=ORIENTED_EDGE('',*,*,#52199,.F.);
#74650=ORIENTED_EDGE('',*,*,#52200,.F.);
#74651=ORIENTED_EDGE('',*,*,#52201,.T.);
#74652=ORIENTED_EDGE('',*,*,#52202,.T.);
#74653=ORIENTED_EDGE('',*,*,#52153,.T.);
#74654=ORIENTED_EDGE('',*,*,#52203,.T.);
#74655=ORIENTED_EDGE('',*,*,#52126,.F.);
#74656=ORIENTED_EDGE('',*,*,#52125,.F.);
#74657=ORIENTED_EDGE('',*,*,#52131,.F.);
#74658=ORIENTED_EDGE('',*,*,#52133,.F.);
#74659=ORIENTED_EDGE('',*,*,#52136,.F.);
#74660=ORIENTED_EDGE('',*,*,#52151,.F.);
#74661=ORIENTED_EDGE('',*,*,#52204,.F.);
#74662=ORIENTED_EDGE('',*,*,#52058,.F.);
#74663=ORIENTED_EDGE('',*,*,#52062,.F.);
#74664=ORIENTED_EDGE('',*,*,#52066,.F.);
#74665=ORIENTED_EDGE('',*,*,#52205,.F.);
#74666=ORIENTED_EDGE('',*,*,#52073,.F.);
#74667=ORIENTED_EDGE('',*,*,#52206,.T.);
#74668=ORIENTED_EDGE('',*,*,#52196,.F.);
#74669=ORIENTED_EDGE('',*,*,#52203,.F.);
#74670=ORIENTED_EDGE('',*,*,#52207,.F.);
#74671=ORIENTED_EDGE('',*,*,#52072,.T.);
#74672=ORIENTED_EDGE('',*,*,#52208,.F.);
#74673=ORIENTED_EDGE('',*,*,#52197,.F.);
#74674=ORIENTED_EDGE('',*,*,#52206,.F.);
#74675=ORIENTED_EDGE('',*,*,#52209,.F.);
#74676=ORIENTED_EDGE('',*,*,#52198,.T.);
#74677=ORIENTED_EDGE('',*,*,#52208,.T.);
#74678=ORIENTED_EDGE('',*,*,#52071,.F.);
#74679=ORIENTED_EDGE('',*,*,#52076,.F.);
#74680=ORIENTED_EDGE('',*,*,#52128,.T.);
#74681=ORIENTED_EDGE('',*,*,#52209,.T.);
#74682=ORIENTED_EDGE('',*,*,#52075,.F.);
#74683=ORIENTED_EDGE('',*,*,#52210,.F.);
#74684=ORIENTED_EDGE('',*,*,#52067,.F.);
#74685=ORIENTED_EDGE('',*,*,#52064,.F.);
#74686=ORIENTED_EDGE('',*,*,#52211,.F.);
#74687=ORIENTED_EDGE('',*,*,#52150,.T.);
#74688=ORIENTED_EDGE('',*,*,#52137,.T.);
#74689=ORIENTED_EDGE('',*,*,#52134,.T.);
#74690=ORIENTED_EDGE('',*,*,#52129,.T.);
#74691=ORIENTED_EDGE('',*,*,#52053,.F.);
#74692=ORIENTED_EDGE('',*,*,#52212,.F.);
#74693=ORIENTED_EDGE('',*,*,#52152,.T.);
#74694=ORIENTED_EDGE('',*,*,#52123,.T.);
#74695=ORIENTED_EDGE('',*,*,#52120,.T.);
#74696=ORIENTED_EDGE('',*,*,#52117,.T.);
#74697=ORIENTED_EDGE('',*,*,#52211,.T.);
#74698=ORIENTED_EDGE('',*,*,#52063,.F.);
#74699=ORIENTED_EDGE('',*,*,#52060,.F.);
#74700=ORIENTED_EDGE('',*,*,#52056,.F.);
#74701=ORIENTED_EDGE('',*,*,#52044,.F.);
#74702=ORIENTED_EDGE('',*,*,#52043,.F.);
#74703=ORIENTED_EDGE('',*,*,#52195,.F.);
#74704=ORIENTED_EDGE('',*,*,#52081,.F.);
#74705=ORIENTED_EDGE('',*,*,#52213,.F.);
#74706=ORIENTED_EDGE('',*,*,#52214,.T.);
#74707=ORIENTED_EDGE('',*,*,#52199,.T.);
#74708=ORIENTED_EDGE('',*,*,#52212,.T.);
#74709=ORIENTED_EDGE('',*,*,#52052,.F.);
#74710=ORIENTED_EDGE('',*,*,#52049,.F.);
#74711=ORIENTED_EDGE('',*,*,#52045,.F.);
#74712=ORIENTED_EDGE('',*,*,#52074,.F.);
#74713=ORIENTED_EDGE('',*,*,#52207,.T.);
#74714=ORIENTED_EDGE('',*,*,#52205,.T.);
#74715=ORIENTED_EDGE('',*,*,#52065,.T.);
#74716=ORIENTED_EDGE('',*,*,#52210,.T.);
#74717=ORIENTED_EDGE('',*,*,#52059,.F.);
#74718=ORIENTED_EDGE('',*,*,#52204,.T.);
#74719=ORIENTED_EDGE('',*,*,#52115,.F.);
#74720=ORIENTED_EDGE('',*,*,#52119,.F.);
#74721=ORIENTED_EDGE('',*,*,#52122,.F.);
#74722=ORIENTED_EDGE('',*,*,#52154,.F.);
#74723=ORIENTED_EDGE('',*,*,#52215,.F.);
#74724=ORIENTED_EDGE('',*,*,#52047,.F.);
#74725=ORIENTED_EDGE('',*,*,#52051,.F.);
#74726=ORIENTED_EDGE('',*,*,#52055,.F.);
#74727=ORIENTED_EDGE('',*,*,#52202,.F.);
#74728=ORIENTED_EDGE('',*,*,#52216,.F.);
#74729=ORIENTED_EDGE('',*,*,#52217,.T.);
#74730=ORIENTED_EDGE('',*,*,#52079,.T.);
#74731=ORIENTED_EDGE('',*,*,#52078,.T.);
#74732=ORIENTED_EDGE('',*,*,#52038,.F.);
#74733=ORIENTED_EDGE('',*,*,#52041,.F.);
#74734=ORIENTED_EDGE('',*,*,#52048,.F.);
#74735=ORIENTED_EDGE('',*,*,#52215,.T.);
#74736=ORIENTED_EDGE('',*,*,#52218,.F.);
#74737=ORIENTED_EDGE('',*,*,#52219,.T.);
#74738=ORIENTED_EDGE('',*,*,#52220,.T.);
#74739=ORIENTED_EDGE('',*,*,#52219,.F.);
#74740=ORIENTED_EDGE('',*,*,#52221,.F.);
#74741=ORIENTED_EDGE('',*,*,#52218,.T.);
#74742=ORIENTED_EDGE('',*,*,#52222,.T.);
#74743=ORIENTED_EDGE('',*,*,#52223,.F.);
#74744=ORIENTED_EDGE('',*,*,#52222,.F.);
#74745=ORIENTED_EDGE('',*,*,#52221,.T.);
#74746=ORIENTED_EDGE('',*,*,#52214,.F.);
#74747=ORIENTED_EDGE('',*,*,#52213,.T.);
#74748=ORIENTED_EDGE('',*,*,#52080,.T.);
#74749=ORIENTED_EDGE('',*,*,#52217,.F.);
#74750=ORIENTED_EDGE('',*,*,#52216,.T.);
#74751=ORIENTED_EDGE('',*,*,#52201,.F.);
#74752=ORIENTED_EDGE('',*,*,#52200,.T.);
#74753=ORIENTED_EDGE('',*,*,#52223,.T.);
#74754=ORIENTED_EDGE('',*,*,#52220,.F.);
#74755=ORIENTED_EDGE('',*,*,#52149,.F.);
#74756=ORIENTED_EDGE('',*,*,#52224,.T.);
#74757=ORIENTED_EDGE('',*,*,#52147,.T.);
#74758=ORIENTED_EDGE('',*,*,#52224,.F.);
#74759=ORIENTED_EDGE('',*,*,#52225,.T.);
#74760=ORIENTED_EDGE('',*,*,#52226,.F.);
#74761=ORIENTED_EDGE('',*,*,#52225,.F.);
#74762=ORIENTED_EDGE('',*,*,#52226,.T.);
#74763=ORIENTED_EDGE('',*,*,#52227,.T.);
#74764=ORIENTED_EDGE('',*,*,#52228,.F.);
#74765=ORIENTED_EDGE('',*,*,#52227,.F.);
#74766=ORIENTED_EDGE('',*,*,#52160,.T.);
#74767=ORIENTED_EDGE('',*,*,#52113,.T.);
#74768=ORIENTED_EDGE('',*,*,#52229,.T.);
#74769=ORIENTED_EDGE('',*,*,#52143,.T.);
#74770=ORIENTED_EDGE('',*,*,#52186,.T.);
#74771=ORIENTED_EDGE('',*,*,#52228,.T.);
#74772=ORIENTED_EDGE('',*,*,#52033,.T.);
#74773=ORIENTED_EDGE('',*,*,#52178,.T.);
#74774=ORIENTED_EDGE('',*,*,#52187,.T.);
#74775=ORIENTED_EDGE('',*,*,#52139,.F.);
#74776=ORIENTED_EDGE('',*,*,#52146,.F.);
#74777=ORIENTED_EDGE('',*,*,#52230,.T.);
#74778=ORIENTED_EDGE('',*,*,#52231,.T.);
#74779=ORIENTED_EDGE('',*,*,#52232,.T.);
#74780=ORIENTED_EDGE('',*,*,#52230,.F.);
#74781=ORIENTED_EDGE('',*,*,#52145,.F.);
#74782=ORIENTED_EDGE('',*,*,#52144,.F.);
#74783=ORIENTED_EDGE('',*,*,#52229,.F.);
#74784=ORIENTED_EDGE('',*,*,#52112,.T.);
#74785=ORIENTED_EDGE('',*,*,#52111,.T.);
#74786=ORIENTED_EDGE('',*,*,#52164,.T.);
#74787=ORIENTED_EDGE('',*,*,#52163,.T.);
#74788=ORIENTED_EDGE('',*,*,#52185,.T.);
#74789=ORIENTED_EDGE('',*,*,#52034,.F.);
#74790=ORIENTED_EDGE('',*,*,#52232,.F.);
#74791=ORIENTED_EDGE('',*,*,#52231,.F.);
#74792=ORIENTED_EDGE('',*,*,#52233,.F.);
#74793=ORIENTED_EDGE('',*,*,#52234,.T.);
#74794=ORIENTED_EDGE('',*,*,#52155,.F.);
#74795=ORIENTED_EDGE('',*,*,#52190,.T.);
#74796=ORIENTED_EDGE('',*,*,#52235,.T.);
#74797=ORIENTED_EDGE('',*,*,#52004,.F.);
#74798=ORIENTED_EDGE('',*,*,#52005,.F.);
#74799=ORIENTED_EDGE('',*,*,#52235,.F.);
#74800=ORIENTED_EDGE('',*,*,#52189,.T.);
#74801=ORIENTED_EDGE('',*,*,#52156,.F.);
#74802=ORIENTED_EDGE('',*,*,#52234,.F.);
#74803=ORIENTED_EDGE('',*,*,#52236,.T.);
#74804=ORIENTED_EDGE('',*,*,#52193,.F.);
#74805=ORIENTED_EDGE('',*,*,#52236,.F.);
#74806=ORIENTED_EDGE('',*,*,#52233,.T.);
#74807=ORIENTED_EDGE('',*,*,#52188,.T.);
#74808=ORIENTED_EDGE('',*,*,#52194,.T.);
#75299=SPHERICAL_SURFACE('',#86032,68.);
#75300=SPHERICAL_SURFACE('',#86054,67.);
#79158=ADVANCED_FACE('',(#23728),#2299,.T.);
#79159=ADVANCED_FACE('',(#23729),#2300,.T.);
#79160=ADVANCED_FACE('',(#23730),#2301,.T.);
#79161=ADVANCED_FACE('',(#23731),#2302,.T.);
#79162=ADVANCED_FACE('',(#23732),#2303,.T.);
#79163=ADVANCED_FACE('',(#23733),#2304,.T.);
#79164=ADVANCED_FACE('',(#23734),#2305,.T.);
#79165=ADVANCED_FACE('',(#23735),#2306,.T.);
#79166=ADVANCED_FACE('',(#23736),#2307,.T.);
#79167=ADVANCED_FACE('',(#23737),#2308,.T.);
#79168=ADVANCED_FACE('',(#23738),#2309,.T.);
#79169=ADVANCED_FACE('',(#23739),#2310,.T.);
#79170=ADVANCED_FACE('',(#23740),#2311,.T.);
#79171=ADVANCED_FACE('',(#23741),#2312,.T.);
#79172=ADVANCED_FACE('',(#23742),#2313,.T.);
#79173=ADVANCED_FACE('',(#23743),#2314,.T.);
#79174=ADVANCED_FACE('',(#23744),#2315,.T.);
#79175=ADVANCED_FACE('',(#23745),#1963,.T.);
#79176=ADVANCED_FACE('',(#23746),#2316,.T.);
#79177=ADVANCED_FACE('',(#23747),#2317,.T.);
#79178=ADVANCED_FACE('',(#23748),#2318,.T.);
#79179=ADVANCED_FACE('',(#23749),#2319,.T.);
#79180=ADVANCED_FACE('',(#23750),#2320,.T.);
#79181=ADVANCED_FACE('',(#23751),#2321,.T.);
#79182=ADVANCED_FACE('',(#23752),#2322,.T.);
#79183=ADVANCED_FACE('',(#23753),#2323,.T.);
#79184=ADVANCED_FACE('',(#23754),#2324,.T.);
#79185=ADVANCED_FACE('',(#23755),#2325,.T.);
#79186=ADVANCED_FACE('',(#23756),#2326,.T.);
#79187=ADVANCED_FACE('',(#23757),#2327,.T.);
#79188=ADVANCED_FACE('',(#23758),#2328,.T.);
#79189=ADVANCED_FACE('',(#23759),#2329,.T.);
#79190=ADVANCED_FACE('',(#23760),#2330,.T.);
#79191=ADVANCED_FACE('',(#23761),#2331,.T.);
#79192=ADVANCED_FACE('',(#23762),#1964,.T.);
#79193=ADVANCED_FACE('',(#23763),#1965,.T.);
#79194=ADVANCED_FACE('',(#23764),#2332,.F.);
#79195=ADVANCED_FACE('',(#23765),#2333,.T.);
#79196=ADVANCED_FACE('',(#23766),#2334,.T.);
#79197=ADVANCED_FACE('',(#23767),#2335,.T.);
#79198=ADVANCED_FACE('',(#23768),#2336,.T.);
#79199=ADVANCED_FACE('',(#23769),#2337,.T.);
#79200=ADVANCED_FACE('',(#23770),#2338,.T.);
#79201=ADVANCED_FACE('',(#23771),#207,.F.);
#79202=ADVANCED_FACE('',(#23772),#208,.F.);
#79203=ADVANCED_FACE('',(#23773),#209,.F.);
#79204=ADVANCED_FACE('',(#23774),#210,.F.);
#79205=ADVANCED_FACE('',(#23775),#19857,.F.);
#79206=ADVANCED_FACE('',(#23776),#211,.F.);
#79207=ADVANCED_FACE('',(#23777),#212,.F.);
#79208=ADVANCED_FACE('',(#23778),#213,.F.);
#79209=ADVANCED_FACE('',(#23779),#214,.F.);
#79210=ADVANCED_FACE('',(#23780),#19858,.T.);
#79211=ADVANCED_FACE('',(#23781),#75299,.T.);
#79212=ADVANCED_FACE('',(#23782),#1966,.T.);
#79213=ADVANCED_FACE('',(#23783),#215,.F.);
#79214=ADVANCED_FACE('',(#23784),#216,.F.);
#79215=ADVANCED_FACE('',(#23785),#217,.F.);
#79216=ADVANCED_FACE('',(#23786),#218,.F.);
#79217=ADVANCED_FACE('',(#23787),#19859,.F.);
#79218=ADVANCED_FACE('',(#23788),#219,.F.);
#79219=ADVANCED_FACE('',(#23789),#220,.F.);
#79220=ADVANCED_FACE('',(#23790),#221,.F.);
#79221=ADVANCED_FACE('',(#23791),#222,.F.);
#79222=ADVANCED_FACE('',(#23792),#2339,.T.);
#79223=ADVANCED_FACE('',(#23793),#223,.F.);
#79224=ADVANCED_FACE('',(#23794),#224,.F.);
#79225=ADVANCED_FACE('',(#23795),#2340,.F.);
#79226=ADVANCED_FACE('',(#23796),#1967,.F.);
#79227=ADVANCED_FACE('',(#23797,#1721),#19860,.F.);
#79228=ADVANCED_FACE('',(#23798,#1722),#19861,.F.);
#79229=ADVANCED_FACE('',(#23799,#1723),#19862,.T.);
#79230=ADVANCED_FACE('',(#23800),#2341,.F.);
#79231=ADVANCED_FACE('',(#23801),#1968,.F.);
#79232=ADVANCED_FACE('',(#23802,#1724),#19863,.T.);
#79233=ADVANCED_FACE('',(#23803),#2342,.T.);
#79234=ADVANCED_FACE('',(#23804),#225,.F.);
#79235=ADVANCED_FACE('',(#23805),#75300,.T.);
#79236=ADVANCED_FACE('',(#23806),#19864,.T.);
#79237=ADVANCED_FACE('',(#23807),#2343,.T.);
#79334=CLOSED_SHELL('',(#79158,#79159,#79160,#79161,#79162,#79163,#79164,
#79165,#79166,#79167,#79168,#79169,#79170,#79171,#79172,#79173,#79174,#79175,
#79176,#79177,#79178,#79179,#79180,#79181,#79182,#79183,#79184,#79185,#79186,
#79187,#79188,#79189,#79190,#79191,#79192,#79193,#79194,#79195,#79196,#79197,
#79198,#79199,#79200,#79201,#79202,#79203,#79204,#79205,#79206,#79207,#79208,
#79209,#79210,#79211,#79212,#79213,#79214,#79215,#79216,#79217,#79218,#79219,
#79220,#79221,#79222,#79223,#79224,#79225,#79226,#79227,#79228,#79229,#79230,
#79231,#79232,#79233,#79234,#79235,#79236,#79237));
#85967=AXIS2_PLACEMENT_3D('',#203966,#106079,#106080);
#85968=AXIS2_PLACEMENT_3D('',#203967,#106081,#106082);
#85969=AXIS2_PLACEMENT_3D('',#204039,#106085,#106086);
#85970=AXIS2_PLACEMENT_3D('',#204040,#106087,#106088);
#85971=AXIS2_PLACEMENT_3D('',#204138,#106090,#106091);
#85972=AXIS2_PLACEMENT_3D('',#204280,#106093,#106094);
#85973=AXIS2_PLACEMENT_3D('',#204414,#106096,#106097);
#85974=AXIS2_PLACEMENT_3D('',#204551,#106099,#106100);
#85975=AXIS2_PLACEMENT_3D('',#204690,#106102,#106103);
#85976=AXIS2_PLACEMENT_3D('',#204828,#106105,#106106);
#85977=AXIS2_PLACEMENT_3D('',#204964,#106108,#106109);
#85978=AXIS2_PLACEMENT_3D('',#205093,#106111,#106112);
#85979=AXIS2_PLACEMENT_3D('',#205106,#106114,#106115);
#85980=AXIS2_PLACEMENT_3D('',#205107,#106116,#106117);
#85981=AXIS2_PLACEMENT_3D('',#205176,#106119,#106120);
#85982=AXIS2_PLACEMENT_3D('',#205241,#106121,#106122);
#85983=AXIS2_PLACEMENT_3D('',#205384,#106124,#106125);
#85984=AXIS2_PLACEMENT_3D('',#205549,#106127,#106128);
#85985=AXIS2_PLACEMENT_3D('',#205709,#106130,#106131);
#85986=AXIS2_PLACEMENT_3D('',#205876,#106133,#106134);
#85987=AXIS2_PLACEMENT_3D('',#206041,#106136,#106137);
#85988=AXIS2_PLACEMENT_3D('',#206201,#106139,#106140);
#85989=AXIS2_PLACEMENT_3D('',#206204,#106141,#106142);
#85990=AXIS2_PLACEMENT_3D('',#206205,#106143,#106144);
#85991=AXIS2_PLACEMENT_3D('',#206301,#106148,#106149);
#85992=AXIS2_PLACEMENT_3D('',#206357,#106151,#106152);
#85993=AXIS2_PLACEMENT_3D('',#206416,#106153,#106154);
#85994=AXIS2_PLACEMENT_3D('',#206452,#106157,#106158);
#85995=AXIS2_PLACEMENT_3D('',#206586,#106160,#106161);
#85996=AXIS2_PLACEMENT_3D('',#206734,#106163,#106164);
#85997=AXIS2_PLACEMENT_3D('',#206878,#106166,#106167);
#85998=AXIS2_PLACEMENT_3D('',#206906,#106170,#106171);
#85999=AXIS2_PLACEMENT_3D('',#207040,#106173,#106174);
#86000=AXIS2_PLACEMENT_3D('',#207168,#106176,#106177);
#86001=AXIS2_PLACEMENT_3D('',#207314,#106179,#106180);
#86002=AXIS2_PLACEMENT_3D('',#207330,#106182,#106183);
#86003=AXIS2_PLACEMENT_3D('',#207331,#106184,#106185);
#86004=AXIS2_PLACEMENT_3D('',#207411,#106187,#106188);
#86005=AXIS2_PLACEMENT_3D('',#207484,#106189,#106190);
#86006=AXIS2_PLACEMENT_3D('',#207642,#106192,#106193);
#86007=AXIS2_PLACEMENT_3D('',#207800,#106195,#106196);
#86008=AXIS2_PLACEMENT_3D('',#207858,#106199,#106200);
#86009=AXIS2_PLACEMENT_3D('',#208016,#106202,#106203);
#86010=AXIS2_PLACEMENT_3D('',#208178,#106205,#106206);
#86011=AXIS2_PLACEMENT_3D('',#208336,#106208,#106209);
#86012=AXIS2_PLACEMENT_3D('',#208341,#106211,#106212);
#86013=AXIS2_PLACEMENT_3D('',#208414,#106213,#106214);
#86014=AXIS2_PLACEMENT_3D('',#208452,#106215,#106216);
#86015=AXIS2_PLACEMENT_3D('',#208466,#106217,#106218);
#86016=AXIS2_PLACEMENT_3D('',#208467,#106219,#106220);
#86017=AXIS2_PLACEMENT_3D('',#208469,#106221,#106222);
#86018=AXIS2_PLACEMENT_3D('',#208472,#106224,#106225);
#86019=AXIS2_PLACEMENT_3D('',#208473,#106226,#106227);
#86020=AXIS2_PLACEMENT_3D('',#208490,#106228,#106229);
#86021=AXIS2_PLACEMENT_3D('',#208525,#106230,#106231);
#86022=AXIS2_PLACEMENT_3D('',#208558,#106232,#106233);
#86023=AXIS2_PLACEMENT_3D('',#208592,#106236,#106237);
#86024=AXIS2_PLACEMENT_3D('',#208594,#106238,#106239);
#86025=AXIS2_PLACEMENT_3D('',#208725,#106240,#106241);
#86026=AXIS2_PLACEMENT_3D('',#208846,#106242,#106243);
#86027=AXIS2_PLACEMENT_3D('',#209644,#106247,#106248);
#86028=AXIS2_PLACEMENT_3D('',#210311,#106251,#106252);
#86029=AXIS2_PLACEMENT_3D('',#210316,#106254,#106255);
#86030=AXIS2_PLACEMENT_3D('',#210317,#106256,#106257);
#86031=AXIS2_PLACEMENT_3D('',#210318,#106258,#106259);
#86032=AXIS2_PLACEMENT_3D('',#210319,#106260,#106261);
#86033=AXIS2_PLACEMENT_3D('',#210320,#106262,#106263);
#86034=AXIS2_PLACEMENT_3D('',#210322,#106264,#106265);
#86035=AXIS2_PLACEMENT_3D('',#210333,#106266,#106267);
#86036=AXIS2_PLACEMENT_3D('',#211402,#106270,#106271);
#86037=AXIS2_PLACEMENT_3D('',#212210,#106274,#106275);
#86038=AXIS2_PLACEMENT_3D('',#212631,#106277,#106278);
#86039=AXIS2_PLACEMENT_3D('',#212634,#106279,#106280);
#86040=AXIS2_PLACEMENT_3D('',#212637,#106282,#106283);
#86041=AXIS2_PLACEMENT_3D('',#212638,#106284,#106285);
#86042=AXIS2_PLACEMENT_3D('',#212639,#106286,#106287);
#86043=AXIS2_PLACEMENT_3D('',#212642,#106289,#106290);
#86044=AXIS2_PLACEMENT_3D('',#212643,#106291,#106292);
#86045=AXIS2_PLACEMENT_3D('',#212644,#106293,#106294);
#86046=AXIS2_PLACEMENT_3D('',#212645,#106295,#106296);
#86047=AXIS2_PLACEMENT_3D('',#212647,#106297,#106298);
#86048=AXIS2_PLACEMENT_3D('',#212648,#106299,#106300);
#86049=AXIS2_PLACEMENT_3D('',#212651,#106302,#106303);
#86050=AXIS2_PLACEMENT_3D('',#212652,#106304,#106305);
#86051=AXIS2_PLACEMENT_3D('',#212655,#106307,#106308);
#86052=AXIS2_PLACEMENT_3D('',#212656,#106309,#106310);
#86053=AXIS2_PLACEMENT_3D('',#212663,#106311,#106312);
#86054=AXIS2_PLACEMENT_3D('',#212772,#106313,#106314);
#86055=AXIS2_PLACEMENT_3D('',#212784,#106315,#106316);
#86056=AXIS2_PLACEMENT_3D('',#212785,#106317,#106318);
#86057=AXIS2_PLACEMENT_3D('',#212786,#106319,#106320);
#86058=AXIS2_PLACEMENT_3D('',#212788,#106322,#106323);
#106079=DIRECTION('axis',(0.,0.,1.));
#106080=DIRECTION('refdir',(1.,0.,0.));
#106081=DIRECTION('center_axis',(-1.,0.,0.));
#106082=DIRECTION('ref_axis',(0.,-0.924224592736303,-0.381849318686593));
#106083=DIRECTION('',(1.,0.,0.));
#106084=DIRECTION('',(1.,0.,0.));
#106085=DIRECTION('center_axis',(-1.,0.,0.));
#106086=DIRECTION('ref_axis',(0.,0.924224592736303,0.381849318686593));
#106087=DIRECTION('center_axis',(-1.,0.,0.));
#106088=DIRECTION('ref_axis',(0.,0.924224592736303,0.381849318686593));
#106089=DIRECTION('',(-1.,0.,0.));
#106090=DIRECTION('center_axis',(-1.,0.,0.));
#106091=DIRECTION('ref_axis',(0.,-0.924224592736303,-0.381849318686593));
#106092=DIRECTION('',(1.,0.,0.));
#106093=DIRECTION('center_axis',(-1.,0.,0.));
#106094=DIRECTION('ref_axis',(0.,-0.924224592736303,-0.381849318686593));
#106095=DIRECTION('',(1.,0.,0.));
#106096=DIRECTION('center_axis',(-1.,0.,0.));
#106097=DIRECTION('ref_axis',(0.,-0.924224592736303,-0.381849318686593));
#106098=DIRECTION('',(1.,0.,0.));
#106099=DIRECTION('center_axis',(-1.,0.,0.));
#106100=DIRECTION('ref_axis',(0.,-0.924224592736303,-0.381849318686593));
#106101=DIRECTION('',(1.,0.,0.));
#106102=DIRECTION('center_axis',(-1.,0.,0.));
#106103=DIRECTION('ref_axis',(0.,-0.924224592736303,-0.381849318686593));
#106104=DIRECTION('',(1.,0.,0.));
#106105=DIRECTION('center_axis',(-1.,0.,0.));
#106106=DIRECTION('ref_axis',(0.,-0.924224592736303,-0.381849318686593));
#106107=DIRECTION('',(1.,0.,0.));
#106108=DIRECTION('center_axis',(-1.,0.,0.));
#106109=DIRECTION('ref_axis',(0.,-0.924224592736303,-0.381849318686593));
#106110=DIRECTION('',(1.,0.,0.));
#106111=DIRECTION('center_axis',(-1.,0.,0.));
#106112=DIRECTION('ref_axis',(0.,-0.924224592736303,-0.381849318686593));
#106113=DIRECTION('',(1.,0.,0.));
#106114=DIRECTION('center_axis',(1.,0.,0.));
#106115=DIRECTION('ref_axis',(0.,0.999244149014678,-0.0388732640761329));
#106116=DIRECTION('center_axis',(-1.,0.,0.));
#106117=DIRECTION('ref_axis',(0.,-0.924224592736303,-0.381849318686593));
#106118=DIRECTION('',(1.,0.,0.));
#106119=DIRECTION('center_axis',(1.,0.,0.));
#106120=DIRECTION('ref_axis',(0.,0.999244149014678,-0.0388732640761329));
#106121=DIRECTION('center_axis',(-1.,0.,0.));
#106122=DIRECTION('ref_axis',(0.,-0.924224592736303,-0.381849318686593));
#106123=DIRECTION('',(1.,0.,0.));
#106124=DIRECTION('center_axis',(-1.,0.,0.));
#106125=DIRECTION('ref_axis',(0.,-0.924224592736303,-0.381849318686593));
#106126=DIRECTION('',(1.,0.,0.));
#106127=DIRECTION('center_axis',(-1.,0.,0.));
#106128=DIRECTION('ref_axis',(0.,-0.924224592736303,-0.381849318686593));
#106129=DIRECTION('',(1.,0.,0.));
#106130=DIRECTION('center_axis',(-1.,0.,0.));
#106131=DIRECTION('ref_axis',(0.,-0.924224592736303,-0.381849318686593));
#106132=DIRECTION('',(1.,0.,0.));
#106133=DIRECTION('center_axis',(-1.,0.,0.));
#106134=DIRECTION('ref_axis',(0.,-0.924224592736303,-0.381849318686593));
#106135=DIRECTION('',(1.,0.,0.));
#106136=DIRECTION('center_axis',(-1.,0.,0.));
#106137=DIRECTION('ref_axis',(0.,-0.924224592736303,-0.381849318686593));
#106138=DIRECTION('',(1.,0.,0.));
#106139=DIRECTION('center_axis',(-1.,0.,0.));
#106140=DIRECTION('ref_axis',(0.,-0.924224592736303,-0.381849318686593));
#106141=DIRECTION('center_axis',(1.,0.,0.));
#106142=DIRECTION('ref_axis',(0.,-0.924224592736303,-0.381849318686593));
#106143=DIRECTION('center_axis',(1.,0.,0.));
#106144=DIRECTION('ref_axis',(0.,-0.924224592736303,-0.381849318686593));
#106145=DIRECTION('',(1.,0.,0.));
#106146=DIRECTION('',(-1.,0.,0.));
#106147=DIRECTION('',(1.,0.,0.));
#106148=DIRECTION('center_axis',(-1.,7.59792509022099E-17,3.13913148593356E-17));
#106149=DIRECTION('ref_axis',(-8.2208644413218E-17,-0.924224592736303,-0.381849318686593));
#106150=DIRECTION('',(0.70710665146941,-0.653525596750962,-0.270008292167144));
#106151=DIRECTION('center_axis',(1.,0.,0.));
#106152=DIRECTION('ref_axis',(0.,-0.050910732461195,0.99870320782516));
#106153=DIRECTION('center_axis',(1.,0.,0.));
#106154=DIRECTION('ref_axis',(0.,0.924224592736303,0.381849318686593));
#106155=DIRECTION('',(-1.,0.,0.));
#106156=DIRECTION('',(0.999999999998702,-7.34588796642656E-7,-1.43405400215834E-6));
#106157=DIRECTION('center_axis',(1.,0.,0.));
#106158=DIRECTION('ref_axis',(0.,0.924224592736303,0.381849318686593));
#106159=DIRECTION('',(-1.,0.,0.));
#106160=DIRECTION('center_axis',(1.,0.,0.));
#106161=DIRECTION('ref_axis',(0.,0.924224592736303,0.381849318686593));
#106162=DIRECTION('',(-1.,0.,0.));
#106163=DIRECTION('center_axis',(1.,0.,0.));
#106164=DIRECTION('ref_axis',(0.,0.924224592736303,0.381849318686593));
#106165=DIRECTION('',(-1.,0.,0.));
#106166=DIRECTION('center_axis',(1.,0.,0.));
#106167=DIRECTION('ref_axis',(0.,0.924224592736303,0.381849318686592));
#106168=DIRECTION('',(-1.,0.,0.));
#106169=DIRECTION('',(0.999999999947399,4.18358171207589E-7,1.02482902784251E-5));
#106170=DIRECTION('center_axis',(1.,0.,0.));
#106171=DIRECTION('ref_axis',(0.,0.924224592736303,0.381849318686592));
#106172=DIRECTION('',(-1.,0.,0.));
#106173=DIRECTION('center_axis',(1.,0.,0.));
#106174=DIRECTION('ref_axis',(0.,0.924224592736303,0.381849318686592));
#106175=DIRECTION('',(-1.,0.,0.));
#106176=DIRECTION('center_axis',(1.,0.,0.));
#106177=DIRECTION('ref_axis',(0.,0.924224592736303,0.381849318686592));
#106178=DIRECTION('',(-1.,0.,0.));
#106179=DIRECTION('center_axis',(1.,0.,0.));
#106180=DIRECTION('ref_axis',(0.,0.924224592736303,0.381849318686592));
#106181=DIRECTION('',(-1.,0.,0.));
#106182=DIRECTION('center_axis',(-1.,0.,0.));
#106183=DIRECTION('ref_axis',(0.,0.924224592736303,0.381849318686592));
#106184=DIRECTION('center_axis',(1.,1.82571941840305E-14,2.33421417227065E-14));
#106185=DIRECTION('ref_axis',(-2.57869287727445E-14,0.924224592736303,0.381849318686593));
#106186=DIRECTION('',(-1.,-1.82571941840305E-14,-2.33421417227065E-14));
#106187=DIRECTION('center_axis',(0.,-0.695858933987439,0.718178490341966));
#106188=DIRECTION('ref_axis',(-0.0305944370091769,0.717842297089703,0.69553318895152));
#106189=DIRECTION('center_axis',(1.,1.82571941840305E-14,2.33421417227065E-14));
#106190=DIRECTION('ref_axis',(-2.57869287727445E-14,0.924224592736303,0.381849318686593));
#106191=DIRECTION('',(-1.,-1.82571941840305E-14,-2.33421417227065E-14));
#106192=DIRECTION('center_axis',(1.,1.82571941840305E-14,2.33421417227065E-14));
#106193=DIRECTION('ref_axis',(-2.57869287727445E-14,0.924224592736303,0.381849318686593));
#106194=DIRECTION('',(-1.,-1.82571941840305E-14,-2.33421417227065E-14));
#106195=DIRECTION('center_axis',(1.,0.,0.));
#106196=DIRECTION('ref_axis',(0.,0.924224592736303,0.381849318686593));
#106197=DIRECTION('',(-1.,0.,0.));
#106198=DIRECTION('',(-0.999999999940701,1.01456975879523E-5,3.95770558922334E-6));
#106199=DIRECTION('center_axis',(1.,0.,0.));
#106200=DIRECTION('ref_axis',(0.,0.924224592736303,0.381849318686593));
#106201=DIRECTION('',(-1.,0.,0.));
#106202=DIRECTION('center_axis',(1.,0.,0.));
#106203=DIRECTION('ref_axis',(0.,0.924224592736303,0.381849318686593));
#106204=DIRECTION('',(-1.,0.,0.));
#106205=DIRECTION('center_axis',(1.,0.,0.));
#106206=DIRECTION('ref_axis',(0.,0.924224592736303,0.381849318686593));
#106207=DIRECTION('',(-1.,0.,0.));
#106208=DIRECTION('center_axis',(1.,-2.54046812768854E-17,-1.04961070212471E-17));
#106209=DIRECTION('ref_axis',(2.74875625216498E-17,0.924224592736303,0.381849318686593));
#106210=DIRECTION('',(-0.707106662296841,0.653525586743986,0.270008288032699));
#106211=DIRECTION('center_axis',(-1.,0.,0.));
#106212=DIRECTION('ref_axis',(0.,-0.316348137924587,-0.948643165595814));
#106213=DIRECTION('center_axis',(-1.,0.,0.));
#106214=DIRECTION('ref_axis',(0.,-0.916443657855559,0.400163743955299));
#106215=DIRECTION('center_axis',(1.,-2.54046812768854E-17,-1.04961070212471E-17));
#106216=DIRECTION('ref_axis',(2.74875625216498E-17,0.924224592736303,0.381849318686593));
#106217=DIRECTION('center_axis',(-1.,0.,0.));
#106218=DIRECTION('ref_axis',(0.,-0.316348137924587,-0.948643165595814));
#106219=DIRECTION('center_axis',(0.965925826289076,0.239206926552251,0.0988298760355017));
#106220=DIRECTION('ref_axis',(-0.258819045102494,0.892732403415498,0.368838118670266));
#106221=DIRECTION('center_axis',(1.,2.30623636574203E-15,5.83716380003748E-15));
#106222=DIRECTION('ref_axis',(-4.3603973859905E-15,0.924224592736086,0.381849318687119));
#106223=DIRECTION('',(0.965925826289076,0.239206926552251,0.0988298760355017));
#106224=DIRECTION('center_axis',(1.,-2.30623636574271E-15,-5.83716380003825E-15));
#106225=DIRECTION('ref_axis',(4.36039738597361E-15,0.924224592737593,0.381849318683469));
#106226=DIRECTION('center_axis',(1.,0.,0.));
#106227=DIRECTION('ref_axis',(0.,0.924224592736303,0.381849318686593));
#106228=DIRECTION('center_axis',(1.,1.82571941840305E-14,2.33421417227065E-14));
#106229=DIRECTION('ref_axis',(-2.57869287727445E-14,0.924224592736303,0.381849318686593));
#106230=DIRECTION('center_axis',(0.,-0.393059646033816,-0.919512976884922));
#106231=DIRECTION('ref_axis',(-0.013064730535851,-0.919434498995661,0.393026099480206));
#106232=DIRECTION('center_axis',(0.965925826289076,0.239206926552251,0.0988298760355016));
#106233=DIRECTION('ref_axis',(-0.258819045102493,0.892732403415498,0.368838118670267));
#106234=DIRECTION('',(0.965925826289076,0.239206926552251,0.0988298760355015));
#106235=DIRECTION('',(0.965925826289076,0.239206926552251,0.0988298760355015));
#106236=DIRECTION('center_axis',(1.,0.,0.));
#106237=DIRECTION('ref_axis',(0.,0.924224592736303,0.381849318686592));
#106238=DIRECTION('center_axis',(-1.,0.,0.));
#106239=DIRECTION('ref_axis',(0.,0.924224592736303,0.381849318686592));
#106240=DIRECTION('center_axis',(1.,0.,0.));
#106241=DIRECTION('ref_axis',(0.,0.924224592736303,0.381849318686592));
#106242=DIRECTION('center_axis',(1.,0.,0.));
#106243=DIRECTION('ref_axis',(0.,0.924224592736303,0.381849318686593));
#106244=DIRECTION('',(1.,0.,0.));
#106245=DIRECTION('',(0.461762345735445,0.886264698784526,-0.0361997202927374));
#106246=DIRECTION('',(0.461762444463603,0.789444381060389,-0.404416881565516));
#106247=DIRECTION('center_axis',(0.,0.888370688458611,-0.459126910437161));
#106248=DIRECTION('ref_axis',(-1.,0.,0.));
#106249=DIRECTION('',(0.461762450482966,-0.789465505391419,0.404375636161525));
#106250=DIRECTION('',(0.461762365531076,-0.886266296190208,0.0361603376150716));
#106251=DIRECTION('center_axis',(0.,0.381849318686593,-0.924224592736303));
#106252=DIRECTION('ref_axis',(-1.,0.,0.));
#106253=DIRECTION('',(0.965925826289076,0.239206926552251,0.0988298760355015));
#106254=DIRECTION('center_axis',(-3.19816689560775E-17,0.381849318686593,
-0.924224592736303));
#106255=DIRECTION('ref_axis',(0.995486289304339,0.0877139672710818,0.0362395881964125));
#106256=DIRECTION('center_axis',(-3.19816689560775E-17,0.381849318686593,
-0.924224592736303));
#106257=DIRECTION('ref_axis',(0.995486289304339,0.0877139672710818,0.0362395881964125));
#106258=DIRECTION('center_axis',(-2.85555636349464E-16,0.381849318686593,
-0.924224592736303));
#106259=DIRECTION('ref_axis',(-0.989158808077185,-0.135722160860674,-0.0560744813139883));
#106260=DIRECTION('center_axis',(1.,0.,0.));
#106261=DIRECTION('ref_axis',(0.,-0.381849318686593,0.924224592736303));
#106262=DIRECTION('center_axis',(0.,0.924224592736303,0.381849318686593));
#106263=DIRECTION('ref_axis',(0.,0.381849318686593,-0.924224592736303));
#106264=DIRECTION('center_axis',(-8.53563043435897E-18,-0.381849318686593,
0.924224592736303));
#106265=DIRECTION('ref_axis',(-0.999927597212881,-0.0111214726821253,-0.00459490777440583));
#106266=DIRECTION('center_axis',(-1.,7.59792509022099E-17,3.13913148593356E-17));
#106267=DIRECTION('ref_axis',(-8.2208644413218E-17,-0.924224592736303,-0.381849318686593));
#106268=DIRECTION('',(-1.,0.,0.));
#106269=DIRECTION('',(-0.46175507312697,0.636992745624861,0.617270195670266));
#106270=DIRECTION('center_axis',(0.,-0.0569081128227818,-0.998379420208044));
#106271=DIRECTION('ref_axis',(0.,-0.998379420208044,0.0569081128227818));
#106272=DIRECTION('',(-0.461755065119691,-0.636985304497725,-0.617277880447899));
#106273=DIRECTION('',(-0.461755171831996,0.815781579343936,-0.348256480326666));
#106274=DIRECTION('center_axis',(-1.,0.,0.));
#106275=DIRECTION('ref_axis',(0.,-0.924224592736303,-0.381849318686593));
#106276=DIRECTION('',(-0.461755171705888,-0.815781579302173,0.348256480591701));
#106277=DIRECTION('center_axis',(-1.,0.,0.));
#106278=DIRECTION('ref_axis',(0.,-0.924224592736303,-0.381849318686592));
#106279=DIRECTION('center_axis',(-1.,0.,0.));
#106280=DIRECTION('ref_axis',(0.,-0.924224592736303,-0.381849318686592));
#106281=DIRECTION('',(-1.,0.,0.));
#106282=DIRECTION('center_axis',(-1.,0.,0.));
#106283=DIRECTION('ref_axis',(0.,-0.924224592736303,-0.381849318686592));
#106284=DIRECTION('center_axis',(-1.,0.,0.));
#106285=DIRECTION('ref_axis',(0.,-0.924224592736303,-0.381849318686592));
#106286=DIRECTION('center_axis',(1.,3.80693114761575E-17,1.57285802220435E-17));
#106287=DIRECTION('ref_axis',(-4.11905415364978E-17,0.924224592736303,0.381849318686593));
#106288=DIRECTION('',(0.707106580681804,-0.653525662174577,-0.270008319197331));
#106289=DIRECTION('center_axis',(-1.,0.,0.));
#106290=DIRECTION('ref_axis',(-4.11905415364978E-17,0.924224592736303,0.381849318686593));
#106291=DIRECTION('center_axis',(-1.,0.,0.));
#106292=DIRECTION('ref_axis',(0.,0.,1.));
#106293=DIRECTION('center_axis',(-1.,0.,0.));
#106294=DIRECTION('ref_axis',(0.,0.,1.));
#106295=DIRECTION('center_axis',(-1.,0.,0.));
#106296=DIRECTION('ref_axis',(0.,0.,1.));
#106297=DIRECTION('center_axis',(-1.,0.,0.));
#106298=DIRECTION('ref_axis',(0.,-0.924224592736303,-0.381849318686592));
#106299=DIRECTION('center_axis',(-1.,0.,0.));
#106300=DIRECTION('ref_axis',(0.,-0.924224592736303,-0.381849318686592));
#106301=DIRECTION('',(-1.,0.,0.));
#106302=DIRECTION('center_axis',(1.,0.,0.));
#106303=DIRECTION('ref_axis',(0.,0.924224592736303,0.381849318686592));
#106304=DIRECTION('center_axis',(-1.,2.54488112923718E-17,1.05143396202058E-17));
#106305=DIRECTION('ref_axis',(-2.75353106727304E-17,-0.924224592736303,
-0.381849318686592));
#106306=DIRECTION('',(-0.7071070062405,0.653525268862752,0.270008156698027));
#106307=DIRECTION('center_axis',(1.,0.,0.));
#106308=DIRECTION('ref_axis',(0.,-0.924224592736303,-0.381849318686592));
#106309=DIRECTION('center_axis',(-1.,0.,0.));
#106310=DIRECTION('ref_axis',(0.,0.,1.));
#106311=DIRECTION('center_axis',(-1.,0.,0.));
#106312=DIRECTION('ref_axis',(0.,-0.924224592736303,-0.381849318686593));
#106313=DIRECTION('center_axis',(1.,0.,0.));
#106314=DIRECTION('ref_axis',(0.,-0.381849318686592,0.924224592736303));
#106315=DIRECTION('center_axis',(7.6756005494586E-17,-0.381849318686593,
0.924224592736303));
#106316=DIRECTION('ref_axis',(0.99903497276754,-0.0405935937462799,-0.0167715036332949));
#106317=DIRECTION('center_axis',(0.,0.924224592736303,0.381849318686592));
#106318=DIRECTION('ref_axis',(0.,0.381849318686592,-0.924224592736303));
#106319=DIRECTION('center_axis',(0.,-0.381849318686593,0.924224592736303));
#106320=DIRECTION('ref_axis',(-1.,0.,0.));
#106321=DIRECTION('',(0.965925826289076,0.239206926552251,0.0988298760355015));
#106322=DIRECTION('center_axis',(0.965925826289076,0.239206926552251,0.0988298760355016));
#106323=DIRECTION('ref_axis',(0.258819045102494,-0.892732403415497,-0.36883811867027));
#203966=CARTESIAN_POINT('',(0.,0.,0.));
#203967=CARTESIAN_POINT('Origin',(-45.8894114130409,-83.3180213346267,69.5522455184007));
#203968=CARTESIAN_POINT('',(-50.2096235848678,-73.8447192590796,73.4662010349383));
#203969=CARTESIAN_POINT('',(-49.8038356726598,-73.8447192590796,73.4662010349383));
#203970=CARTESIAN_POINT('',(-45.8894114130409,-73.8447192590796,73.4662010349383));
#203971=CARTESIAN_POINT('',(-48.3958698180353,-73.8447192590796,73.4662010349383));
#203972=CARTESIAN_POINT('Ctrl Pts',(-48.3958698180353,-73.8447192590796,
73.4662010349383));
#203973=CARTESIAN_POINT('Ctrl Pts',(-48.4037688023958,-73.7386706426075,
73.2095219351658));
#203974=CARTESIAN_POINT('Ctrl Pts',(-48.4116574949273,-73.6430539000291,
72.9485323067095));
#203975=CARTESIAN_POINT('Ctrl Pts',(-48.4339260978028,-73.4009224543471,
72.1939151829407));
#203976=CARTESIAN_POINT('Ctrl Pts',(-48.4481645682176,-73.2808293376766,
71.6928179235221));
#203977=CARTESIAN_POINT('Ctrl Pts',(-48.480466899021,-73.0972451440741,
70.5549159518891));
#203978=CARTESIAN_POINT('Ctrl Pts',(-48.4985953623062,-73.0546578172561,
69.9168948451602));
#203979=CARTESIAN_POINT('Ctrl Pts',(-48.5346718023404,-73.0884937885025,
68.6477279521232));
#203980=CARTESIAN_POINT('Ctrl Pts',(-48.5522008894746,-73.1636417714324,
68.0192859017049));
#203981=CARTESIAN_POINT('Ctrl Pts',(-48.5881875157042,-73.4338516390347,
66.7600280206718));
#203982=CARTESIAN_POINT('Ctrl Pts',(-48.6067347220618,-73.632875106913,
66.1330034080448));
#203983=CARTESIAN_POINT('Ctrl Pts',(-48.657339605336,-74.331064994807,64.4968207509486));
#203984=CARTESIAN_POINT('Ctrl Pts',(-48.6880625258242,-74.9383023010144,
63.5436661186597));
#203985=CARTESIAN_POINT('Ctrl Pts',(-48.7390155039672,-76.1391472861404,
62.2049346832462));
#203986=CARTESIAN_POINT('Ctrl Pts',(-48.7583174976583,-76.6390544266697,
61.747719387351));
#203987=CARTESIAN_POINT('Ctrl Pts',(-48.7960590212527,-77.7208277256431,
60.938919054492));
#203988=CARTESIAN_POINT('Ctrl Pts',(-48.8147908333194,-78.2999318592946,
60.5891687634112));
#203989=CARTESIAN_POINT('Ctrl Pts',(-48.8432065712902,-79.2059868334308,
60.1574727831644));
#203990=CARTESIAN_POINT('Ctrl Pts',(-48.8525662532641,-79.5094106761401,
60.0304249838887));
#203991=CARTESIAN_POINT('Ctrl Pts',(-48.8912166329455,-80.7871613627979,
59.5662775472869));
#203992=CARTESIAN_POINT('Ctrl Pts',(-48.9194279440347,-81.8034663869601,
59.362498805665));
#203993=CARTESIAN_POINT('Ctrl Pts',(-48.9579250197248,-83.1622898710032,
59.2981281043926));
#203994=CARTESIAN_POINT('Ctrl Pts',(-48.9673076225165,-83.4921415542527,
59.2984239272769));
#203995=CARTESIAN_POINT('Ctrl Pts',(-49.0066694377159,-84.8746715504436,
59.3664025361002));
#203996=CARTESIAN_POINT('Ctrl Pts',(-49.0355301671101,-85.9136649961914,
59.5804252807785));
#203997=CARTESIAN_POINT('Ctrl Pts',(-49.0821868355881,-87.4577419933632,
60.1566345648574));
#203998=CARTESIAN_POINT('Ctrl Pts',(-49.0991802722567,-87.9947530123903,
60.412060635265));
#203999=CARTESIAN_POINT('Ctrl Pts',(-49.130122341021,-88.9451920275598,
60.9699355087346));
#204000=CARTESIAN_POINT('Ctrl Pts',(-49.1441985526236,-89.3639849856817,
61.2596329916114));
#204001=CARTESIAN_POINT('Ctrl Pts',(-49.1763003559444,-90.2547807826329,
61.9793192667773));
#204002=CARTESIAN_POINT('Ctrl Pts',(-49.1943953113045,-90.7116591687776,
62.4246969029591));
#204003=CARTESIAN_POINT('Ctrl Pts',(-49.2304152840414,-91.5332756733942,
63.3902299748733));
#204004=CARTESIAN_POINT('Ctrl Pts',(-49.2479248411482,-91.8970273447589,
63.9076464520963));
#204005=CARTESIAN_POINT('Ctrl Pts',(-49.2838818041742,-92.5368653667999,
65.0239821634796));
#204006=CARTESIAN_POINT('Ctrl Pts',(-49.3024121914913,-92.8075370872142,
65.6226997428383));
#204007=CARTESIAN_POINT('Ctrl Pts',(-49.3595038029608,-93.4554727643574,
67.5222243619057));
#204008=CARTESIAN_POINT('Ctrl Pts',(-49.3964227073141,-93.6345282408168,
68.8750549678309));
#204009=CARTESIAN_POINT('Ctrl Pts',(-49.473309124989,-93.457508738034,71.5719325676014));
#204010=CARTESIAN_POINT('Ctrl Pts',(-49.5102216656477,-93.1032506221796,
72.8895546941323));
#204011=CARTESIAN_POINT('Ctrl Pts',(-49.5748954774791,-92.0944299133281,
74.9269751780849));
#204012=CARTESIAN_POINT('Ctrl Pts',(-49.6003951487874,-91.5755097026235,
75.6944736760051));
#204013=CARTESIAN_POINT('Ctrl Pts',(-49.6510179783252,-90.3743525456944,
77.0386154460731));
#204014=CARTESIAN_POINT('Ctrl Pts',(-49.6762791930195,-89.705601088901,
77.6167589418837));
#204015=CARTESIAN_POINT('Ctrl Pts',(-49.7143859714278,-88.5696143825758,
78.3678616677063));
#204016=CARTESIAN_POINT('Ctrl Pts',(-49.727738082698,-88.1497797203329,
78.6047827076002));
#204017=CARTESIAN_POINT('Ctrl Pts',(-49.7606212091936,-87.0916211277151,
79.1072676497953));
#204018=CARTESIAN_POINT('Ctrl Pts',(-49.7803096541967,-86.4401008290713,
79.3395385943935));
#204019=CARTESIAN_POINT('Ctrl Pts',(-49.8093097839274,-85.4456603226875,
79.5845625524906));
#204020=CARTESIAN_POINT('Ctrl Pts',(-49.8186505287261,-85.1173873690851,
79.6486070096269));
#204021=CARTESIAN_POINT('Ctrl Pts',(-49.8457240773238,-84.1567284833155,
79.7876783315113));
#204022=CARTESIAN_POINT('Ctrl Pts',(-49.8634779845325,-83.5197662041813,
79.8200011829918));
#204023=CARTESIAN_POINT('Ctrl Pts',(-49.8956682408467,-82.3857593300351,
79.7719330243677));
#204024=CARTESIAN_POINT('Ctrl Pts',(-49.9099239632542,-81.8897876487362,
79.7144930808433));
#204025=CARTESIAN_POINT('Ctrl Pts',(-49.9387558076438,-80.8833860201483,
79.522781806287));
#204026=CARTESIAN_POINT('Ctrl Pts',(-49.9532988892753,-80.3751380966072,
79.384767434848));
#204027=CARTESIAN_POINT('Ctrl Pts',(-49.9859711911988,-79.2764357760924,
78.9935480759183));
#204028=CARTESIAN_POINT('Ctrl Pts',(-50.0041557488463,-78.6946047619587,
78.7226660461564));
#204029=CARTESIAN_POINT('Ctrl Pts',(-50.0403294878792,-77.5960381700283,
78.07992568427));
#204030=CARTESIAN_POINT('Ctrl Pts',(-50.057894567962,-77.0809299480628,
77.7107451120727));
#204031=CARTESIAN_POINT('Ctrl Pts',(-50.0939331145918,-76.1062593244605,
76.8656229924851));
#204032=CARTESIAN_POINT('Ctrl Pts',(-50.1125077195411,-75.6520038235377,
76.3879723904082));
#204033=CARTESIAN_POINT('Ctrl Pts',(-50.1577532611068,-74.67166569896,75.1355452763787));
#204034=CARTESIAN_POINT('Ctrl Pts',(-50.1834334662541,-74.2002175935722,
74.3266459469391));
#204035=CARTESIAN_POINT('Ctrl Pts',(-50.2096235848678,-73.8447192590796,
73.4662010349383));
#204036=CARTESIAN_POINT('',(-47.5675364832709,-73.8447192590796,73.4662010349383));
#204037=CARTESIAN_POINT('',(-45.8894114130409,-73.8447192590796,73.4662010349383));
#204038=CARTESIAN_POINT('',(-47.5675364832709,-79.4040658180891,60.0789434428536));
#204039=CARTESIAN_POINT('Origin',(-47.5675364832709,-83.3180213346267,69.5522455184007));
#204040=CARTESIAN_POINT('Origin',(-47.5675364832709,-83.3180213346267,69.5522455184007));
#204041=CARTESIAN_POINT('',(-47.8635970591063,-89.6396660823375,77.6206672715227));
#204042=CARTESIAN_POINT('Ctrl Pts',(-47.8635486253615,-89.639547528851,
77.6207526030934));
#204043=CARTESIAN_POINT('Ctrl Pts',(-47.8770445391941,-89.2585502588736,
77.9192569232619));
#204044=CARTESIAN_POINT('Ctrl Pts',(-47.8905695996721,-88.8568898237617,
78.1903990846767));
#204045=CARTESIAN_POINT('Ctrl Pts',(-47.9176339376232,-88.0279594985981,
78.6683051771889));
#204046=CARTESIAN_POINT('Ctrl Pts',(-47.9311316261011,-87.6024902668963,
78.8758384030079));
#204047=CARTESIAN_POINT('Ctrl Pts',(-47.9711978571694,-86.2919724125154,
79.4063621105855));
#204048=CARTESIAN_POINT('Ctrl Pts',(-47.9969625168339,-85.3752442622018,
79.6376724024459));
#204049=CARTESIAN_POINT('Ctrl Pts',(-48.0398242697937,-83.8709049161899,
79.8033179102035));
#204050=CARTESIAN_POINT('Ctrl Pts',(-48.0562071817464,-83.2976725144938,
79.8181968614348));
#204051=CARTESIAN_POINT('Ctrl Pts',(-48.0866529239232,-82.2155375469544,
79.7556116214413));
#204052=CARTESIAN_POINT('Ctrl Pts',(-48.1008092000048,-81.7077987292351,
79.6878924020851));
#204053=CARTESIAN_POINT('Ctrl Pts',(-48.1330146582569,-80.5833618276912,
79.4512656104272));
#204054=CARTESIAN_POINT('Ctrl Pts',(-48.1511310418103,-79.9730946449028,
79.2620556484616));
#204055=CARTESIAN_POINT('Ctrl Pts',(-48.1871877210263,-78.8013052805535,
78.7750688738245));
#204056=CARTESIAN_POINT('Ctrl Pts',(-48.2047101916097,-78.2418707084766,
78.4793891225225));
#204057=CARTESIAN_POINT('Ctrl Pts',(-48.2406868075071,-77.1638968790423,
77.7753651650062));
#204058=CARTESIAN_POINT('Ctrl Pts',(-48.2592283648658,-76.6503036986312,
77.3647016622442));
#204059=CARTESIAN_POINT('Ctrl Pts',(-48.3097623744413,-75.3754982319245,
76.1275080151719));
#204060=CARTESIAN_POINT('Ctrl Pts',(-48.3404245900448,-74.7048426895327,
75.2206595097633));
#204061=CARTESIAN_POINT('Ctrl Pts',(-48.3800496111431,-74.0674708014668,
73.9757305662848));
#204062=CARTESIAN_POINT('Ctrl Pts',(-48.387963293798,-73.9508691029355,
73.723125144543));
#204063=CARTESIAN_POINT('Ctrl Pts',(-48.3958698180353,-73.8447192590796,
73.4662010349383));
#204064=CARTESIAN_POINT('',(-47.8257920924624,-92.7913239034034,65.6382911956717));
#204065=CARTESIAN_POINT('Ctrl Pts',(-47.8635940884284,-89.6412075243314,
77.6194517516842));
#204066=CARTESIAN_POINT('Ctrl Pts',(-47.8609618681876,-90.29911965049,77.1037712608345));
#204067=CARTESIAN_POINT('Ctrl Pts',(-47.8579335141401,-90.8914872330497,
76.5095387599098));
#204068=CARTESIAN_POINT('Ctrl Pts',(-47.8536397962644,-91.9122995837084,
75.1986881766102));
#204069=CARTESIAN_POINT('Ctrl Pts',(-47.852298616386,-92.3389533405578,
74.4885092324321));
#204070=CARTESIAN_POINT('Ctrl Pts',(-47.8482467829845,-92.9035044699208,
73.2254447666301));
#204071=CARTESIAN_POINT('Ctrl Pts',(-47.8461648680152,-93.0892289316702,
72.6982574235016));
#204072=CARTESIAN_POINT('Ctrl Pts',(-47.840752948818,-93.5123572579288,
71.0889018852209));
#204073=CARTESIAN_POINT('Ctrl Pts',(-47.838841880717,-93.6186069667047,
69.9807652008248));
#204074=CARTESIAN_POINT('Ctrl Pts',(-47.8332362516957,-93.4722739304251,
67.763692091706));
#204075=CARTESIAN_POINT('Ctrl Pts',(-47.828574338379,-93.2174407788572,
66.6696609455417));
#204076=CARTESIAN_POINT('Ctrl Pts',(-47.8257920924624,-92.7913239034034,
65.6382911956717));
#204077=CARTESIAN_POINT('',(-47.8068141272352,-88.0240721664947,60.4464459619263));
#204078=CARTESIAN_POINT('Ctrl Pts',(-47.8257920924624,-92.7913239034034,
65.6382911956717));
#204079=CARTESIAN_POINT('Ctrl Pts',(-47.8243052474299,-92.5636050825149,
65.087122450969));
#204080=CARTESIAN_POINT('Ctrl Pts',(-47.8231856641482,-92.2882261844406,
64.556891664567));
#204081=CARTESIAN_POINT('Ctrl Pts',(-47.8203484488529,-91.6444757055702,
63.5441620336233));
#204082=CARTESIAN_POINT('Ctrl Pts',(-47.8182709902653,-91.2762819077662,
63.0643356310676));
#204083=CARTESIAN_POINT('Ctrl Pts',(-47.8141911238361,-90.4598803479546,
62.1752216331248));
#204084=CARTESIAN_POINT('Ctrl Pts',(-47.8123348538898,-90.0132957742932,
61.7676494127296));
#204085=CARTESIAN_POINT('Ctrl Pts',(-47.8093723566015,-89.0590858823477,
61.0399854921902));
#204086=CARTESIAN_POINT('Ctrl Pts',(-47.8082478401419,-88.5540397942691,
60.7203433366149));
#204087=CARTESIAN_POINT('Ctrl Pts',(-47.8068141268167,-88.0240721666117,
60.446445961702));
#204088=CARTESIAN_POINT('',(-48.1735608262671,-88.0240721664362,60.4464459619211));
#204089=CARTESIAN_POINT('',(-47.8068954859909,-88.0240721666105,60.4464459616985));
#204090=CARTESIAN_POINT('',(-48.5599506281375,-92.7913014568048,65.638236866552));
#204091=CARTESIAN_POINT('Ctrl Pts',(-48.1735608267226,-88.0240721665407,
60.4464459616653));
#204092=CARTESIAN_POINT('Ctrl Pts',(-48.2057390453445,-88.5540323787309,
60.7203395041181));
#204093=CARTESIAN_POINT('Ctrl Pts',(-48.2381635012091,-89.0590731093268,
61.0399772116219));
#204094=CARTESIAN_POINT('Ctrl Pts',(-48.3027869041061,-90.0132657864085,
61.7676250678447));
#204095=CARTESIAN_POINT('Ctrl Pts',(-48.3348415809302,-90.4598486250631,
62.175189981084));
#204096=CARTESIAN_POINT('Ctrl Pts',(-48.3987590450242,-91.2763238760333,
63.0643784397394));
#204097=CARTESIAN_POINT('Ctrl Pts',(-48.4306399072594,-91.6445575518518,
63.5442696368761));
#204098=CARTESIAN_POINT('Ctrl Pts',(-48.4954405792784,-92.2882704723868,
64.5569822372555));
#204099=CARTESIAN_POINT('Ctrl Pts',(-48.5278559888906,-92.5636125815672,
65.0871495574296));
#204100=CARTESIAN_POINT('Ctrl Pts',(-48.5599506281375,-92.7913014568048,
65.638236866552));
#204101=CARTESIAN_POINT('',(-49.2715796128967,-89.6395615474175,77.6207039925155));
#204102=CARTESIAN_POINT('Ctrl Pts',(-48.5599506281375,-92.7913014568048,
65.638236866552));
#204103=CARTESIAN_POINT('Ctrl Pts',(-48.6200116739718,-93.2173923022698,
66.6695268548046));
#204104=CARTESIAN_POINT('Ctrl Pts',(-48.6777501611375,-93.472228091973,
67.7634817707358));
#204105=CARTESIAN_POINT('Ctrl Pts',(-48.7973670931621,-93.6186218586882,
69.9805110412447));
#204106=CARTESIAN_POINT('Ctrl Pts',(-48.8573471180377,-93.5123874190092,
71.0887662129763));
#204107=CARTESIAN_POINT('Ctrl Pts',(-48.945646231306,-93.089241678521,72.6982195125106));
#204108=CARTESIAN_POINT('Ctrl Pts',(-48.9749440674501,-92.903517206451,
73.2254112828409));
#204109=CARTESIAN_POINT('Ctrl Pts',(-49.0488658367833,-92.3389663971347,
74.48848740033));
#204110=CARTESIAN_POINT('Ctrl Pts',(-49.0938910637439,-91.9123107069189,
75.198671314922));
#204111=CARTESIAN_POINT('Ctrl Pts',(-49.1831733484294,-90.8915047968733,
76.509518816451));
#204112=CARTESIAN_POINT('Ctrl Pts',(-49.2270302012072,-90.2991361429743,
77.1037580932684));
#204113=CARTESIAN_POINT('Ctrl Pts',(-49.2714848090302,-89.6412093512397,
77.6194503197283));
#204114=CARTESIAN_POINT('Ctrl Pts',(-49.8038356726598,-73.8447192590796,
73.4662010349383));
#204115=CARTESIAN_POINT('Ctrl Pts',(-49.7973206317714,-73.9339046545335,
73.6820645490462));
#204116=CARTESIAN_POINT('Ctrl Pts',(-49.7908122535838,-74.0304697561549,
73.8948834855084));
#204117=CARTESIAN_POINT('Ctrl Pts',(-49.7750566224764,-74.280725526146,
74.3997763747891));
#204118=CARTESIAN_POINT('Ctrl Pts',(-49.7657933185793,-74.4413676838132,
74.6880306542796));
#204119=CARTESIAN_POINT('Ctrl Pts',(-49.7422829552721,-74.8805252003446,
75.3936935266779));
#204120=CARTESIAN_POINT('Ctrl Pts',(-49.727961661627,-75.1762973368638,
75.79933948665));
#204121=CARTESIAN_POINT('Ctrl Pts',(-49.6954955524956,-75.9185369956801,
76.6745882707689));
#204122=CARTESIAN_POINT('Ctrl Pts',(-49.6776829623546,-76.3821893621727,
77.1268327465661));
#204123=CARTESIAN_POINT('Ctrl Pts',(-49.6333168146343,-77.6135001835875,
78.1193750085976));
#204124=CARTESIAN_POINT('Ctrl Pts',(-49.6064851997932,-78.4185952388004,
78.6039249756669));
#204125=CARTESIAN_POINT('Ctrl Pts',(-49.5660277136841,-79.7486669733972,
79.1743177482119));
#204126=CARTESIAN_POINT('Ctrl Pts',(-49.5518256482393,-80.233605180047,
79.3405518921836));
#204127=CARTESIAN_POINT('Ctrl Pts',(-49.5184093692975,-81.3830672892489,
79.6406306448179));
#204128=CARTESIAN_POINT('Ctrl Pts',(-49.4990777274927,-82.0524924873491,
79.7462625759489));
#204129=CARTESIAN_POINT('Ctrl Pts',(-49.4638379832304,-83.2977325994776,
79.8181320445648));
#204130=CARTESIAN_POINT('Ctrl Pts',(-49.448059778772,-83.8697967280917,
79.8033130035401));
#204131=CARTESIAN_POINT('Ctrl Pts',(-49.4056942010153,-85.3734803820745,
79.6380751530243));
#204132=CARTESIAN_POINT('Ctrl Pts',(-49.3786880403919,-86.2906982588559,
79.4067906991592));
#204133=CARTESIAN_POINT('Ctrl Pts',(-49.3390820081314,-87.6018225060059,
78.8761524780747));
#204134=CARTESIAN_POINT('Ctrl Pts',(-49.3259729344058,-88.0274335519023,
78.6685842401965));
#204135=CARTESIAN_POINT('Ctrl Pts',(-49.2991355767715,-88.8566142472486,
78.1905826735702));
#204136=CARTESIAN_POINT('Ctrl Pts',(-49.285430642252,-89.2583801024993,
77.9193842087995));
#204137=CARTESIAN_POINT('Ctrl Pts',(-49.2716572296686,-89.6394684428446,
77.6208145648924));
#204138=CARTESIAN_POINT('Origin',(-45.8894114130409,-83.3180213346267,69.5522455184007));
#204139=CARTESIAN_POINT('',(-52.0239203182307,-73.8447192573355,73.466201030717));
#204140=CARTESIAN_POINT('',(-51.6180871401245,-73.8447192590796,73.4662010349383));
#204141=CARTESIAN_POINT('',(-45.8894114130409,-73.8447192590796,73.4662010349383));
#204142=CARTESIAN_POINT('Ctrl Pts',(-50.2096235848678,-73.8447192590796,
73.4662010349383));
#204143=CARTESIAN_POINT('Ctrl Pts',(-50.2152587311499,-73.7682291466274,
73.2810650675032));
#204144=CARTESIAN_POINT('Ctrl Pts',(-50.2209205166887,-73.6971066797446,
73.093542991864));
#204145=CARTESIAN_POINT('Ctrl Pts',(-50.2421792944865,-73.4517838938014,
72.384532604673));
#204146=CARTESIAN_POINT('Ctrl Pts',(-50.2579032979112,-73.3141470715678,
71.8515923228509));
#204147=CARTESIAN_POINT('Ctrl Pts',(-50.2878406499025,-73.1314464457096,
70.8021108337474));
#204148=CARTESIAN_POINT('Ctrl Pts',(-50.3021105145613,-73.0814677050922,
70.2880755204298));
#204149=CARTESIAN_POINT('Ctrl Pts',(-50.3344513860217,-73.056673214677,
69.1343003713136));
#204150=CARTESIAN_POINT('Ctrl Pts',(-50.3525860612607,-73.1026014222336,
68.4962506052134));
#204151=CARTESIAN_POINT('Ctrl Pts',(-50.3886731043955,-73.3114457217308,
67.2435798090198));
#204152=CARTESIAN_POINT('Ctrl Pts',(-50.4062059720365,-73.4726928682544,
66.6314572753463));
#204153=CARTESIAN_POINT('Ctrl Pts',(-50.4421982095901,-73.9143301697055,
65.421377238379));
#204154=CARTESIAN_POINT('Ctrl Pts',(-50.4607485014183,-74.1981312827367,
64.8277274844779));
#204155=CARTESIAN_POINT('Ctrl Pts',(-50.5113921507918,-75.1163956227987,
63.3025446990746));
#204156=CARTESIAN_POINT('Ctrl Pts',(-50.5421483544675,-75.8504591731212,
62.4416229161422));
#204157=CARTESIAN_POINT('Ctrl Pts',(-50.5931362890706,-77.2260936162112,
61.2813551912261));
#204158=CARTESIAN_POINT('Ctrl Pts',(-50.6124378411332,-77.7845151191548,
60.8977936531863));
#204159=CARTESIAN_POINT('Ctrl Pts',(-50.6501790766711,-78.9678990253529,
60.2466336853813));
#204160=CARTESIAN_POINT('Ctrl Pts',(-50.6689114356124,-79.5898722357642,
59.9804704590923));
#204161=CARTESIAN_POINT('Ctrl Pts',(-50.702648826188,-80.7262240909296,
59.6218847490626));
#204162=CARTESIAN_POINT('Ctrl Pts',(-50.7174214577686,-81.2300224633969,
59.5038756888092));
#204163=CARTESIAN_POINT('Ctrl Pts',(-50.7413547345326,-82.0681130272073,
59.3733398517201));
#204164=CARTESIAN_POINT('Ctrl Pts',(-50.7505851433636,-82.3979440931124,
59.3382428579476));
#204165=CARTESIAN_POINT('Ctrl Pts',(-50.7975213204536,-84.0782644435076,
59.2415055227305));
#204166=CARTESIAN_POINT('Ctrl Pts',(-50.8360007821808,-85.4297666425667,
59.431481709767));
#204167=CARTESIAN_POINT('Ctrl Pts',(-50.9113416243312,-87.9796635714467,
60.3243343480095));
#204168=CARTESIAN_POINT('Ctrl Pts',(-50.9497759551382,-89.1532807598111,
61.0179025958922));
#204169=CARTESIAN_POINT('Ctrl Pts',(-51.0047808895068,-90.6220228361453,
62.3341359280561));
#204170=CARTESIAN_POINT('Ctrl Pts',(-51.0221410764558,-91.0465650538621,
62.7906518478815));
#204171=CARTESIAN_POINT('Ctrl Pts',(-51.0542450765868,-91.7390711980155,
63.6863618893484));
#204172=CARTESIAN_POINT('Ctrl Pts',(-51.0688308864644,-92.0204998589996,
64.1126185471536));
#204173=CARTESIAN_POINT('Ctrl Pts',(-51.1022187659112,-92.5987553498626,
65.1490151296931));
#204174=CARTESIAN_POINT('Ctrl Pts',(-51.1208774390134,-92.8691501617716,
65.7711860632802));
#204175=CARTESIAN_POINT('Ctrl Pts',(-51.1548729987492,-93.2384272103452,
66.9199684144007));
#204176=CARTESIAN_POINT('Ctrl Pts',(-51.1699759240403,-93.3612329273738,
67.4362989395747));
#204177=CARTESIAN_POINT('Ctrl Pts',(-51.2117835909394,-93.5900395746801,
68.8911604270237));
#204178=CARTESIAN_POINT('Ctrl Pts',(-51.2375992875248,-93.6073154449516,
69.8382887136524));
#204179=CARTESIAN_POINT('Ctrl Pts',(-51.2824202947345,-93.4183243877577,
71.4120497051439));
#204180=CARTESIAN_POINT('Ctrl Pts',(-51.3008195271194,-93.281981828787,
72.0411193268221));
#204181=CARTESIAN_POINT('Ctrl Pts',(-51.332914609746,-92.9358387018392,
73.1316242487575));
#204182=CARTESIAN_POINT('Ctrl Pts',(-51.3468118683534,-92.7490800421751,
73.5981691204317));
#204183=CARTESIAN_POINT('Ctrl Pts',(-51.3702006408016,-92.3831290921145,
74.3477352292558));
#204184=CARTESIAN_POINT('Ctrl Pts',(-51.3795720312957,-92.2229254887043,
74.6390500290059));
#204185=CARTESIAN_POINT('Ctrl Pts',(-51.402509724984,-91.7993587266667,
75.3277306857764));
#204186=CARTESIAN_POINT('Ctrl Pts',(-51.4161202137027,-91.521889929389,
75.7155119559237));
#204187=CARTESIAN_POINT('Ctrl Pts',(-51.4429325966705,-90.9153420781408,
76.4493165723929));
#204188=CARTESIAN_POINT('Ctrl Pts',(-51.4561078238969,-90.5870482648257,
76.7944913293652));
#204189=CARTESIAN_POINT('Ctrl Pts',(-51.48756500931,-89.7569663312927,77.5537380621301));
#204190=CARTESIAN_POINT('Ctrl Pts',(-51.5059390037133,-89.2374296711775,
77.9453668480806));
#204191=CARTESIAN_POINT('Ctrl Pts',(-51.533918319714,-88.3993095355104,
78.4603850334184));
#204192=CARTESIAN_POINT('Ctrl Pts',(-51.5434030417083,-88.105845456195,
78.621489376031));
#204193=CARTESIAN_POINT('Ctrl Pts',(-51.5729128059786,-87.1587681226295,
79.0826086526193));
#204194=CARTESIAN_POINT('Ctrl Pts',(-51.5927914031008,-86.4812026847779,
79.3284127140952));
#204195=CARTESIAN_POINT('Ctrl Pts',(-51.6274224279696,-85.2930522074634,
79.6228502185749));
#204196=CARTESIAN_POINT('Ctrl Pts',(-51.6418592851651,-84.7942755429739,
79.7079580210748));
#204197=CARTESIAN_POINT('Ctrl Pts',(-51.6735664554767,-83.6780138171301,
79.8144286227466));
#204198=CARTESIAN_POINT('Ctrl Pts',(-51.6905597091711,-83.0607405314188,
79.8175173393461));
#204199=CARTESIAN_POINT('Ctrl Pts',(-51.7267421582604,-81.7746480406731,
79.7078230825936));
#204200=CARTESIAN_POINT('Ctrl Pts',(-51.7459449176401,-81.1096667916172,
79.5842398510074));
#204201=CARTESIAN_POINT('Ctrl Pts',(-51.7941678793656,-79.4778033105092,
79.110735851032));
#204202=CARTESIAN_POINT('Ctrl Pts',(-51.822180689247,-78.542268924523,78.6793590613686));
#204203=CARTESIAN_POINT('Ctrl Pts',(-51.8681523662406,-77.1877831947701,
77.7886683778086));
#204204=CARTESIAN_POINT('Ctrl Pts',(-51.8852020986695,-76.7188368099212,
77.4179469190336));
#204205=CARTESIAN_POINT('Ctrl Pts',(-51.9241413640814,-75.7069031604261,
76.4634318958915));
#204206=CARTESIAN_POINT('Ctrl Pts',(-51.9461415253868,-75.1943307168622,
75.8529811569711));
#204207=CARTESIAN_POINT('Ctrl Pts',(-51.9865585514724,-74.4108924845377,
74.6632671062139));
#204208=CARTESIAN_POINT('Ctrl Pts',(-52.0045251918746,-74.1136240030923,
74.1062078376817));
#204209=CARTESIAN_POINT('Ctrl Pts',(-52.0227265417637,-73.8611037358073,
73.5056828137199));
#204210=CARTESIAN_POINT('Ctrl Pts',(-52.0233235296543,-73.8528803082147,
73.4859539635495));
#204211=CARTESIAN_POINT('Ctrl Pts',(-52.0239203182307,-73.8447192555915,
73.4662010264956));
#204212=CARTESIAN_POINT('Ctrl Pts',(-51.6180871401245,-73.8447192590796,
73.4662010349383));
#204213=CARTESIAN_POINT('Ctrl Pts',(-51.6088680289194,-73.9695775786798,
73.7684069678417));
#204214=CARTESIAN_POINT('Ctrl Pts',(-51.5995742687078,-74.1090451023638,
74.0649984361503));
#204215=CARTESIAN_POINT('Ctrl Pts',(-51.5808374449442,-74.4176933519959,
74.6469431862595));
#204216=CARTESIAN_POINT('Ctrl Pts',(-51.5714221024677,-74.5866248525164,
74.9313253023218));
#204217=CARTESIAN_POINT('Ctrl Pts',(-51.5488062304926,-75.0295876819302,
75.6010035997114));
#204218=CARTESIAN_POINT('Ctrl Pts',(-51.535725037155,-75.3170941776685,
75.9764790508954));
#204219=CARTESIAN_POINT('Ctrl Pts',(-51.5132824279099,-75.8479256737056,
76.5785740598815));
#204220=CARTESIAN_POINT('Ctrl Pts',(-51.5040042629682,-76.0782335248933,
76.8156532917978));
#204221=CARTESIAN_POINT('Ctrl Pts',(-51.4804745108094,-76.6859979262158,
77.3836101134934));
#204222=CARTESIAN_POINT('Ctrl Pts',(-51.4661488559317,-77.0770455482743,
77.6986695192962));
#204223=CARTESIAN_POINT('Ctrl Pts',(-51.433710034848,-78.0202762089417,
78.3506896419294));
#204224=CARTESIAN_POINT('Ctrl Pts',(-51.4159271820186,-78.584424246117,
78.6666178546337));
#204225=CARTESIAN_POINT('Ctrl Pts',(-51.3715379735554,-80.0317792974971,
79.3062993131463));
#204226=CARTESIAN_POINT('Ctrl Pts',(-51.3446502820813,-80.9369703855401,
79.5658141301405));
#204227=CARTESIAN_POINT('Ctrl Pts',(-51.304010833661,-82.3760421333811,
79.7719296091203));
#204228=CARTESIAN_POINT('Ctrl Pts',(-51.2896814831992,-82.8921232634512,
79.8064094839421));
#204229=CARTESIAN_POINT('Ctrl Pts',(-51.2561239832045,-84.0848126465833,
79.7958694853764));
#204230=CARTESIAN_POINT('Ctrl Pts',(-51.2367826235284,-84.7587699279815,
79.7229893473125));
#204231=CARTESIAN_POINT('Ctrl Pts',(-51.2020429532851,-85.9627283515491,
79.4706534872351));
#204232=CARTESIAN_POINT('Ctrl Pts',(-51.1867385626414,-86.4947373285883,
79.3132787849589));
#204233=CARTESIAN_POINT('Ctrl Pts',(-51.1397423175928,-88.0607289081945,
78.7083671943219));
#204234=CARTESIAN_POINT('Ctrl Pts',(-51.1075807679138,-89.0361904333139,
78.1330603498034));
#204235=CARTESIAN_POINT('Ctrl Pts',(-51.0578986311202,-90.4020450773067,
76.9893310403567));
#204236=CARTESIAN_POINT('Ctrl Pts',(-51.0395561058025,-90.863790620292,
76.5203866193077));
#204237=CARTESIAN_POINT('Ctrl Pts',(-51.0029816279645,-91.675537924791,
75.5199506099501));
#204238=CARTESIAN_POINT('Ctrl Pts',(-50.9849985245908,-92.0273794945852,
74.9936318724835));
#204239=CARTESIAN_POINT('Ctrl Pts',(-50.949530423408,-92.6329030547024,
73.8769649768003));
#204240=CARTESIAN_POINT('Ctrl Pts',(-50.9317844359032,-92.8841638273681,
73.2884379965072));
#204241=CARTESIAN_POINT('Ctrl Pts',(-50.8990848004757,-93.2367409953333,
72.1882560767215));
#204242=CARTESIAN_POINT('Ctrl Pts',(-50.8843122210643,-93.3570080036304,
71.6849187868307));
#204243=CARTESIAN_POINT('Ctrl Pts',(-50.8543688558147,-93.5248753284648,
70.6377495403507));
#204244=CARTESIAN_POINT('Ctrl Pts',(-50.8393398806685,-93.5680841921314,
70.0948338660248));
#204245=CARTESIAN_POINT('Ctrl Pts',(-50.7920614820175,-93.5678887198971,
68.4056658668837));
#204246=CARTESIAN_POINT('Ctrl Pts',(-50.7593317019474,-93.3757688773966,
67.2683584434087));
#204247=CARTESIAN_POINT('Ctrl Pts',(-50.6897094276442,-92.5559597270763,
64.9101762264595));
#204248=CARTESIAN_POINT('Ctrl Pts',(-50.651244773498,-91.8642330778891,
63.7341197715842));
#204249=CARTESIAN_POINT('Ctrl Pts',(-50.5952993305559,-90.5283527393984,
62.2377214259173));
#204250=CARTESIAN_POINT('Ctrl Pts',(-50.5770222587136,-90.0465525155411,
61.7922196472051));
#204251=CARTESIAN_POINT('Ctrl Pts',(-50.5405414684501,-89.0236613067167,
61.0137450018216));
#204252=CARTESIAN_POINT('Ctrl Pts',(-50.5225693444161,-88.4875600718011,
60.6789031349042));
#204253=CARTESIAN_POINT('Ctrl Pts',(-50.4872101825288,-87.3566336744448,
60.1100214718486));
#204254=CARTESIAN_POINT('Ctrl Pts',(-50.4695694709475,-86.7638732376919,
59.8779451961286));
#204255=CARTESIAN_POINT('Ctrl Pts',(-50.4373797327673,-85.6703517985294,
59.5631628233311));
#204256=CARTESIAN_POINT('Ctrl Pts',(-50.4230182927863,-85.1776707837086,
59.4598259614579));
#204257=CARTESIAN_POINT('Ctrl Pts',(-50.3908246801374,-84.0495941544247,
59.3086580637835));
#204258=CARTESIAN_POINT('Ctrl Pts',(-50.3733051002074,-83.4133024216528,
59.2830095979889));
#204259=CARTESIAN_POINT('Ctrl Pts',(-50.3286408184093,-81.8229071678612,
59.366800535251));
#204260=CARTESIAN_POINT('Ctrl Pts',(-50.3011872547787,-80.8788235245975,
59.5507967074688));
#204261=CARTESIAN_POINT('Ctrl Pts',(-50.2585181496259,-79.4353698362872,
60.0489707053046));
#204262=CARTESIAN_POINT('Ctrl Pts',(-50.2427049380204,-78.9131522289264,
60.2794712754771));
#204263=CARTESIAN_POINT('Ctrl Pts',(-50.2012185078618,-77.6216584887111,
60.98336079612));
#204264=CARTESIAN_POINT('Ctrl Pts',(-50.1754966749369,-76.8908060720885,
61.51699453351));
#204265=CARTESIAN_POINT('Ctrl Pts',(-50.1321267801252,-75.7662093542935,
62.5909022123853));
#204266=CARTESIAN_POINT('Ctrl Pts',(-50.1138751742358,-75.337562903395,
63.0867648717513));
#204267=CARTESIAN_POINT('Ctrl Pts',(-50.0774292702906,-74.5942431474175,
64.1341646722153));
#204268=CARTESIAN_POINT('Ctrl Pts',(-50.0594601022904,-74.2775987983706,
64.6808305870127));
#204269=CARTESIAN_POINT('Ctrl Pts',(-50.0245970747622,-73.7541488071094,
65.8137609433811));
#204270=CARTESIAN_POINT('Ctrl Pts',(-50.0074507095344,-73.5463136479135,
66.396670831945));
#204271=CARTESIAN_POINT('Ctrl Pts',(-49.9762190900313,-73.2706174739045,
67.4666577787987));
#204272=CARTESIAN_POINT('Ctrl Pts',(-49.9623096670931,-73.182831640914,
67.9466531175065));
#204273=CARTESIAN_POINT('Ctrl Pts',(-49.9260721432976,-73.0429598345648,
69.2177099815939));
#204274=CARTESIAN_POINT('Ctrl Pts',(-49.9043390259112,-73.0477888731545,
70.0117339440578));
#204275=CARTESIAN_POINT('Ctrl Pts',(-49.8629742368981,-73.2261677555999,
71.4694146974536));
#204276=CARTESIAN_POINT('Ctrl Pts',(-49.8435831292548,-73.3748234753399,
72.1317511881231));
#204277=CARTESIAN_POINT('Ctrl Pts',(-49.8175643780153,-73.6650694216188,
73.0081948368761));
#204278=CARTESIAN_POINT('Ctrl Pts',(-49.8106963345261,-73.7508026049707,
73.238886025726));
#204279=CARTESIAN_POINT('Ctrl Pts',(-49.8038356726598,-73.8447192590796,
73.4662010349383));
#204280=CARTESIAN_POINT('Origin',(-45.8894114130409,-83.3180213346267,69.5522455184007));
#204281=CARTESIAN_POINT('',(-53.8378263131057,-73.8447192590796,73.4662010349383));
#204282=CARTESIAN_POINT('',(-53.4317936414903,-73.8447192595573,73.4662010360945));
#204283=CARTESIAN_POINT('',(-45.8894114130409,-73.8447192590796,73.4662010349383));
#204284=CARTESIAN_POINT('Ctrl Pts',(-52.0239203182307,-73.8447192555915,
73.4662010264956));
#204285=CARTESIAN_POINT('Ctrl Pts',(-52.0422770133231,-73.5936924086256,
72.858617944282));
#204286=CARTESIAN_POINT('Ctrl Pts',(-52.0605483749575,-73.4016808879974,
72.228248441614));
#204287=CARTESIAN_POINT('Ctrl Pts',(-52.0942628704608,-73.1657213497129,
71.0613550323591));
#204288=CARTESIAN_POINT('Ctrl Pts',(-52.1095099790986,-73.1009902501868,
70.531469726697));
#204289=CARTESIAN_POINT('Ctrl Pts',(-52.1377410759291,-73.0573142951046,
69.5302680403876));
#204290=CARTESIAN_POINT('Ctrl Pts',(-52.1507348460864,-73.0690701400119,
69.060720889055));
#204291=CARTESIAN_POINT('Ctrl Pts',(-52.173186689646,-73.1441802615669,
68.2611238726265));
#204292=CARTESIAN_POINT('Ctrl Pts',(-52.1825655151234,-73.1916465457803,
67.9303426470445));
#204293=CARTESIAN_POINT('Ctrl Pts',(-52.2061708075939,-73.3503948751928,
67.1110373782177));
#204294=CARTESIAN_POINT('Ctrl Pts',(-52.2204692031783,-73.4814864543216,
66.6272407659104));
#204295=CARTESIAN_POINT('Ctrl Pts',(-52.2531015148368,-73.8637581996122,
65.5390745711569));
#204296=CARTESIAN_POINT('Ctrl Pts',(-52.2710912133515,-74.1384598613343,
64.9452632469345));
#204297=CARTESIAN_POINT('Ctrl Pts',(-52.3083462598444,-74.8082876769875,
63.7987580593691));
#204298=CARTESIAN_POINT('Ctrl Pts',(-52.3275847766853,-75.205561491599,
63.2509628073172));
#204299=CARTESIAN_POINT('Ctrl Pts',(-52.3708968886107,-76.2199062240943,
62.1087133425954));
#204300=CARTESIAN_POINT('Ctrl Pts',(-52.3942780319818,-76.8633589762556,
61.544327886537));
#204301=CARTESIAN_POINT('Ctrl Pts',(-52.4439230593988,-78.3198530270727,
60.557645931314));
#204302=CARTESIAN_POINT('Ctrl Pts',(-52.4697754954037,-79.1346429520161,
60.1509757586101));
#204303=CARTESIAN_POINT('Ctrl Pts',(-52.5133928595621,-80.6140705410418,
59.64349633463));
#204304=CARTESIAN_POINT('Ctrl Pts',(-52.5317625923539,-81.2549684453486,
59.4905128716933));
#204305=CARTESIAN_POINT('Ctrl Pts',(-52.5683778176634,-82.532282188248,
59.3128694076042));
#204306=CARTESIAN_POINT('Ctrl Pts',(-52.5863670039881,-83.1652054050903,
59.283902231493));
#204307=CARTESIAN_POINT('Ctrl Pts',(-52.6218833432031,-84.435990751974,
59.3433199942979));
#204308=CARTESIAN_POINT('Ctrl Pts',(-52.6396741231847,-85.0710214742086,
59.4330062849073));
#204309=CARTESIAN_POINT('Ctrl Pts',(-52.6726137453752,-86.2028426545355,
59.7026552256781));
#204310=CARTESIAN_POINT('Ctrl Pts',(-52.6875849700365,-86.7021081484069,
59.8628401268524));
#204311=CARTESIAN_POINT('Ctrl Pts',(-52.7167190063917,-87.65853629047,60.2526874831467));
#204312=CARTESIAN_POINT('Ctrl Pts',(-52.7308076230974,-88.1151488521579,
60.4797915353621));
#204313=CARTESIAN_POINT('Ctrl Pts',(-52.7624829229541,-89.0887049844133,
61.0581310247888));
#204314=CARTESIAN_POINT('Ctrl Pts',(-52.7801173891084,-89.5942839773548,
61.4245592008917));
#204315=CARTESIAN_POINT('Ctrl Pts',(-52.8362453338733,-91.079955018231,
62.7230769619799));
#204316=CARTESIAN_POINT('Ctrl Pts',(-52.8731268851787,-91.9109898122703,
63.8036767077062));
#204317=CARTESIAN_POINT('Ctrl Pts',(-52.9499845296873,-93.1071166812942,
66.2261390180689));
#204318=CARTESIAN_POINT('Ctrl Pts',(-52.986907153841,-93.4599413377088,
67.5445518777276));
#204319=CARTESIAN_POINT('Ctrl Pts',(-53.0347878919167,-93.5681338346198,
69.2242163121293));
#204320=CARTESIAN_POINT('Ctrl Pts',(-53.0442240638684,-93.5733808590658,
69.5558979227205));
#204321=CARTESIAN_POINT('Ctrl Pts',(-53.0681128435813,-93.5456188232973,
70.4048654754654));
#204322=CARTESIAN_POINT('Ctrl Pts',(-53.0824397629106,-93.4894872847451,
70.9204549018704));
#204323=CARTESIAN_POINT('Ctrl Pts',(-53.1266209662051,-93.2006489952452,
72.4707885674772));
#204324=CARTESIAN_POINT('Ctrl Pts',(-53.1569471242125,-92.8464568547865,
73.4756555819651));
#204325=CARTESIAN_POINT('Ctrl Pts',(-53.1956975694565,-92.1884187399158,
74.6988304708029));
#204326=CARTESIAN_POINT('Ctrl Pts',(-53.2048792607579,-92.0182280079635,
74.981581587507));
#204327=CARTESIAN_POINT('Ctrl Pts',(-53.2330373667578,-91.4592599313037,
75.8162701146337));
#204328=CARTESIAN_POINT('Ctrl Pts',(-53.2522385332535,-91.0293762727016,
76.3384637818322));
#204329=CARTESIAN_POINT('Ctrl Pts',(-53.3008563819609,-89.8156874020234,
77.5472951144627));
#204330=CARTESIAN_POINT('Ctrl Pts',(-53.3292423807927,-88.9729888883224,
78.1639715288605));
#204331=CARTESIAN_POINT('Ctrl Pts',(-53.3762905115393,-87.5019766114925,
78.9299701749641));
#204332=CARTESIAN_POINT('Ctrl Pts',(-53.3939907626489,-86.9269766557998,
79.1659159521151));
#204333=CARTESIAN_POINT('Ctrl Pts',(-53.4258660672702,-85.8371802711613,
79.5014547760017));
#204334=CARTESIAN_POINT('Ctrl Pts',(-53.440293462899,-85.3292546008724,
79.6164328858441));
#204335=CARTESIAN_POINT('Ctrl Pts',(-53.473959533795,-84.1456861017741,
79.7911392171768));
#204336=CARTESIAN_POINT('Ctrl Pts',(-53.493308172292,-83.46844100145,79.8234349761715));
#204337=CARTESIAN_POINT('Ctrl Pts',(-53.5276985212792,-82.2519364355357,
79.7610384134673));
#204338=CARTESIAN_POINT('Ctrl Pts',(-53.542672354733,-81.7139511536507,
79.6904382341201));
#204339=CARTESIAN_POINT('Ctrl Pts',(-53.5900109002638,-80.0596313329246,
79.3383093961517));
#204340=CARTESIAN_POINT('Ctrl Pts',(-53.6228577484491,-78.983432082236,
78.9114915684615));
#204341=CARTESIAN_POINT('Ctrl Pts',(-53.6926017569744,-76.8452963902698,
77.6140401558868));
#204342=CARTESIAN_POINT('Ctrl Pts',(-53.7310713831788,-75.8399591963833,
76.691383828323));
#204343=CARTESIAN_POINT('Ctrl Pts',(-53.7870357222705,-74.6559146677685,
75.0712859410944));
#204344=CARTESIAN_POINT('Ctrl Pts',(-53.805332611289,-74.3208843648723,
74.5063768204541));
#204345=CARTESIAN_POINT('Ctrl Pts',(-53.8285582294811,-73.9727193494954,
73.7658432035555));
#204346=CARTESIAN_POINT('Ctrl Pts',(-53.8331925250674,-73.9069169167772,
73.6167436758221));
#204347=CARTESIAN_POINT('Ctrl Pts',(-53.8378263131057,-73.8447192590796,
73.4662010349383));
#204348=CARTESIAN_POINT('Ctrl Pts',(-53.4317936414903,-73.844719260035,
73.4662010372508));
#204349=CARTESIAN_POINT('Ctrl Pts',(-53.4314659960779,-73.8491222862514,
73.4768580815603));
#204350=CARTESIAN_POINT('Ctrl Pts',(-53.4311383816884,-73.8535434612602,
73.4875080972125));
#204351=CARTESIAN_POINT('Ctrl Pts',(-53.4128952710928,-74.1007721347706,
74.0802219304168));
#204352=CARTESIAN_POINT('Ctrl Pts',(-53.3954072228787,-74.3967639325128,
74.6386413478996));
#204353=CARTESIAN_POINT('Ctrl Pts',(-53.3594844786823,-75.1007300517108,
75.7139927044221));
#204354=CARTESIAN_POINT('Ctrl Pts',(-53.3409746455454,-75.5109043610059,
76.226068551973));
#204355=CARTESIAN_POINT('Ctrl Pts',(-53.2839183522462,-76.9087607598518,
77.6645611460637));
#204356=CARTESIAN_POINT('Ctrl Pts',(-53.2470045192626,-78.0328192134182,
78.4379034484896));
#204357=CARTESIAN_POINT('Ctrl Pts',(-53.1760057253269,-80.3261415055106,
79.4224570102882));
#204358=CARTESIAN_POINT('Ctrl Pts',(-53.1446794675631,-81.446073105076,
79.6946439377546));
#204359=CARTESIAN_POINT('Ctrl Pts',(-53.0968240154838,-83.130495291176,
79.8149681958114));
#204360=CARTESIAN_POINT('Ctrl Pts',(-53.0812542410853,-83.6755298664529,
79.8104536842918));
#204361=CARTESIAN_POINT('Ctrl Pts',(-53.0514361457815,-84.7323198864851,
79.7173440421182));
#204362=CARTESIAN_POINT('Ctrl Pts',(-53.0371402952389,-85.2428522259182,
79.6331432599799));
#204363=CARTESIAN_POINT('Ctrl Pts',(-53.0022205705578,-86.4535301974657,
79.3381092417562));
#204364=CARTESIAN_POINT('Ctrl Pts',(-52.9814285047545,-87.1417473880965,
79.0902559042181));
#204365=CARTESIAN_POINT('Ctrl Pts',(-52.9512840399917,-88.0988145283276,
78.6252011401997));
#204366=CARTESIAN_POINT('Ctrl Pts',(-52.941924293927,-88.3924870962548,
78.4642770171724));
#204367=CARTESIAN_POINT('Ctrl Pts',(-52.9143597158262,-89.2348059345622,
77.9475554461033));
#204368=CARTESIAN_POINT('Ctrl Pts',(-52.8961354568488,-89.7578902781713,
77.5533485346869));
#204369=CARTESIAN_POINT('Ctrl Pts',(-52.8641346519024,-90.5899246708746,
76.7915263111902));
#204370=CARTESIAN_POINT('Ctrl Pts',(-52.8505713097731,-90.9172918257617,
76.447087942484));
#204371=CARTESIAN_POINT('Ctrl Pts',(-52.8238139978604,-91.5221729799957,
75.7150387416953));
#204372=CARTESIAN_POINT('Ctrl Pts',(-52.8106602608981,-91.7989167849175,
75.3282771916983));
#204373=CARTESIAN_POINT('Ctrl Pts',(-52.7880664001755,-92.2224186552218,
74.63999416063));
#204374=CARTESIAN_POINT('Ctrl Pts',(-52.7787101072541,-92.3830593056323,
74.347927168135));
#204375=CARTESIAN_POINT('Ctrl Pts',(-52.7550857351594,-92.7494153707999,
73.5974083153159));
#204376=CARTESIAN_POINT('Ctrl Pts',(-52.7407446071526,-92.936195309577,
73.1306895624725));
#204377=CARTESIAN_POINT('Ctrl Pts',(-52.7084130093085,-93.2818563157177,
72.0412732352165));
#204378=CARTESIAN_POINT('Ctrl Pts',(-52.6907451184266,-93.4179637838621,
71.4135437556393));
#204379=CARTESIAN_POINT('Ctrl Pts',(-52.6462484222971,-93.607556126628,
69.8385019542383));
#204380=CARTESIAN_POINT('Ctrl Pts',(-52.6191261781122,-93.5901249332605,
68.8886457121736));
#204381=CARTESIAN_POINT('Ctrl Pts',(-52.577694997278,-93.3590903377669,
67.4244244110862));
#204382=CARTESIAN_POINT('Ctrl Pts',(-52.5628004969001,-93.23389135412,66.9015454393607));
#204383=CARTESIAN_POINT('Ctrl Pts',(-52.5286159492089,-92.8595098718149,
65.7468748805531));
#204384=CARTESIAN_POINT('Ctrl Pts',(-52.5092323715447,-92.5874114302617,
65.1251422778849));
#204385=CARTESIAN_POINT('Ctrl Pts',(-52.4763357891662,-92.0161993105707,
64.1075959626971));
#204386=CARTESIAN_POINT('Ctrl Pts',(-52.4627751968757,-91.7460663408475,
63.6981383524777));
#204387=CARTESIAN_POINT('Ctrl Pts',(-52.4309630398125,-91.0532107862128,
62.7958510848964));
#204388=CARTESIAN_POINT('Ctrl Pts',(-52.412630142182,-90.6109278293944,
62.3206812572907));
#204389=CARTESIAN_POINT('Ctrl Pts',(-52.384692694973,-89.8767155914402,
61.6682144442994));
#204390=CARTESIAN_POINT('Ctrl Pts',(-52.3752083043004,-89.6159179377135,
61.4583639230839));
#204391=CARTESIAN_POINT('Ctrl Pts',(-52.3457945902119,-88.7667206818431,
60.8409941032593));
#204392=CARTESIAN_POINT('Ctrl Pts',(-52.326011970883,-88.1456699508842,
60.4820724973368));
#204393=CARTESIAN_POINT('Ctrl Pts',(-52.2915787964989,-87.0339097740575,
59.986337237425));
#204394=CARTESIAN_POINT('Ctrl Pts',(-52.2772408043858,-86.5611004650484,
59.8158774709484));
#204395=CARTESIAN_POINT('Ctrl Pts',(-52.2448876251276,-85.4596461536221,
59.507953321651));
#204396=CARTESIAN_POINT('Ctrl Pts',(-52.22719657544,-84.8267186286824,59.3935941724937));
#204397=CARTESIAN_POINT('Ctrl Pts',(-52.1827229976503,-83.2468765253718,
59.2591326613441));
#204398=CARTESIAN_POINT('Ctrl Pts',(-52.1556494608471,-82.2999282653714,
59.3093587972093));
#204399=CARTESIAN_POINT('Ctrl Pts',(-52.1143881262755,-80.8505356441113,
59.5894406872827));
#204400=CARTESIAN_POINT('Ctrl Pts',(-52.0996164496285,-80.336457153583,
59.7310317134483));
#204401=CARTESIAN_POINT('Ctrl Pts',(-52.0655683723267,-79.1991284312426,
60.141861162038));
#204402=CARTESIAN_POINT('Ctrl Pts',(-52.046193967924,-78.5868929144694,
60.4342949386094));
#204403=CARTESIAN_POINT('Ctrl Pts',(-52.0129298437869,-77.5780295802241,
61.045327815706));
#204404=CARTESIAN_POINT('Ctrl Pts',(-51.9990216839351,-77.1678265296377,
61.3369998056442));
#204405=CARTESIAN_POINT('Ctrl Pts',(-51.9673054134062,-76.2944334305258,
62.0602316501973));
#204406=CARTESIAN_POINT('Ctrl Pts',(-51.9494382097905,-75.8464292686363,
62.5069380626748));
#204407=CARTESIAN_POINT('Ctrl Pts',(-51.8930940259451,-74.5786579956985,
64.0289113611284));
#204408=CARTESIAN_POINT('Ctrl Pts',(-51.8562261691269,-73.9281584556253,
65.2262591381618));
#204409=CARTESIAN_POINT('Ctrl Pts',(-51.7793863201825,-73.1278341473228,
67.8060293697946));
#204410=CARTESIAN_POINT('Ctrl Pts',(-51.7424659278239,-72.9866121356817,
69.1634381986777));
#204411=CARTESIAN_POINT('Ctrl Pts',(-51.674918110725,-73.2082696381617,
71.527539235845));
#204412=CARTESIAN_POINT('Ctrl Pts',(-51.6468253702287,-73.4555052622732,
72.5241510427503));
#204413=CARTESIAN_POINT('Ctrl Pts',(-51.6180871401245,-73.8447192590796,
73.4662010349383));
#204414=CARTESIAN_POINT('Origin',(-45.8894114130409,-83.3180213346267,69.5522455184007));
#204415=CARTESIAN_POINT('',(-55.6519493945588,-73.8447192590796,73.4662010349383));
#204416=CARTESIAN_POINT('',(-55.2458788381492,-73.8447192608157,73.4662010391402));
#204417=CARTESIAN_POINT('',(-45.8894114130409,-73.8447192590796,73.4662010349383));
#204418=CARTESIAN_POINT('',(-54.9945874883696,-92.4407690432347,74.2253573558264));
#204419=CARTESIAN_POINT('Ctrl Pts',(-54.9945936623312,-92.4407691206747,
74.2253572046497));
#204420=CARTESIAN_POINT('Ctrl Pts',(-55.0066649201741,-92.2433966771307,
74.6106634295504));
#204421=CARTESIAN_POINT('Ctrl Pts',(-55.0187555319245,-92.0218130116692,
74.9830764195218));
#204422=CARTESIAN_POINT('Ctrl Pts',(-55.0429782090374,-91.5373152573875,
75.6911698136988));
#204423=CARTESIAN_POINT('Ctrl Pts',(-55.0550815346248,-91.2756917979126,
76.0267078005093));
#204424=CARTESIAN_POINT('Ctrl Pts',(-55.0899110882135,-90.4637607069585,
76.944205363172));
#204425=CARTESIAN_POINT('Ctrl Pts',(-55.1119688536957,-89.8651910287765,
77.4792395854887));
#204426=CARTESIAN_POINT('Ctrl Pts',(-55.1495375466645,-88.770245468781,
78.248524598755));
#204427=CARTESIAN_POINT('Ctrl Pts',(-55.1648147582145,-88.3063051566961,
78.522698919535));
#204428=CARTESIAN_POINT('Ctrl Pts',(-55.2055978337842,-87.018110709541,
79.1530156806458));
#204429=CARTESIAN_POINT('Ctrl Pts',(-55.2302546487337,-86.1650441718704,
79.4396070179568));
#204430=CARTESIAN_POINT('Ctrl Pts',(-55.2783996876088,-84.4858971272087,
79.7680474707867));
#204431=CARTESIAN_POINT('Ctrl Pts',(-55.3017789764987,-83.6703563978136,
79.8285489547887));
#204432=CARTESIAN_POINT('Ctrl Pts',(-55.3434912289675,-82.1819265079146,
79.761431518673));
#204433=CARTESIAN_POINT('Ctrl Pts',(-55.3621760200869,-81.5122159206528,
79.6644786670884));
#204434=CARTESIAN_POINT('Ctrl Pts',(-55.3999714383141,-80.2140361905615,
79.3433819460147));
#204435=CARTESIAN_POINT('Ctrl Pts',(-55.4189476524304,-79.5880784923225,
79.1224394238562));
#204436=CARTESIAN_POINT('Ctrl Pts',(-55.4515257106814,-78.5351379874725,
78.6316709205173));
#204437=CARTESIAN_POINT('Ctrl Pts',(-55.4653579824756,-78.0984814130689,
78.3878747900162));
#204438=CARTESIAN_POINT('Ctrl Pts',(-55.4993518147926,-77.0860228121406,
77.7212560786378));
#204439=CARTESIAN_POINT('Ctrl Pts',(-55.5196795163116,-76.5332138955025,
77.2682618098607));
#204440=CARTESIAN_POINT('Ctrl Pts',(-55.556419597369,-75.6208619052758,
76.3461951921266));
#204441=CARTESIAN_POINT('Ctrl Pts',(-55.5725755041761,-75.2461089869606,
75.8963961645671));
#204442=CARTESIAN_POINT('Ctrl Pts',(-55.6097438652591,-74.4859060044505,
74.8067753415515));
#204443=CARTESIAN_POINT('Ctrl Pts',(-55.6308775706893,-74.1282814057265,
74.152532256902));
#204444=CARTESIAN_POINT('Ctrl Pts',(-55.6519493945588,-73.8447192590796,
73.4662010349383));
#204445=CARTESIAN_POINT('Ctrl Pts',(-53.8378263131057,-73.8447192590796,
73.4662010349383));
#204446=CARTESIAN_POINT('Ctrl Pts',(-53.8511289913648,-73.6661622292858,
73.034023235829));
#204447=CARTESIAN_POINT('Ctrl Pts',(-53.8643689226581,-73.5173135352037,
72.5899503891903));
#204448=CARTESIAN_POINT('Ctrl Pts',(-53.8952071739069,-73.2388572589834,
71.5214345218071));
#204449=CARTESIAN_POINT('Ctrl Pts',(-53.9128793880311,-73.1360869876221,
70.8921947571121));
#204450=CARTESIAN_POINT('Ctrl Pts',(-53.9452141595788,-73.0574520151227,
69.7520446546323));
#204451=CARTESIAN_POINT('Ctrl Pts',(-53.9596908591394,-73.060116320017,
69.2447001582753));
#204452=CARTESIAN_POINT('Ctrl Pts',(-53.9911563796819,-73.1483514527247,
68.1352280525231));
#204453=CARTESIAN_POINT('Ctrl Pts',(-54.0078860100975,-73.2499536620984,
67.5362743482051));
#204454=CARTESIAN_POINT('Ctrl Pts',(-54.0538873493735,-73.6666986665519,
65.9486543020002));
#204455=CARTESIAN_POINT('Ctrl Pts',(-54.0835374881285,-74.0796424871106,
64.9930500366725));
#204456=CARTESIAN_POINT('Ctrl Pts',(-54.1216000517381,-74.8031229615294,
63.8367233665558));
#204457=CARTESIAN_POINT('Ctrl Pts',(-54.1307538091373,-74.9909046909345,
63.5664443345819));
#204458=CARTESIAN_POINT('Ctrl Pts',(-54.1695655229798,-75.835137602131,
62.4681159636899));
#204459=CARTESIAN_POINT('Ctrl Pts',(-54.199814925981,-76.604543554259,61.7351064166373));
#204460=CARTESIAN_POINT('Ctrl Pts',(-54.2384870978,-77.7431291443887,60.9445863880131));
#204461=CARTESIAN_POINT('Ctrl Pts',(-54.2476655873979,-78.0228892527884,
60.7697177274664));
#204462=CARTESIAN_POINT('Ctrl Pts',(-54.275819493118,-78.8993382745417,
60.2790031422139));
#204463=CARTESIAN_POINT('Ctrl Pts',(-54.2950191884045,-79.5191976094664,
60.0083099722502));
#204464=CARTESIAN_POINT('Ctrl Pts',(-54.3333466588036,-80.803899112053,
59.5924195242559));
#204465=CARTESIAN_POINT('Ctrl Pts',(-54.3520059209203,-81.4656598308053,
59.4483995778347));
#204466=CARTESIAN_POINT('Ctrl Pts',(-54.3898335992285,-82.8072553351873,
59.292751143846));
#204467=CARTESIAN_POINT('Ctrl Pts',(-54.4090163993889,-83.4837877804349,
59.281383272417));
#204468=CARTESIAN_POINT('Ctrl Pts',(-54.4639581430243,-85.4117236740045,
59.4396240734754));
#204469=CARTESIAN_POINT('Ctrl Pts',(-54.4983910906639,-86.6372735668571,
59.7731223727129));
#204470=CARTESIAN_POINT('Ctrl Pts',(-54.5726681292479,-88.98890674642,60.9075822236667));
#204471=CARTESIAN_POINT('Ctrl Pts',(-54.6095885006169,-90.0781160339654,
61.7298248074316));
#204472=CARTESIAN_POINT('Ctrl Pts',(-54.6864723593932,-91.8744273761514,
63.749145864274));
#204473=CARTESIAN_POINT('Ctrl Pts',(-54.7233852421897,-92.5640450374486,
64.9263287131589));
#204474=CARTESIAN_POINT('Ctrl Pts',(-54.7712204353895,-93.113501112805,
66.5157418434284));
#204475=CARTESIAN_POINT('Ctrl Pts',(-54.7806358196329,-93.2063305295844,
66.8332160469199));
#204476=CARTESIAN_POINT('Ctrl Pts',(-54.8032919823625,-93.3944761228066,
67.6152358256552));
#204477=CARTESIAN_POINT('Ctrl Pts',(-54.8164128915059,-93.4732278824495,
68.0829828651234));
#204478=CARTESIAN_POINT('Ctrl Pts',(-54.8568831913935,-93.6141114685972,
69.5234256761779));
#204479=CARTESIAN_POINT('Ctrl Pts',(-54.8847845352893,-93.5703528386626,
70.5009228320982));
#204480=CARTESIAN_POINT('Ctrl Pts',(-54.9256171947155,-93.299580095652,
71.9322540715961));
#204481=CARTESIAN_POINT('Ctrl Pts',(-54.9390015578452,-93.1763120124036,
72.4000628234908));
#204482=CARTESIAN_POINT('Ctrl Pts',(-54.9664446175706,-92.8606052411454,
73.326831632913));
#204483=CARTESIAN_POINT('Ctrl Pts',(-54.9804793163858,-92.6668492605553,
73.7840084525099));
#204484=CARTESIAN_POINT('Ctrl Pts',(-54.9945874883696,-92.4407690432347,
74.2253573558264));
#204485=CARTESIAN_POINT('Ctrl Pts',(-55.2458788381492,-73.8447192625517,
73.4662010433421));
#204486=CARTESIAN_POINT('Ctrl Pts',(-55.2297528696875,-74.0655340732995,
74.0006591869956));
#204487=CARTESIAN_POINT('Ctrl Pts',(-55.2135935927371,-74.3311972775467,
74.5155097397992));
#204488=CARTESIAN_POINT('Ctrl Pts',(-55.183301353506,-74.8996943264174,
75.4203468553558));
#204489=CARTESIAN_POINT('Ctrl Pts',(-55.1692882837076,-75.1899507473671,
75.81621473778));
#204490=CARTESIAN_POINT('Ctrl Pts',(-55.1461364105071,-75.7217303075469,
76.4419764121167));
#204491=CARTESIAN_POINT('Ctrl Pts',(-55.1369251615355,-75.9481322718447,
76.6836385079598));
#204492=CARTESIAN_POINT('Ctrl Pts',(-55.090006389838,-77.1564578517171,
77.8542969941396));
#204493=CARTESIAN_POINT('Ctrl Pts',(-55.0515322837808,-78.3035517458425,
78.5934851025729));
#204494=CARTESIAN_POINT('Ctrl Pts',(-54.9792274053784,-80.7159449267234,
79.54388110746));
#204495=CARTESIAN_POINT('Ctrl Pts',(-54.9438092074083,-81.9440597031267,
79.7853203004272));
#204496=CARTESIAN_POINT('Ctrl Pts',(-54.89027037167,-83.8602625554975,79.8101225522134));
#204497=CARTESIAN_POINT('Ctrl Pts',(-54.8715308620345,-84.534374830482,
79.7521743592111));
#204498=CARTESIAN_POINT('Ctrl Pts',(-54.835980245164,-85.7685029902784,
79.5219286684053));
#204499=CARTESIAN_POINT('Ctrl Pts',(-54.8193640330692,-86.3290526933151,
79.367190176599));
#204500=CARTESIAN_POINT('Ctrl Pts',(-54.7840781959813,-87.5074927108403,
78.9313593608611));
#204501=CARTESIAN_POINT('Ctrl Pts',(-54.7654199970558,-88.116753108433,
78.6347357161773));
#204502=CARTESIAN_POINT('Ctrl Pts',(-54.7254516240248,-89.3235904518117,
77.8916193892214));
#204503=CARTESIAN_POINT('Ctrl Pts',(-54.7041942197188,-89.9107924539841,
77.4356074635136));
#204504=CARTESIAN_POINT('Ctrl Pts',(-54.6696585841749,-90.7969186263016,
76.5786314889983));
#204505=CARTESIAN_POINT('Ctrl Pts',(-54.6560407988341,-91.1251485086316,
76.2120331897269));
#204506=CARTESIAN_POINT('Ctrl Pts',(-54.624771622307,-91.8070700324784,
75.3303838982876));
#204507=CARTESIAN_POINT('Ctrl Pts',(-54.6070471573018,-92.1425801188347,
74.8037196308037));
#204508=CARTESIAN_POINT('Ctrl Pts',(-54.5714386598732,-92.717120542965,
73.6895063011282));
#204509=CARTESIAN_POINT('Ctrl Pts',(-54.5539604063772,-92.9537503793338,
73.1036848450657));
#204510=CARTESIAN_POINT('Ctrl Pts',(-54.5180538921639,-93.3231649468449,
71.8733423618886));
#204511=CARTESIAN_POINT('Ctrl Pts',(-54.4995542665266,-93.4508684858144,
71.2302749514709));
#204512=CARTESIAN_POINT('Ctrl Pts',(-54.4495299901436,-93.6271087478463,
69.4805027022376));
#204513=CARTESIAN_POINT('Ctrl Pts',(-54.4193034082145,-93.5594452055571,
68.370856821029));
#204514=CARTESIAN_POINT('Ctrl Pts',(-54.3720253945435,-93.1916543097974,
66.7428817075923));
#204515=CARTESIAN_POINT('Ctrl Pts',(-54.3558699902278,-93.0219857585303,
66.2034796354675));
#204516=CARTESIAN_POINT('Ctrl Pts',(-54.3255956470203,-92.6149618668774,
65.2056719483687));
#204517=CARTESIAN_POINT('Ctrl Pts',(-54.3113954907581,-92.3857452384584,
64.7457714800481));
#204518=CARTESIAN_POINT('Ctrl Pts',(-54.2704420897157,-91.6377007500768,
63.4905370973475));
#204519=CARTESIAN_POINT('Ctrl Pts',(-54.2432415288258,-91.0416890949028,
62.7473696885035));
#204520=CARTESIAN_POINT('Ctrl Pts',(-54.1978552987443,-89.8614061132386,
61.6338059550811));
#204521=CARTESIAN_POINT('Ctrl Pts',(-54.1791614739977,-89.3262307344683,
61.220439620894));
#204522=CARTESIAN_POINT('Ctrl Pts',(-54.15073098846,-88.4740913422993,60.6873304216285));
#204523=CARTESIAN_POINT('Ctrl Pts',(-54.1413258110868,-88.1855274474128,
60.5256647389317));
#204524=CARTESIAN_POINT('Ctrl Pts',(-54.1063868463423,-87.0860231827504,
59.9777549500284));
#204525=CARTESIAN_POINT('Ctrl Pts',(-54.0816698923603,-86.2332398533938,
59.684610714934));
#204526=CARTESIAN_POINT('Ctrl Pts',(-54.0333045512917,-84.5483186723791,
59.3432627791053));
#204527=CARTESIAN_POINT('Ctrl Pts',(-54.0097425891856,-83.7267279618335,
59.2775227600617));
#204528=CARTESIAN_POINT('Ctrl Pts',(-53.9731695174769,-82.4213334318633,
59.3300217190208));
#204529=CARTESIAN_POINT('Ctrl Pts',(-53.9597184654046,-81.9385320176203,
59.3839162936977));
#204530=CARTESIAN_POINT('Ctrl Pts',(-53.9265872639273,-80.7775262929086,
59.5977546904946));
#204531=CARTESIAN_POINT('Ctrl Pts',(-53.906747086961,-80.1082752639565,
59.7929671092526));
#204532=CARTESIAN_POINT('Ctrl Pts',(-53.8775898556133,-79.1541777096603,
60.1801230406874));
#204533=CARTESIAN_POINT('Ctrl Pts',(-53.8682463598381,-78.8507238093768,
60.320911537634));
#204534=CARTESIAN_POINT('Ctrl Pts',(-53.8411009154114,-77.9889598507366,
60.773190208319));
#204535=CARTESIAN_POINT('Ctrl Pts',(-53.8232780385363,-77.4522311778858,
61.1223459295986));
#204536=CARTESIAN_POINT('Ctrl Pts',(-53.7910712531785,-76.5622674900813,
61.8276764044678));
#204537=CARTESIAN_POINT('Ctrl Pts',(-53.7768719459693,-76.1959593877359,
62.1640513327241));
#204538=CARTESIAN_POINT('Ctrl Pts',(-53.7438427134036,-75.3914487368743,
63.0184756185197));
#204539=CARTESIAN_POINT('Ctrl Pts',(-53.7251832600842,-74.9773718025744,
63.5560568101502));
#204540=CARTESIAN_POINT('Ctrl Pts',(-53.6910623784577,-74.3366115978245,
64.5841032757758));
#204541=CARTESIAN_POINT('Ctrl Pts',(-53.6758314458016,-74.0898149296533,
65.0590998480982));
#204542=CARTESIAN_POINT('Ctrl Pts',(-53.6338431539426,-73.5124670231051,
66.4208153637462));
#204543=CARTESIAN_POINT('Ctrl Pts',(-53.6079792363515,-73.2657260226396,
67.3372712664529));
#204544=CARTESIAN_POINT('Ctrl Pts',(-53.5631322461169,-73.068023389348,
68.9108519644783));
#204545=CARTESIAN_POINT('Ctrl Pts',(-53.5447588669558,-73.0479750547569,
69.553312848836));
#204546=CARTESIAN_POINT('Ctrl Pts',(-53.5126853145242,-73.1194954370545,
70.69441226386));
#204547=CARTESIAN_POINT('Ctrl Pts',(-53.4987850519446,-73.1876555209855,
71.1924183709513));
#204548=CARTESIAN_POINT('Ctrl Pts',(-53.4672275747629,-73.4216606742602,
72.2932815615116));
#204549=CARTESIAN_POINT('Ctrl Pts',(-53.4495081762787,-73.6066644662848,
72.8900153957329));
#204550=CARTESIAN_POINT('Ctrl Pts',(-53.4317936414903,-73.844719260035,
73.4662010372508));
#204551=CARTESIAN_POINT('Origin',(-45.8894114130409,-83.3180213346267,69.5522455184007));
#204552=CARTESIAN_POINT('',(-57.4656305641639,-73.8447192505465,73.4662010142849));
#204553=CARTESIAN_POINT('',(-57.0597576325586,-73.8447192590796,73.4662010349383));
#204554=CARTESIAN_POINT('',(-45.8894114130409,-73.8447192590796,73.4662010349383));
#204555=CARTESIAN_POINT('Ctrl Pts',(-55.6519493945588,-73.8447192590796,
73.4662010349383));
#204556=CARTESIAN_POINT('Ctrl Pts',(-55.6596548633805,-73.7410272723995,
73.2152259003247));
#204557=CARTESIAN_POINT('Ctrl Pts',(-55.6673089420921,-73.6472380756339,
72.9599589662023));
#204558=CARTESIAN_POINT('Ctrl Pts',(-55.693783075687,-73.3563706209773,
72.0588877901198));
#204559=CARTESIAN_POINT('Ctrl Pts',(-55.7124900378615,-73.2130079057446,
71.3979008056047));
#204560=CARTESIAN_POINT('Ctrl Pts',(-55.7490543465984,-73.0648169282569,
70.1141264021171));
#204561=CARTESIAN_POINT('Ctrl Pts',(-55.7667415433354,-73.0495893992716,
69.4954674524715));
#204562=CARTESIAN_POINT('Ctrl Pts',(-55.7982479286604,-73.1233063252767,
68.3752183108468));
#204563=CARTESIAN_POINT('Ctrl Pts',(-55.8122316879438,-73.1936777975706,
67.8743663203349));
#204564=CARTESIAN_POINT('Ctrl Pts',(-55.8465381892149,-73.4529159797878,
66.6784751248108));
#204565=CARTESIAN_POINT('Ctrl Pts',(-55.8670281966967,-73.6785787543878,
65.9941580673973));
#204566=CARTESIAN_POINT('Ctrl Pts',(-55.8968590589922,-74.1114591169312,
65.034098859896));
#204567=CARTESIAN_POINT('Ctrl Pts',(-55.9062138364164,-74.2638300519005,
64.7360168915535));
#204568=CARTESIAN_POINT('Ctrl Pts',(-55.9336509373363,-74.7538575094382,
63.8831286030609));
#204569=CARTESIAN_POINT('Ctrl Pts',(-55.951753234742,-75.1299332157745,
63.3523266230311));
#204570=CARTESIAN_POINT('Ctrl Pts',(-55.9884629980572,-75.9748276848023,
62.3719812270974));
#204571=CARTESIAN_POINT('Ctrl Pts',(-56.0068615798354,-76.4411920836949,
61.9241444889541));
#204572=CARTESIAN_POINT('Ctrl Pts',(-56.0437401783078,-77.4752970866365,
61.1035355941262));
#204573=CARTESIAN_POINT('Ctrl Pts',(-56.0624840712685,-78.0441979459242,
60.7372066610557));
#204574=CARTESIAN_POINT('Ctrl Pts',(-56.0979096502699,-79.1575194967214,
60.1669181507204));
#204575=CARTESIAN_POINT('Ctrl Pts',(-56.1143937075693,-79.691291249844,
59.948028732579));
#204576=CARTESIAN_POINT('Ctrl Pts',(-56.1495554039872,-80.8854448912311,
59.5721617095557));
#204577=CARTESIAN_POINT('Ctrl Pts',(-56.1682134633932,-81.5487757186324,
59.4334867485));
#204578=CARTESIAN_POINT('Ctrl Pts',(-56.2016707642748,-82.7284245294484,
59.3064939682056));
#204579=CARTESIAN_POINT('Ctrl Pts',(-56.2162221770782,-83.2393039312188,
59.2898458278949));
#204580=CARTESIAN_POINT('Ctrl Pts',(-56.2572368274195,-84.6830704364769,
59.3506456915793));
#204581=CARTESIAN_POINT('Ctrl Pts',(-56.2828304154574,-85.6070970828485,
59.517499285441));
#204582=CARTESIAN_POINT('Ctrl Pts',(-56.3275371032007,-87.1103919978489,
60.0076922478935));
#204583=CARTESIAN_POINT('Ctrl Pts',(-56.3460612710478,-87.7047786737991,
60.2658608219851));
#204584=CARTESIAN_POINT('Ctrl Pts',(-56.378260555719,-88.7097868041539,
60.8205394610542));
#204585=CARTESIAN_POINT('Ctrl Pts',(-56.3921434363624,-89.1303370186752,
61.094656321998));
#204586=CARTESIAN_POINT('Ctrl Pts',(-56.4154357382099,-89.7911270975001,
61.5980097340351));
#204587=CARTESIAN_POINT('Ctrl Pts',(-56.4247243732342,-90.0433431070999,
61.8100875413661));
#204588=CARTESIAN_POINT('Ctrl Pts',(-56.452214235767,-90.754116528576,62.4687302659228));
#204589=CARTESIAN_POINT('Ctrl Pts',(-56.4704556899168,-91.1815977372855,
62.9464992597366));
#204590=CARTESIAN_POINT('Ctrl Pts',(-56.5071829360745,-91.9628756085017,
64.0038582558589));
#204591=CARTESIAN_POINT('Ctrl Pts',(-56.525925414791,-92.3093942268284,
64.5850212040973));
#204592=CARTESIAN_POINT('Ctrl Pts',(-56.5613911435208,-92.8416373612569,
65.7186337167351));
#204593=CARTESIAN_POINT('Ctrl Pts',(-56.5779176350843,-93.0424188895371,
66.2610542810256));
#204594=CARTESIAN_POINT('Ctrl Pts',(-56.6084856298555,-93.332806991791,
67.3099887600299));
#204595=CARTESIAN_POINT('Ctrl Pts',(-56.6226291267961,-93.4321298310447,
67.811998230913));
#204596=CARTESIAN_POINT('Ctrl Pts',(-56.6548144418948,-93.5702521925257,
68.9519470315959));
#204597=CARTESIAN_POINT('Ctrl Pts',(-56.6729236665936,-93.5877404272269,
69.5903449546178));
#204598=CARTESIAN_POINT('Ctrl Pts',(-56.7089675415116,-93.5043286909993,
70.8561658371274));
#204599=CARTESIAN_POINT('Ctrl Pts',(-56.7264852422334,-93.4047065420545,
71.4809369788909));
#204600=CARTESIAN_POINT('Ctrl Pts',(-56.762454721504,-93.0856878741423,
72.7279953005713));
#204601=CARTESIAN_POINT('Ctrl Pts',(-56.78099231533,-92.8625183377958,73.3463538705992));
#204602=CARTESIAN_POINT('Ctrl Pts',(-56.8380957305256,-92.0033788889631,
75.1605993844289));
#204603=CARTESIAN_POINT('Ctrl Pts',(-56.8750159211701,-91.1890365629882,
76.2556911510731));
#204604=CARTESIAN_POINT('Ctrl Pts',(-56.9394218654422,-89.5083996664527,
77.7726051826705));
#204605=CARTESIAN_POINT('Ctrl Pts',(-56.9646156137638,-88.7524208614728,
78.2908043918305));
#204606=CARTESIAN_POINT('Ctrl Pts',(-57.0145463896372,-87.1660224735993,
79.0917971309653));
#204607=CARTESIAN_POINT('Ctrl Pts',(-57.0393569399326,-86.3479398257574,
79.3822892230226));
#204608=CARTESIAN_POINT('Ctrl Pts',(-57.0824456155048,-84.8436188663561,
79.7105293118066));
#204609=CARTESIAN_POINT('Ctrl Pts',(-57.1011387504411,-84.1714940580514,
79.7889326366568));
#204610=CARTESIAN_POINT('Ctrl Pts',(-57.1385945747034,-82.8468398370674,
79.8120090611029));
#204611=CARTESIAN_POINT('Ctrl Pts',(-57.1572119729289,-82.1975152551376,
79.7615175035752));
#204612=CARTESIAN_POINT('Ctrl Pts',(-57.1894891839894,-81.0638680605308,
79.5638499525962));
#204613=CARTESIAN_POINT('Ctrl Pts',(-57.2033614830846,-80.5773546512452,
79.4417439633923));
#204614=CARTESIAN_POINT('Ctrl Pts',(-57.237438190015,-79.4234850655456,
79.0604173874403));
#204615=CARTESIAN_POINT('Ctrl Pts',(-57.2578090455034,-78.7705347652535,
78.7659901996338));
#204616=CARTESIAN_POINT('Ctrl Pts',(-57.294600414176,-77.6485276573791,
78.1115176796365));
#204617=CARTESIAN_POINT('Ctrl Pts',(-57.3107631445904,-77.1696568020812,
77.7742837679813));
#204618=CARTESIAN_POINT('Ctrl Pts',(-57.3555562978816,-75.9440543266112,
76.7439374202992));
#204619=CARTESIAN_POINT('Ctrl Pts',(-57.3847050625789,-75.2675824966305,
75.9776838207498));
#204620=CARTESIAN_POINT('Ctrl Pts',(-57.4306208441241,-74.3748318537071,
74.5993556208464));
#204621=CARTESIAN_POINT('Ctrl Pts',(-57.4479646014832,-74.0835506812208,
74.0442664246711));
#204622=CARTESIAN_POINT('Ctrl Pts',(-57.4656305635332,-73.8447192505397,
73.4662010142684));
#204623=CARTESIAN_POINT('',(-56.402691677048,-92.4407740768623,74.2253475292745));
#204624=CARTESIAN_POINT('Ctrl Pts',(-56.402691677048,-92.4407740768623,
74.2253475292745));
#204625=CARTESIAN_POINT('Ctrl Pts',(-56.3905033769764,-92.6400598197725,
73.8363051857964));
#204626=CARTESIAN_POINT('Ctrl Pts',(-56.3782950668991,-92.8142542880859,
73.434915401122));
#204627=CARTESIAN_POINT('Ctrl Pts',(-56.3538404997768,-93.1075649334602,
72.6200352877034));
#204628=CARTESIAN_POINT('Ctrl Pts',(-56.3416239456816,-93.2273594088019,
72.2077141799071));
#204629=CARTESIAN_POINT('Ctrl Pts',(-56.3064251645048,-93.4976065211303,
70.9992048619457));
#204630=CARTESIAN_POINT('Ctrl Pts',(-56.2841306774455,-93.5800601632956,
70.1911577827392));
#204631=CARTESIAN_POINT('Ctrl Pts',(-56.2462056610967,-93.5576184697801,
68.8413324644591));
#204632=CARTESIAN_POINT('Ctrl Pts',(-56.2308430996121,-93.5058840444699,
68.3023686440525));
#204633=CARTESIAN_POINT('Ctrl Pts',(-56.1861214976241,-93.2323654622646,
66.7532673876798));
#204634=CARTESIAN_POINT('Ctrl Pts',(-56.1578623953141,-92.9002472360519,
65.7694620125991));
#204635=CARTESIAN_POINT('Ctrl Pts',(-56.1193148260535,-92.2756548246651,
64.5590576078324));
#204636=CARTESIAN_POINT('Ctrl Pts',(-56.1099340714407,-92.1104824250455,
64.2736330038756));
#204637=CARTESIAN_POINT('Ctrl Pts',(-56.0706362546844,-91.3614570484951,
63.1122829809782));
#204638=CARTESIAN_POINT('Ctrl Pts',(-56.0418346173385,-90.6582563846677,
62.3209985596782));
#204639=CARTESIAN_POINT('Ctrl Pts',(-55.9952001354449,-89.3883262034003,
61.2716708088244));
#204640=CARTESIAN_POINT('Ctrl Pts',(-55.9781648862883,-88.8975221472293,
60.9333305046939));
#204641=CARTESIAN_POINT('Ctrl Pts',(-55.9471894467687,-87.9381682201456,
60.3884524901742));
#204642=CARTESIAN_POINT('Ctrl Pts',(-55.9331194762118,-87.4781282173937,
60.1706478673319));
#204643=CARTESIAN_POINT('Ctrl Pts',(-55.9010251811469,-86.4097959957748,
59.7589459962414));
#204644=CARTESIAN_POINT('Ctrl Pts',(-55.8829313028535,-85.7957245889421,
59.5858640933454));
#204645=CARTESIAN_POINT('Ctrl Pts',(-55.8469130984081,-84.5488417933286,
59.3568591162553));
#204646=CARTESIAN_POINT('Ctrl Pts',(-55.829404124793,-83.9188942874507,
59.3004272451562));
#204647=CARTESIAN_POINT('Ctrl Pts',(-55.7934480639542,-82.6322366741683,
59.3042251232283));
#204648=CARTESIAN_POINT('Ctrl Pts',(-55.7749181977989,-81.9784073585776,
59.3690416053286));
#204649=CARTESIAN_POINT('Ctrl Pts',(-55.7178274654666,-80.0093521796394,
59.7572670969582));
#204650=CARTESIAN_POINT('Ctrl Pts',(-55.6809086679753,-78.7481366318407,
60.2783551802272));
#204651=CARTESIAN_POINT('Ctrl Pts',(-55.6097089193793,-76.6669921704943,
61.6685973025684));
#204652=CARTESIAN_POINT('Ctrl Pts',(-55.5781944556113,-75.8241727682959,
62.464908313525));
#204653=CARTESIAN_POINT('Ctrl Pts',(-55.5315078954419,-74.832900228938,
63.7806558257333));
#204654=CARTESIAN_POINT('Ctrl Pts',(-55.5173291291132,-74.5635846023956,
64.1979608868738));
#204655=CARTESIAN_POINT('Ctrl Pts',(-55.4940067945626,-74.16665515639,64.9235733410436));
#204656=CARTESIAN_POINT('Ctrl Pts',(-55.4847913851266,-74.0219336784218,
65.2215567936392));
#204657=CARTESIAN_POINT('Ctrl Pts',(-55.4378676907604,-73.3610031428395,
66.7689170716168));
#204658=CARTESIAN_POINT('Ctrl Pts',(-55.399391064315,-73.0811505043503,
68.1046266887717));
#204659=CARTESIAN_POINT('Ctrl Pts',(-55.3240281637205,-73.0557992009588,
70.8070225842464));
#204660=CARTESIAN_POINT('Ctrl Pts',(-55.2855668439352,-73.3103358396947,
72.1472223742944));
#204661=CARTESIAN_POINT('Ctrl Pts',(-55.2472197563395,-73.826436129375,
73.4217271981451));
#204662=CARTESIAN_POINT('Ctrl Pts',(-55.2465492717017,-73.8355389359018,
73.4439810648777));
#204663=CARTESIAN_POINT('Ctrl Pts',(-55.2458788381492,-73.8447192625517,
73.4662010433421));
#204664=CARTESIAN_POINT('Ctrl Pts',(-57.0597576325586,-73.8447192590796,
73.4662010349383));
#204665=CARTESIAN_POINT('Ctrl Pts',(-57.0383631309816,-74.1368641142954,
74.173305766094));
#204666=CARTESIAN_POINT('Ctrl Pts',(-57.017120994494,-74.5075970143452,
74.8462899755402));
#204667=CARTESIAN_POINT('Ctrl Pts',(-56.9775517730568,-75.3131405065833,
75.9848714513742));
#204668=CARTESIAN_POINT('Ctrl Pts',(-56.9596411120092,-75.7221508602249,
76.4630748477586));
#204669=CARTESIAN_POINT('Ctrl Pts',(-56.9262735382076,-76.5782428806903,
77.2955277986793));
#204670=CARTESIAN_POINT('Ctrl Pts',(-56.9105628863771,-77.0161437030378,
77.6559096055087));
#204671=CARTESIAN_POINT('Ctrl Pts',(-56.8692274112796,-78.2210699328814,
78.49052611963));
#204672=CARTESIAN_POINT('Ctrl Pts',(-56.8435370700548,-79.0248178896983,
78.9031918397772));
#204673=CARTESIAN_POINT('Ctrl Pts',(-56.8002362825214,-80.4868816128833,
79.4251031806845));
#204674=CARTESIAN_POINT('Ctrl Pts',(-56.782023377819,-81.1212594724405,
79.5853357798321));
#204675=CARTESIAN_POINT('Ctrl Pts',(-56.7456291264912,-82.3892565663906,
79.7795008913734));
#204676=CARTESIAN_POINT('Ctrl Pts',(-56.7276633061683,-83.0194376518196,
79.8172453346938));
#204677=CARTESIAN_POINT('Ctrl Pts',(-56.6910944083757,-84.3275691096218,
79.7749717110202));
#204678=CARTESIAN_POINT('Ctrl Pts',(-56.6722514824881,-85.0021935016001,
79.6856989908197));
#204679=CARTESIAN_POINT('Ctrl Pts',(-56.6380194886854,-86.1789920181178,
79.4091352178211));
#204680=CARTESIAN_POINT('Ctrl Pts',(-56.6228592144546,-86.6847766798411,
79.2480375883778));
#204681=CARTESIAN_POINT('Ctrl Pts',(-56.5944086671809,-87.6200748728344,
78.8680794275189));
#204682=CARTESIAN_POINT('Ctrl Pts',(-56.5811308970273,-88.0511129218097,
78.6566551578047));
#204683=CARTESIAN_POINT('Ctrl Pts',(-56.5404818101695,-89.3082340958285,
77.9265516464997));
#204684=CARTESIAN_POINT('Ctrl Pts',(-56.5125613702138,-90.0766500260617,
77.3196503160365));
#204685=CARTESIAN_POINT('Ctrl Pts',(-56.4717017702708,-91.0808193787086,
76.2630686063062));
#204686=CARTESIAN_POINT('Ctrl Pts',(-56.4583111596744,-91.3886321735106,
75.8895496120529));
#204687=CARTESIAN_POINT('Ctrl Pts',(-56.4308548308858,-91.9566231006264,
75.0914887461845));
#204688=CARTESIAN_POINT('Ctrl Pts',(-56.4168131368927,-92.2145804213453,
74.6669190743884));
#204689=CARTESIAN_POINT('Ctrl Pts',(-56.4026978510105,-92.4407741543022,
74.2253473780977));
#204690=CARTESIAN_POINT('Origin',(-45.8894114130409,-83.3180213346267,69.5522455184007));
#204691=CARTESIAN_POINT('',(-59.2798347108578,-73.8447192567251,73.4662010292395));
#204692=CARTESIAN_POINT('',(-58.8740778711611,-73.8447192590796,73.4662010349383));
#204693=CARTESIAN_POINT('',(-45.8894114130409,-73.8447192590796,73.4662010349383));
#204694=CARTESIAN_POINT('Ctrl Pts',(-57.4656305635332,-73.8447192505397,
73.4662010142684));
#204695=CARTESIAN_POINT('Ctrl Pts',(-57.467015475443,-73.8259962117467,
73.4208839424198));
#204696=CARTESIAN_POINT('Ctrl Pts',(-57.4684018447326,-73.8075955063203,
73.3754256525906));
#204697=CARTESIAN_POINT('Ctrl Pts',(-57.4791268020266,-73.6678971821377,
73.0230533866649));
#204698=CARTESIAN_POINT('Ctrl Pts',(-57.4885180167998,-73.5611619934532,
72.7105833747677));
#204699=CARTESIAN_POINT('Ctrl Pts',(-57.523407156596,-73.2210881588465,
71.531826866936));
#204700=CARTESIAN_POINT('Ctrl Pts',(-57.548081453985,-73.0866520074193,
70.6412316611888));
#204701=CARTESIAN_POINT('Ctrl Pts',(-57.5888899414059,-73.0594451953212,
69.1913900793089));
#204702=CARTESIAN_POINT('Ctrl Pts',(-57.6046512373244,-73.0938694204248,
68.6382921288233));
#204703=CARTESIAN_POINT('Ctrl Pts',(-57.6381300257707,-73.2620038171208,
67.4712027258487));
#204704=CARTESIAN_POINT('Ctrl Pts',(-57.6554659852384,-73.4078004036538,
66.8611954226435));
#204705=CARTESIAN_POINT('Ctrl Pts',(-57.6912072348374,-73.8173648043539,
65.6502278125564));
#204706=CARTESIAN_POINT('Ctrl Pts',(-57.7096703600775,-74.0849436597277,
65.0535258942587));
#204707=CARTESIAN_POINT('Ctrl Pts',(-57.7592658896886,-74.9467254860372,
63.5377100424494));
#204708=CARTESIAN_POINT('Ctrl Pts',(-57.7891281575565,-75.6340776115638,
62.6812739247584));
#204709=CARTESIAN_POINT('Ctrl Pts',(-57.8362286935468,-76.8675816802812,
61.5659286950294));
#204710=CARTESIAN_POINT('Ctrl Pts',(-57.8525941770391,-77.3230367740463,
61.2186032227383));
#204711=CARTESIAN_POINT('Ctrl Pts',(-57.8830343508329,-78.2366472048036,
60.635732430482));
#204712=CARTESIAN_POINT('Ctrl Pts',(-57.8972020710319,-78.6882446648011,
60.3931112276017));
#204713=CARTESIAN_POINT('Ctrl Pts',(-57.9294173301977,-79.7386233211922,
59.9264068339872));
#204714=CARTESIAN_POINT('Ctrl Pts',(-57.9475315653165,-80.3440470263072,
59.7224783147016));
#204715=CARTESIAN_POINT('Ctrl Pts',(-57.9835838838406,-81.5789840879344,
59.431134072273));
#204716=CARTESIAN_POINT('Ctrl Pts',(-58.0011045048751,-82.2055797286569,
59.3432482787389));
#204717=CARTESIAN_POINT('Ctrl Pts',(-58.0370784200417,-83.491556625581,
59.2827403410888));
#204718=CARTESIAN_POINT('Ctrl Pts',(-58.0556185294284,-84.1482869379266,
59.3148877030279));
#204719=CARTESIAN_POINT('Ctrl Pts',(-58.1127259893701,-86.1347912884453,
59.6046365093555));
#204720=CARTESIAN_POINT('Ctrl Pts',(-58.1496465648296,-87.4204709874273,
60.0623024090173));
#204721=CARTESIAN_POINT('Ctrl Pts',(-58.2140602109242,-89.3635408703946,
61.2247457987552));
#204722=CARTESIAN_POINT('Ctrl Pts',(-58.2392619101364,-90.0807132733979,
61.7958566462899));
#204723=CARTESIAN_POINT('Ctrl Pts',(-58.289212135638,-91.3118471784145,
63.078474596357));
#204724=CARTESIAN_POINT('Ctrl Pts',(-58.3140360354744,-91.8295124567072,
63.7759588220253));
#204725=CARTESIAN_POINT('Ctrl Pts',(-58.3571375745626,-92.5841413592949,
65.1186017192531));
#204726=CARTESIAN_POINT('Ctrl Pts',(-58.3758307916147,-92.8559443419004,
65.7382969424522));
#204727=CARTESIAN_POINT('Ctrl Pts',(-58.4132835267388,-93.2659095571014,
66.9980073250782));
#204728=CARTESIAN_POINT('Ctrl Pts',(-58.4318976573724,-93.4077773086004,
67.6335361596171));
#204729=CARTESIAN_POINT('Ctrl Pts',(-58.4641721348258,-93.5507993058548,
68.7752647657367));
#204730=CARTESIAN_POINT('Ctrl Pts',(-58.4780448026798,-93.5765425307035,
69.2762201526045));
#204731=CARTESIAN_POINT('Ctrl Pts',(-58.501263199602,-93.5583826674336,
70.1040382693334));
#204732=CARTESIAN_POINT('Ctrl Pts',(-58.5104876105466,-93.5355624150462,
70.4304981763666));
#204733=CARTESIAN_POINT('Ctrl Pts',(-58.5334900665776,-93.4403878401189,
71.2357751792268));
#204734=CARTESIAN_POINT('Ctrl Pts',(-58.547318724833,-93.3496548816368,
71.7116215901034));
#204735=CARTESIAN_POINT('Ctrl Pts',(-58.574536530198,-93.1018985141553,
72.6460147409128));
#204736=CARTESIAN_POINT('Ctrl Pts',(-58.587905219172,-92.9453145061345,
73.1034273015737));
#204737=CARTESIAN_POINT('Ctrl Pts',(-58.6188859134196,-92.5135392729312,
74.1233723398468));
#204738=CARTESIAN_POINT('Ctrl Pts',(-58.6365653879551,-92.217926162049,
74.6751774283831));
#204739=CARTESIAN_POINT('Ctrl Pts',(-58.6927354152328,-91.1305436805013,
76.3234632986986));
#204740=CARTESIAN_POINT('Ctrl Pts',(-58.7296145133979,-90.1718171794844,
77.2924245070318));
#204741=CARTESIAN_POINT('Ctrl Pts',(-58.8064690912481,-87.932682125596,
78.803961807163));
#204742=CARTESIAN_POINT('Ctrl Pts',(-58.8433913931026,-86.6738345838654,
79.3311957990902));
#204743=CARTESIAN_POINT('Ctrl Pts',(-58.8912730138183,-85.0240359243524,
79.6647104567488));
#204744=CARTESIAN_POINT('Ctrl Pts',(-58.9007099114252,-84.6960500960934,
79.714601179362));
#204745=CARTESIAN_POINT('Ctrl Pts',(-58.9246479319649,-83.8492960797604,
79.8016496087255));
#204746=CARTESIAN_POINT('Ctrl Pts',(-58.9390230634141,-83.3290745763266,
79.8154039115205));
#204747=CARTESIAN_POINT('Ctrl Pts',(-58.983088324147,-81.7582657834689,
79.7374628040006));
#204748=CARTESIAN_POINT('Ctrl Pts',(-59.0132451352954,-80.7207744835811,
79.5234944201013));
#204749=CARTESIAN_POINT('Ctrl Pts',(-59.0518229434533,-79.4253578817725,
79.0400433472406));
#204750=CARTESIAN_POINT('Ctrl Pts',(-59.0609975786727,-79.1223001401009,
78.9099727851408));
#204751=CARTESIAN_POINT('Ctrl Pts',(-59.0991745160973,-77.8979093966226,
78.3130146836009));
#204752=CARTESIAN_POINT('Ctrl Pts',(-59.1287536206049,-77.0434672368736,
77.722843357872));
#204753=CARTESIAN_POINT('Ctrl Pts',(-59.1667441086209,-76.0522700704332,
76.7896127227359));
#204754=CARTESIAN_POINT('Ctrl Pts',(-59.175894985545,-75.8238468424815,
76.5528150534514));
#204755=CARTESIAN_POINT('Ctrl Pts',(-59.2147979782694,-74.90895439182,75.5081892250738));
#204756=CARTESIAN_POINT('Ctrl Pts',(-59.2451433370349,-74.3385626997602,
74.6074410487942));
#204757=CARTESIAN_POINT('Ctrl Pts',(-59.276419405404,-73.8919916490818,
73.5791817223545));
#204758=CARTESIAN_POINT('Ctrl Pts',(-59.2781271442497,-73.8681010896515,
73.522794203641));
#204759=CARTESIAN_POINT('Ctrl Pts',(-59.2798347108578,-73.8447192543706,
73.4662010235407));
#204760=CARTESIAN_POINT('Ctrl Pts',(-58.8740778711611,-73.8447192590796,
73.4662010349383));
#204761=CARTESIAN_POINT('Ctrl Pts',(-58.865480677016,-73.9616231644785,
73.7491541765811));
#204762=CARTESIAN_POINT('Ctrl Pts',(-58.8568298332965,-74.09121168495,74.0268880893285));
#204763=CARTESIAN_POINT('Ctrl Pts',(-58.8302237393543,-74.5252897744171,
74.8577555728255));
#204764=CARTESIAN_POINT('Ctrl Pts',(-58.8122496763533,-74.8684541002789,
75.3888023861618));
#204765=CARTESIAN_POINT('Ctrl Pts',(-58.7768679492777,-75.6511414097794,
76.3849489172506));
#204766=CARTESIAN_POINT('Ctrl Pts',(-58.7592049293814,-76.0897008063705,
76.8473303810519));
#204767=CARTESIAN_POINT('Ctrl Pts',(-58.7269131274484,-76.9486812697864,
77.5989544351491));
#204768=CARTESIAN_POINT('Ctrl Pts',(-58.7124707266324,-77.3531964397123,
77.9032261900877));
#204769=CARTESIAN_POINT('Ctrl Pts',(-58.6807977870372,-78.29566564173,78.5085980364354));
#204770=CARTESIAN_POINT('Ctrl Pts',(-58.6638417859424,-78.8416606190714,
78.7935930503238));
#204771=CARTESIAN_POINT('Ctrl Pts',(-58.627698835136,-80.0336530067509,
79.2852146576557));
#204772=CARTESIAN_POINT('Ctrl Pts',(-58.608496923001,-80.6812934670574,
79.4802570519605));
#204773=CARTESIAN_POINT('Ctrl Pts',(-58.5600660160198,-82.3557729216487,
79.8090010738735));
#204774=CARTESIAN_POINT('Ctrl Pts',(-58.5318567286296,-83.3923970656817,
79.8537709129494));
#204775=CARTESIAN_POINT('Ctrl Pts',(-58.4853312865826,-85.0232559252403,
79.6777124242945));
#204776=CARTESIAN_POINT('Ctrl Pts',(-58.4679508268199,-85.6213368974583,
79.558626364145));
#204777=CARTESIAN_POINT('Ctrl Pts',(-58.4380518470019,-86.646968988707,
79.2575264967924));
#204778=CARTESIAN_POINT('Ctrl Pts',(-58.42528094242,-87.0793893314218,79.0982647335386));
#204779=CARTESIAN_POINT('Ctrl Pts',(-58.3934235862151,-88.1159538346857,
78.6350881133373));
#204780=CARTESIAN_POINT('Ctrl Pts',(-58.3741823220147,-88.7035566415454,
78.2994838844307));
#204781=CARTESIAN_POINT('Ctrl Pts',(-58.3313046014104,-89.9366003987063,
77.4235995634658));
#204782=CARTESIAN_POINT('Ctrl Pts',(-58.3083313497893,-90.5573190559137,
76.8567902276832));
#204783=CARTESIAN_POINT('Ctrl Pts',(-58.2592872983452,-91.6885342963543,
75.5363384200497));
#204784=CARTESIAN_POINT('Ctrl Pts',(-58.2335590056109,-92.1820867856877,
74.777493662248));
#204785=CARTESIAN_POINT('Ctrl Pts',(-58.1901753773432,-92.8515860581853,
73.3734487086653));
#204786=CARTESIAN_POINT('Ctrl Pts',(-58.1719163428853,-93.0759736461244,
72.7573677826434));
#204787=CARTESIAN_POINT('Ctrl Pts',(-58.1354603489394,-93.398315423905,
71.5137992126148));
#204788=CARTESIAN_POINT('Ctrl Pts',(-58.1174903912482,-93.4998675695853,
70.8901716192675));
#204789=CARTESIAN_POINT('Ctrl Pts',(-58.0824142987632,-93.5867158206437,
69.6374893199529));
#204790=CARTESIAN_POINT('Ctrl Pts',(-58.0650557091113,-93.5728043262034,
69.0111571492715));
#204791=CARTESIAN_POINT('Ctrl Pts',(-58.033439441235,-93.446014573542,67.9001845679106));
#204792=CARTESIAN_POINT('Ctrl Pts',(-58.0193633296556,-93.3548473656371,
67.4150341783458));
#204793=CARTESIAN_POINT('Ctrl Pts',(-57.984896436781,-93.0444752203358,
66.2382037502742));
#204794=CARTESIAN_POINT('Ctrl Pts',(-57.964979096147,-92.7861597068894,
65.5596103650216));
#204795=CARTESIAN_POINT('Ctrl Pts',(-57.9256306149137,-92.1527470234762,
64.3113813617936));
#204796=CARTESIAN_POINT('Ctrl Pts',(-57.906324565792,-91.7881652191835,
63.7405605140367));
#204797=CARTESIAN_POINT('Ctrl Pts',(-57.8696146466932,-90.9849265731252,
62.7208107423569));
#204798=CARTESIAN_POINT('Ctrl Pts',(-57.8524474480341,-90.5560339049798,
62.2679395581874));
#204799=CARTESIAN_POINT('Ctrl Pts',(-57.816081258715,-89.5821851003058,
61.4111191668209));
#204800=CARTESIAN_POINT('Ctrl Pts',(-57.7968753902134,-89.0328908418219,
61.0165594991972));
#204801=CARTESIAN_POINT('Ctrl Pts',(-57.7495900455221,-87.5903056963919,
60.1824216424184));
#204802=CARTESIAN_POINT('Ctrl Pts',(-57.7224612188126,-86.6642607996665,
59.813216008457));
#204803=CARTESIAN_POINT('Ctrl Pts',(-57.6786930873766,-85.1618430352934,
59.4542952374702));
#204804=CARTESIAN_POINT('Ctrl Pts',(-57.662870210739,-84.6144877193528,
59.3695416427853));
#204805=CARTESIAN_POINT('Ctrl Pts',(-57.6318897240014,-83.5148596654779,
59.2894106959836));
#204806=CARTESIAN_POINT('Ctrl Pts',(-57.616694018074,-82.9644194841229,
59.29361524856));
#204807=CARTESIAN_POINT('Ctrl Pts',(-57.5823326533279,-81.7445440283663,
59.4012675295343));
#204808=CARTESIAN_POINT('Ctrl Pts',(-57.5630922550812,-81.0796192684715,
59.5268914182743));
#204809=CARTESIAN_POINT('Ctrl Pts',(-57.5200807259351,-79.6238649777219,
59.9540763863877));
#204810=CARTESIAN_POINT('Ctrl Pts',(-57.496981824707,-78.8481281168846,
60.2898647187717));
#204811=CARTESIAN_POINT('Ctrl Pts',(-57.4477592580867,-77.3440856523192,
61.1743283643562));
#204812=CARTESIAN_POINT('Ctrl Pts',(-57.42199881721,-76.6297843294988,61.7327245217374));
#204813=CARTESIAN_POINT('Ctrl Pts',(-57.3785501803015,-75.5392890057419,
62.845304764873));
#204814=CARTESIAN_POINT('Ctrl Pts',(-57.3602576970691,-75.1266074514152,
63.3560804893024));
#204815=CARTESIAN_POINT('Ctrl Pts',(-57.3237553788541,-74.4177483227882,
64.4291868520268));
#204816=CARTESIAN_POINT('Ctrl Pts',(-57.3057811167003,-74.1193365693104,
64.9866343142496));
#204817=CARTESIAN_POINT('Ctrl Pts',(-57.2703971876994,-73.6268660256079,
66.153940148766));
#204818=CARTESIAN_POINT('Ctrl Pts',(-57.252732005662,-73.4347273572782,
66.7616419920649));
#204819=CARTESIAN_POINT('Ctrl Pts',(-57.2204301539975,-73.1931212225111,
67.8775242147072));
#204820=CARTESIAN_POINT('Ctrl Pts',(-57.2059797441725,-73.1228285498709,
68.379072569883));
#204821=CARTESIAN_POINT('Ctrl Pts',(-57.1743559469827,-73.0498849447111,
69.4951367228938));
#204822=CARTESIAN_POINT('Ctrl Pts',(-57.1574534724381,-73.0648239198485,
70.1088705785681));
#204823=CARTESIAN_POINT('Ctrl Pts',(-57.1213672411522,-73.2111942817992,
71.3879527785283));
#204824=CARTESIAN_POINT('Ctrl Pts',(-57.1021665281674,-73.3539131345902,
72.0491045978209));
#204825=CARTESIAN_POINT('Ctrl Pts',(-57.07519652206,-73.6449321917794,72.9536791724396));
#204826=CARTESIAN_POINT('Ctrl Pts',(-57.0674445709045,-73.7397530610107,
73.2121418107528));
#204827=CARTESIAN_POINT('Ctrl Pts',(-57.0597576325586,-73.8447192590796,
73.4662010349383));
#204828=CARTESIAN_POINT('Origin',(-45.8894114130409,-83.3180213346267,69.5522455184007));
#204829=CARTESIAN_POINT('',(-61.0939133588288,-73.8447192590796,73.4662010349383));
#204830=CARTESIAN_POINT('',(-60.6878802914039,-73.844719258044,73.4662010324316));
#204831=CARTESIAN_POINT('',(-45.8894114130409,-73.8447192590796,73.4662010349383));
#204832=CARTESIAN_POINT('Ctrl Pts',(-59.2798347108578,-73.8447192543706,
73.4662010235407));
#204833=CARTESIAN_POINT('Ctrl Pts',(-59.2873239377854,-73.7421687186716,
73.2179886455785));
#204834=CARTESIAN_POINT('Ctrl Pts',(-59.2948125599226,-73.6494041099293,
72.9658202025441));
#204835=CARTESIAN_POINT('Ctrl Pts',(-59.3212550248384,-73.3587591160992,
72.0683661032157));
#204836=CARTESIAN_POINT('Ctrl Pts',(-59.3404565657231,-73.2147647592278,
71.4074966013702));
#204837=CARTESIAN_POINT('Ctrl Pts',(-59.388980080526,-73.0170996645956,
69.7092774270818));
#204838=CARTESIAN_POINT('Ctrl Pts',(-59.4172768982382,-73.0538311498301,
68.6690429747557));
#204839=CARTESIAN_POINT('Ctrl Pts',(-59.4640581669113,-73.3595772879527,
67.0484062054337));
#204840=CARTESIAN_POINT('Ctrl Pts',(-59.4815942395945,-73.5274854184184,
66.4562414312941));
#204841=CARTESIAN_POINT('Ctrl Pts',(-59.5124154215553,-73.9220915867976,
65.4270660511812));
#204842=CARTESIAN_POINT('Ctrl Pts',(-59.5259528039954,-74.1290945036622,
64.9845080489647));
#204843=CARTESIAN_POINT('Ctrl Pts',(-59.5586389489397,-74.695886677548,
63.9685682266536));
#204844=CARTESIAN_POINT('Ctrl Pts',(-59.5779246592963,-75.0824350281104,
63.4127210382677));
#204845=CARTESIAN_POINT('Ctrl Pts',(-59.6160754054652,-75.957435833677,
62.3872808123945));
#204846=CARTESIAN_POINT('Ctrl Pts',(-59.6346024281748,-76.4433492235958,
61.9198262813317));
#204847=CARTESIAN_POINT('Ctrl Pts',(-59.6724351127768,-77.5016643579224,
61.0853546234917));
#204848=CARTESIAN_POINT('Ctrl Pts',(-59.6916891412228,-78.0717858971223,
60.7207537097166));
#204849=CARTESIAN_POINT('Ctrl Pts',(-59.7328542612989,-79.3668808076306,
60.062470759711));
#204850=CARTESIAN_POINT('Ctrl Pts',(-59.7542186855682,-80.0980279749228,
59.790125831768));
#204851=CARTESIAN_POINT('Ctrl Pts',(-59.7951715359065,-81.509865753293,
59.4403143194271));
#204852=CARTESIAN_POINT('Ctrl Pts',(-59.8145446366639,-82.1813180901955,
59.3430109094515));
#204853=CARTESIAN_POINT('Ctrl Pts',(-59.8478622292068,-83.361431778364,
59.289929148128));
#204854=CARTESIAN_POINT('Ctrl Pts',(-59.8618209663203,-83.8664114920447,
59.3044997145979));
#204855=CARTESIAN_POINT('Ctrl Pts',(-59.8935251351027,-84.993946172304,
59.4206409789947));
#204856=CARTESIAN_POINT('Ctrl Pts',(-59.9113264747551,-85.6123672195088,
59.5425453224756));
#204857=CARTESIAN_POINT('Ctrl Pts',(-59.96760981281,-87.5103181489269,60.1019131248088));
#204858=CARTESIAN_POINT('Ctrl Pts',(-60.0044818029743,-88.7169214609657,
60.7354431445205));
#204859=CARTESIAN_POINT('Ctrl Pts',(-60.0813271816948,-90.8167160050427,
62.4347436381659));
#204860=CARTESIAN_POINT('Ctrl Pts',(-60.1182483491901,-91.688878557295,
63.4844612452277));
#204861=CARTESIAN_POINT('Ctrl Pts',(-60.1661320368538,-92.4901236914144,
64.9647587136454));
#204862=CARTESIAN_POINT('Ctrl Pts',(-60.1755708910434,-92.6337496116151,
65.263923404593));
#204863=CARTESIAN_POINT('Ctrl Pts',(-60.1996437446451,-92.9664064236839,
66.0527836900448));
#204864=CARTESIAN_POINT('Ctrl Pts',(-60.2141509106924,-93.1328026992833,
66.550972454217));
#204865=CARTESIAN_POINT('Ctrl Pts',(-60.2579231222864,-93.5126233441831,
68.0660113822973));
#204866=CARTESIAN_POINT('Ctrl Pts',(-60.2876399382542,-93.6106698144504,
69.1048112013147));
#204867=CARTESIAN_POINT('Ctrl Pts',(-60.325770193447,-93.5322403454906,
70.4690205320168));
#204868=CARTESIAN_POINT('Ctrl Pts',(-60.3349266672721,-93.497552757433,
70.7963862117687));
#204869=CARTESIAN_POINT('Ctrl Pts',(-60.3736531787992,-93.2859391199713,
72.1622881970776));
#204870=CARTESIAN_POINT('Ctrl Pts',(-60.4038129149676,-92.965247396422,
73.1720168367747));
#204871=CARTESIAN_POINT('Ctrl Pts',(-60.4423937032275,-92.3496860665155,
74.410246256175));
#204872=CARTESIAN_POINT('Ctrl Pts',(-60.4515684601349,-92.1888099356396,
74.6981417606306));
#204873=CARTESIAN_POINT('Ctrl Pts',(-60.4897418311879,-91.4678567838218,
75.8537211450771));
#204874=CARTESIAN_POINT('Ctrl Pts',(-60.5193171545131,-90.7921521948344,
76.6420825551035));
#204875=CARTESIAN_POINT('Ctrl Pts',(-60.5573038070801,-89.7610650936442,
77.5308299351059));
#204876=CARTESIAN_POINT('Ctrl Pts',(-60.5664545311213,-89.5018137519351,
77.7334027205151));
#204877=CARTESIAN_POINT('Ctrl Pts',(-60.6053623929022,-88.3676161923673,
78.5348760006254));
#204878=CARTESIAN_POINT('Ctrl Pts',(-60.6357128673784,-87.4122867627898,
79.0086219988744));
#204879=CARTESIAN_POINT('Ctrl Pts',(-60.6744881182545,-86.0868170529555,
79.4267115110407));
#204880=CARTESIAN_POINT('Ctrl Pts',(-60.683670824061,-85.7676285026662,
79.5106958294285));
#204881=CARTESIAN_POINT('Ctrl Pts',(-60.7118302698351,-84.7849002375619,
79.7191542008022));
#204882=CARTESIAN_POINT('Ctrl Pts',(-60.7310319109037,-84.1126408753728,
79.7936482022817));
#204883=CARTESIAN_POINT('Ctrl Pts',(-60.7795303438115,-82.4039510736968,
79.8136444435586));
#204884=CARTESIAN_POINT('Ctrl Pts',(-60.8078034529711,-81.374039833783,
79.6692000450616));
#204885=CARTESIAN_POINT('Ctrl Pts',(-60.8545148446357,-79.7961876611496,
79.1976901625094));
#204886=CARTESIAN_POINT('Ctrl Pts',(-60.8720082387315,-79.2260327763903,
78.9699713583507));
#204887=CARTESIAN_POINT('Ctrl Pts',(-60.9025694825878,-78.2514870702418,
78.475431412836));
#204888=CARTESIAN_POINT('Ctrl Pts',(-60.9158896374163,-77.8391334233009,
78.2283508503706));
#204889=CARTESIAN_POINT('Ctrl Pts',(-60.9483391397852,-76.8921846906305,
77.566424912575));
#204890=CARTESIAN_POINT('Ctrl Pts',(-60.9676110033283,-76.3783307299097,
77.1258263425336));
#204891=CARTESIAN_POINT('Ctrl Pts',(-61.0069268347375,-75.4185044007876,
76.1225455087659));
#204892=CARTESIAN_POINT('Ctrl Pts',(-61.0265516412905,-74.9805923799831,
75.5571176972676));
#204893=CARTESIAN_POINT('Ctrl Pts',(-61.0622515558693,-74.3115140978787,
74.4772523777343));
#204894=CARTESIAN_POINT('Ctrl Pts',(-61.07809329045,-74.0572958058767,73.9807193613414));
#204895=CARTESIAN_POINT('Ctrl Pts',(-61.0939133588288,-73.8447192590796,
73.4662010349383));
#204896=CARTESIAN_POINT('Ctrl Pts',(-60.6878802914039,-73.8447192570083,
73.466201029925));
#204897=CARTESIAN_POINT('Ctrl Pts',(-60.6549485354339,-74.2867494945032,
74.5360869688175));
#204898=CARTESIAN_POINT('Ctrl Pts',(-60.6232629605615,-74.9068773164,75.5234704922587));
#204899=CARTESIAN_POINT('Ctrl Pts',(-60.5753209802943,-76.0346255959043,
76.7840831150594));
#204900=CARTESIAN_POINT('Ctrl Pts',(-60.5600539343161,-76.4209829040694,
77.1534423460483));
#204901=CARTESIAN_POINT('Ctrl Pts',(-60.5260316686445,-77.3582558311916,
77.9189217224717));
#204902=CARTESIAN_POINT('Ctrl Pts',(-60.507373814461,-77.9232451295373,
78.293897249308));
#204903=CARTESIAN_POINT('Ctrl Pts',(-60.4735852233983,-78.9827499354831,
78.8549804346847));
#204904=CARTESIAN_POINT('Ctrl Pts',(-60.4586939764479,-79.4624729874221,
79.063827717357));
#204905=CARTESIAN_POINT('Ctrl Pts',(-60.426245377712,-80.5423576065695,
79.4387734459005));
#204906=CARTESIAN_POINT('Ctrl Pts',(-60.4090584186557,-81.14597687462,79.5886775666442));
#204907=CARTESIAN_POINT('Ctrl Pts',(-60.3734714868846,-82.4039286600131,
79.7822078915812));
#204908=CARTESIAN_POINT('Ctrl Pts',(-60.3550172154272,-83.0564048661365,
79.8196325925183));
#204909=CARTESIAN_POINT('Ctrl Pts',(-60.3055240991709,-84.7952387715697,
79.7534292227667));
#204910=CARTESIAN_POINT('Ctrl Pts',(-60.275748624715,-85.8689920193426,
79.5391809450683));
#204911=CARTESIAN_POINT('Ctrl Pts',(-60.2286892275973,-87.4264980060355,
78.9603211413376));
#204912=CARTESIAN_POINT('Ctrl Pts',(-60.2122723783539,-87.9464068033781,
78.7157340011332));
#204913=CARTESIAN_POINT('Ctrl Pts',(-60.181791493603,-88.88621028393,78.1731239021973));
#204914=CARTESIAN_POINT('Ctrl Pts',(-60.1676315602502,-89.3095230772174,
77.8844831166072));
#204915=CARTESIAN_POINT('Ctrl Pts',(-60.1329740426659,-90.2762019116352,
77.1134404337409));
#204916=CARTESIAN_POINT('Ctrl Pts',(-60.1123084476158,-90.7933462710861,
76.6025959711627));
#204917=CARTESIAN_POINT('Ctrl Pts',(-60.0822953265914,-91.464109478671,
75.7824723431725));
#204918=CARTESIAN_POINT('Ctrl Pts',(-60.0729376397771,-91.6631510759079,
75.513226045402));
#204919=CARTESIAN_POINT('Ctrl Pts',(-60.0454258533602,-92.2099444091266,
74.6923694872839));
#204920=CARTESIAN_POINT('Ctrl Pts',(-60.0272520902438,-92.5186744600083,
74.1167986352821));
#204921=CARTESIAN_POINT('Ctrl Pts',(-59.9952901842358,-92.9543870770854,
73.0776794715771));
#204922=CARTESIAN_POINT('Ctrl Pts',(-59.9817127483823,-93.1074215528269,
72.6272857226748));
#204923=CARTESIAN_POINT('Ctrl Pts',(-59.954926432713,-93.350009756936,71.7081280359482));
#204924=CARTESIAN_POINT('Ctrl Pts',(-59.941758434721,-93.4392147721439,
71.24046037876));
#204925=CARTESIAN_POINT('Ctrl Pts',(-59.9191599910848,-93.5351099586427,
70.437872648298));
#204926=CARTESIAN_POINT('Ctrl Pts',(-59.9098138709979,-93.5584749195833,
70.1057288119585));
#204927=CARTESIAN_POINT('Ctrl Pts',(-59.8862018942637,-93.5764556783268,
69.2711961468843));
#204928=CARTESIAN_POINT('Ctrl Pts',(-59.8718628566531,-93.5503896051845,
68.7692382533867));
#204929=CARTESIAN_POINT('Ctrl Pts',(-59.8395168809513,-93.4074846759297,
67.6347664157249));
#204930=CARTESIAN_POINT('Ctrl Pts',(-59.8218335602118,-93.2677443924347,
67.0072485059131));
#204931=CARTESIAN_POINT('Ctrl Pts',(-59.7773523524948,-92.7795652914737,
65.4984210150904));
#204932=CARTESIAN_POINT('Ctrl Pts',(-59.7502626452427,-92.3660787022586,
64.6443974106));
#204933=CARTESIAN_POINT('Ctrl Pts',(-59.7089452485442,-91.545027571265,
63.4151545487212));
#204934=CARTESIAN_POINT('Ctrl Pts',(-59.6941331228762,-91.214270189443,
62.9950532061332));
#204935=CARTESIAN_POINT('Ctrl Pts',(-59.660040108745,-90.3933564921767,
62.1050767579077));
#204936=CARTESIAN_POINT('Ctrl Pts',(-59.6406626778397,-89.8862581147153,
61.654211444381));
#204937=CARTESIAN_POINT('Ctrl Pts',(-59.6075214539216,-88.9350769997471,
60.9639061007698));
#204938=CARTESIAN_POINT('Ctrl Pts',(-59.5937295363488,-88.5109050975766,
60.7009828543388));
#204939=CARTESIAN_POINT('Ctrl Pts',(-59.5619836481251,-87.5051187295114,
60.1748196345809));
#204940=CARTESIAN_POINT('Ctrl Pts',(-59.543963217233,-86.9146733897969,
59.932891031642));
#204941=CARTESIAN_POINT('Ctrl Pts',(-59.5163445956903,-85.9858608325994,
59.6498785785385));
#204942=CARTESIAN_POINT('Ctrl Pts',(-59.5068630286917,-85.6615240423739,
59.5681462488556));
#204943=CARTESIAN_POINT('Ctrl Pts',(-59.4781411725251,-84.6566684099116,
59.3665969175512));
#204944=CARTESIAN_POINT('Ctrl Pts',(-59.459048540038,-83.9675714778447,
59.2995628231034));
#204945=CARTESIAN_POINT('Ctrl Pts',(-59.4259185777449,-82.795074324431,
59.3042570479986));
#204946=CARTESIAN_POINT('Ctrl Pts',(-59.4121692653147,-82.3139001453329,
59.3401703963216));
#204947=CARTESIAN_POINT('Ctrl Pts',(-59.3737534035655,-80.9733775652037,
59.5359101886738));
#204948=CARTESIAN_POINT('Ctrl Pts',(-59.3498274930302,-80.1293491599953,
59.7718212331793));
#204949=CARTESIAN_POINT('Ctrl Pts',(-59.2992816926066,-78.4806782000531,
60.4690792347319));
#204950=CARTESIAN_POINT('Ctrl Pts',(-59.2731736201417,-77.6876573487076,
60.9381396783424));
#204951=CARTESIAN_POINT('Ctrl Pts',(-59.2099049138779,-75.9067319761303,
62.3437746921879));
#204952=CARTESIAN_POINT('Ctrl Pts',(-59.1714264745829,-75.0218245832259,
63.3827736046064));
#204953=CARTESIAN_POINT('Ctrl Pts',(-59.1153877075156,-74.0437887948291,
65.1381830579093));
#204954=CARTESIAN_POINT('Ctrl Pts',(-59.0969999696884,-73.7796585481076,
65.742394789452));
#204955=CARTESIAN_POINT('Ctrl Pts',(-59.0603571635507,-73.3787293450233,
66.9690057963436));
#204956=CARTESIAN_POINT('Ctrl Pts',(-59.0423634327771,-73.2382779305409,
67.5871900361875));
#204957=CARTESIAN_POINT('Ctrl Pts',(-59.0155634689847,-73.1129690606558,
68.5390171613752));
#204958=CARTESIAN_POINT('Ctrl Pts',(-59.0064538880824,-73.0858103549134,
68.8655272988062));
#204959=CARTESIAN_POINT('Ctrl Pts',(-58.9661357929594,-73.0353080704403,
70.3046748358551));
#204960=CARTESIAN_POINT('Ctrl Pts',(-58.9343155934815,-73.1775838491939,
71.4155416553419));
#204961=CARTESIAN_POINT('Ctrl Pts',(-58.8935634968148,-73.5951978839729,
72.8157920654114));
#204962=CARTESIAN_POINT('Ctrl Pts',(-58.8838562465419,-73.7117537529889,
73.1443725421251));
#204963=CARTESIAN_POINT('Ctrl Pts',(-58.8740778711611,-73.8447192590796,
73.4662010349383));
#204964=CARTESIAN_POINT('Origin',(-45.8894114130409,-83.3180213346267,69.5522455184007));
#204965=CARTESIAN_POINT('',(-62.9075068658247,-73.8447192590796,73.4662010349382));
#204966=CARTESIAN_POINT('',(-62.5017927897014,-73.8447192658252,73.4662010512653));
#204967=CARTESIAN_POINT('',(-45.8894114130409,-73.8447192590796,73.4662010349383));
#204968=CARTESIAN_POINT('',(-62.1255498668003,-93.5595364804028,69.970346919323));
#204969=CARTESIAN_POINT('Ctrl Pts',(-62.9075068658247,-73.8447192590795,
73.4662010349381));
#204970=CARTESIAN_POINT('Ctrl Pts',(-62.8890297137548,-74.0941098645064,
74.0698237715866));
#204971=CARTESIAN_POINT('Ctrl Pts',(-62.8709501951455,-74.4006222769129,
74.6482296293146));
#204972=CARTESIAN_POINT('Ctrl Pts',(-62.8346556323582,-75.1175005308676,
75.7357486846773));
#204973=CARTESIAN_POINT('Ctrl Pts',(-62.816127299745,-75.5256433516957,
76.2427667065413));
#204974=CARTESIAN_POINT('Ctrl Pts',(-62.7595831183316,-76.9123795088531,
77.6650712602952));
#204975=CARTESIAN_POINT('Ctrl Pts',(-62.7232980830352,-78.0241240009392,
78.4305795136538));
#204976=CARTESIAN_POINT('Ctrl Pts',(-62.6471481891126,-80.4749509242041,
79.4898561694312));
#204977=CARTESIAN_POINT('Ctrl Pts',(-62.6109576119547,-81.7899614573926,
79.7749756124774));
#204978=CARTESIAN_POINT('Ctrl Pts',(-62.5541063933797,-83.787779249665,
79.8130641293939));
#204979=CARTESIAN_POINT('Ctrl Pts',(-62.5351119019629,-84.4525860097568,
79.760960059608));
#204980=CARTESIAN_POINT('Ctrl Pts',(-62.4978581696944,-85.7602341430177,
79.5290869291398));
#204981=CARTESIAN_POINT('Ctrl Pts',(-62.4796746883654,-86.4000600770917,
79.3503470402618));
#204982=CARTESIAN_POINT('Ctrl Pts',(-62.4424295539205,-87.6317020290275,
78.8735937106281));
#204983=CARTESIAN_POINT('Ctrl Pts',(-62.4235188596297,-88.2209803079372,
78.5775642584995));
#204984=CARTESIAN_POINT('Ctrl Pts',(-62.3861515017277,-89.3406245664244,
77.8728813615582));
#204985=CARTESIAN_POINT('Ctrl Pts',(-62.3677920367359,-89.8676274107198,
77.4647286706258));
#204986=CARTESIAN_POINT('Ctrl Pts',(-62.3306363167816,-90.8357688888216,
76.5514880424947));
#204987=CARTESIAN_POINT('Ctrl Pts',(-62.3115449033513,-91.2744815876631,
76.0484475302656));
#204988=CARTESIAN_POINT('Ctrl Pts',(-62.2644735866283,-92.2367689999472,
74.7000482335409));
#204989=CARTESIAN_POINT('Ctrl Pts',(-62.237467135121,-92.6923052269227,
73.8144878831633));
#204990=CARTESIAN_POINT('Ctrl Pts',(-62.1815044190819,-93.3352043397708,
71.9398912558015));
#204991=CARTESIAN_POINT('Ctrl Pts',(-62.1531555603415,-93.5190613500812,
70.9606701984125));
#204992=CARTESIAN_POINT('Ctrl Pts',(-62.1255316836823,-93.5594905838186,
69.9703455277973));
#204993=CARTESIAN_POINT('Ctrl Pts',(-61.0939133588288,-73.8447192590796,
73.4662010349383));
#204994=CARTESIAN_POINT('Ctrl Pts',(-61.0972755292109,-73.7995412893984,
73.356852691008));
#204995=CARTESIAN_POINT('Ctrl Pts',(-61.1006343640762,-73.7562441228431,
73.2466919441307));
#204996=CARTESIAN_POINT('Ctrl Pts',(-61.1224071184744,-73.4871979595048,
72.5256982249987));
#204997=CARTESIAN_POINT('Ctrl Pts',(-61.1403527106327,-73.3181970944473,
71.8953260594235));
#204998=CARTESIAN_POINT('Ctrl Pts',(-61.1775605622687,-73.098118251332,
70.587507381851));
#204999=CARTESIAN_POINT('Ctrl Pts',(-61.1967979414229,-73.052132641733,
69.9123831679951));
#205000=CARTESIAN_POINT('Ctrl Pts',(-61.2402988666641,-73.0992182659107,
68.3788970089533));
#205001=CARTESIAN_POINT('Ctrl Pts',(-61.2638572963438,-73.2334570554963,
67.5268448741542));
#205002=CARTESIAN_POINT('Ctrl Pts',(-61.3137826779292,-73.7253916735425,
65.8278126755097));
#205003=CARTESIAN_POINT('Ctrl Pts',(-61.3397066335119,-74.0935684710335,
64.9916059948674));
#205004=CARTESIAN_POINT('Ctrl Pts',(-61.4027530430455,-75.2707843617758,
63.0614753140105));
#205005=CARTESIAN_POINT('Ctrl Pts',(-61.4412152659376,-76.1955325584022,
62.0583624016276));
#205006=CARTESIAN_POINT('Ctrl Pts',(-61.4971523997589,-77.8173921947074,
60.8784979180106));
#205007=CARTESIAN_POINT('Ctrl Pts',(-61.5154210351218,-78.3822816998748,
60.5450659144375));
#205008=CARTESIAN_POINT('Ctrl Pts',(-61.5518901541755,-79.5463008162671,
60.0005807093627));
#205009=CARTESIAN_POINT('Ctrl Pts',(-61.5698612016951,-80.1409618991759,
59.7866688915264));
#205010=CARTESIAN_POINT('Ctrl Pts',(-61.6052068932917,-81.3660595803169,
59.4698207635543));
#205011=CARTESIAN_POINT('Ctrl Pts',(-61.6228341737123,-81.9940518549715,
59.3683098329066));
#205012=CARTESIAN_POINT('Ctrl Pts',(-61.6549628277035,-83.1273207365526,
59.2917772992746));
#205013=CARTESIAN_POINT('Ctrl Pts',(-61.6692758998122,-83.6290562963196,
59.2947200422361));
#205014=CARTESIAN_POINT('Ctrl Pts',(-61.7017999922263,-84.77506317455,59.3856271790135));
#205015=CARTESIAN_POINT('Ctrl Pts',(-61.7196746168933,-85.4152409850817,
59.4981532587356));
#205016=CARTESIAN_POINT('Ctrl Pts',(-61.7639923205417,-86.9382214783504,
59.9177370281428));
#205017=CARTESIAN_POINT('Ctrl Pts',(-61.7907068925564,-87.798079577134,
60.2862491473952));
#205018=CARTESIAN_POINT('Ctrl Pts',(-61.8308005140353,-89.0273972914217,
61.0247355433965));
#205019=CARTESIAN_POINT('Ctrl Pts',(-61.8447519131577,-89.4388416258829,
61.3150761380113));
#205020=CARTESIAN_POINT('Ctrl Pts',(-61.877891718036,-90.3493249207702,
62.0635913641212));
#205021=CARTESIAN_POINT('Ctrl Pts',(-61.8972052867198,-90.8276155890008,
62.5433119093223));
#205022=CARTESIAN_POINT('Ctrl Pts',(-61.9334581013333,-91.6389705443853,
63.5362534302575));
#205023=CARTESIAN_POINT('Ctrl Pts',(-61.9501942467327,-91.9802953089516,
64.0390460305397));
#205024=CARTESIAN_POINT('Ctrl Pts',(-61.9931785862009,-92.7259061778884,
65.3792607709462));
#205025=CARTESIAN_POINT('Ctrl Pts',(-62.0197789243641,-93.0646448459485,
66.2468816466174));
#205026=CARTESIAN_POINT('Ctrl Pts',(-62.0588455447749,-93.3920095183979,
67.6036950542001));
#205027=CARTESIAN_POINT('Ctrl Pts',(-62.0718370519845,-93.4705497370475,
68.0662255956203));
#205028=CARTESIAN_POINT('Ctrl Pts',(-62.0984431327042,-93.5649315281472,
69.0102031279554));
#205029=CARTESIAN_POINT('Ctrl Pts',(-62.1120352760041,-93.5790729419953,
69.4906655321689));
#205030=CARTESIAN_POINT('Ctrl Pts',(-62.1256936736043,-93.5594907615313,
69.9703411746549));
#205031=CARTESIAN_POINT('Ctrl Pts',(-62.5017927901943,-73.8447192658304,
73.466201051278));
#205032=CARTESIAN_POINT('Ctrl Pts',(-62.4841847932971,-74.0855314753815,
74.0490607142885));
#205033=CARTESIAN_POINT('Ctrl Pts',(-62.4666545746529,-74.3796576838083,
74.608539247783));
#205034=CARTESIAN_POINT('Ctrl Pts',(-62.4394720039789,-74.9030783441912,
75.4139829192377));
#205035=CARTESIAN_POINT('Ctrl Pts',(-62.4300873205818,-75.0959934428049,
75.6816408449356));
#205036=CARTESIAN_POINT('Ctrl Pts',(-62.3906602265135,-75.9599741494087,
76.7660047698653));
#205037=CARTESIAN_POINT('Ctrl Pts',(-62.3617397936393,-76.7423395887225,
77.4856935935262));
#205038=CARTESIAN_POINT('Ctrl Pts',(-62.3225114354629,-77.8942276034712,
78.2558738490049));
#205039=CARTESIAN_POINT('Ctrl Pts',(-62.3131477738994,-78.1762943169244,
78.4254257130088));
#205040=CARTESIAN_POINT('Ctrl Pts',(-62.2743741082159,-79.3775580116726,
79.0709689990103));
#205041=CARTESIAN_POINT('Ctrl Pts',(-62.2460503879043,-80.3580374681057,
79.4199630804335));
#205042=CARTESIAN_POINT('Ctrl Pts',(-62.2074372133845,-81.6976361070693,
79.6787181434111));
#205043=CARTESIAN_POINT('Ctrl Pts',(-62.1980576697969,-82.0240197146451,
79.7255760830527));
#205044=CARTESIAN_POINT('Ctrl Pts',(-62.1587914746783,-83.3987458291229,
79.8557054367172));
#205045=CARTESIAN_POINT('Ctrl Pts',(-62.1300181568743,-84.4544380023431,
79.7931618537553));
#205046=CARTESIAN_POINT('Ctrl Pts',(-62.0855312849989,-85.9905269512449,
79.4613724502301));
#205047=CARTESIAN_POINT('Ctrl Pts',(-62.0706589776804,-86.4898777562472,
79.3130040452828));
#205048=CARTESIAN_POINT('Ctrl Pts',(-62.0466231600363,-87.28554034407,79.0090542175185));
#205049=CARTESIAN_POINT('Ctrl Pts',(-62.0373902278873,-87.5893541668113,
78.8757724680081));
#205050=CARTESIAN_POINT('Ctrl Pts',(-61.9904527351222,-89.09610785971,78.1256345376654));
#205051=CARTESIAN_POINT('Ctrl Pts',(-61.951973712199,-90.1750339007047,
77.2898589653742));
#205052=CARTESIAN_POINT('Ctrl Pts',(-61.8792605949586,-91.8836561409898,
75.3202275397201));
#205053=CARTESIAN_POINT('Ctrl Pts',(-61.8434485105681,-92.5252913279683,
74.2283448200108));
#205054=CARTESIAN_POINT('Ctrl Pts',(-61.7895069237388,-93.1837604232446,
72.4132391565384));
#205055=CARTESIAN_POINT('Ctrl Pts',(-61.7707654980411,-93.3507060338506,
71.7575408245925));
#205056=CARTESIAN_POINT('Ctrl Pts',(-61.7325189893887,-93.5533519612268,
70.4222640392778));
#205057=CARTESIAN_POINT('Ctrl Pts',(-61.7132059380748,-93.5884366430676,
69.7459250868423));
#205058=CARTESIAN_POINT('Ctrl Pts',(-61.6754557091104,-93.5250454819414,
68.3970701948348));
#205059=CARTESIAN_POINT('Ctrl Pts',(-61.6567438364296,-93.4268963238492,
67.727850414592));
#205060=CARTESIAN_POINT('Ctrl Pts',(-61.6283187645921,-93.1839472020908,
66.7531845002519));
#205061=CARTESIAN_POINT('Ctrl Pts',(-61.6189338943095,-93.0887989606251,
66.4372592869426));
#205062=CARTESIAN_POINT('Ctrl Pts',(-61.5795009251722,-92.6253410740485,
65.1303232177303));
#205063=CARTESIAN_POINT('Ctrl Pts',(-61.5505751177801,-92.1201334356208,
64.194780818897));
#205064=CARTESIAN_POINT('Ctrl Pts',(-61.5113412268191,-91.281979225922,
63.0911267564976));
#205065=CARTESIAN_POINT('Ctrl Pts',(-61.5019777055676,-91.0705636445477,
62.8389179069684));
#205066=CARTESIAN_POINT('Ctrl Pts',(-61.4632083833256,-90.1453340345577,
61.8372699653512));
#205067=CARTESIAN_POINT('Ctrl Pts',(-61.4348886239657,-89.3322286570764,
61.1878947823721));
#205068=CARTESIAN_POINT('Ctrl Pts',(-61.3907373814084,-87.9805507160714,
60.4089783600418));
#205069=CARTESIAN_POINT('Ctrl Pts',(-61.3757161999373,-87.505859075302,
60.1820519947092));
#205070=CARTESIAN_POINT('Ctrl Pts',(-61.3515272274868,-86.7065344518898,
59.8728609480731));
#205071=CARTESIAN_POINT('Ctrl Pts',(-61.3422905309527,-86.3915729733846,
59.7682898692625));
#205072=CARTESIAN_POINT('Ctrl Pts',(-61.2953514805828,-84.7702512509659,
59.3160254008778));
#205073=CARTESIAN_POINT('Ctrl Pts',(-61.2568735915856,-83.4093454335768,
59.2139267594145));
#205074=CARTESIAN_POINT('Ctrl Pts',(-61.1815476021197,-80.7283712650494,
59.5433686192169));
#205075=CARTESIAN_POINT('Ctrl Pts',(-61.1431283745384,-79.4344568146368,
59.9709177871001));
#205076=CARTESIAN_POINT('Ctrl Pts',(-61.0879192659949,-77.7127072891277,
60.9476124636147));
#205077=CARTESIAN_POINT('Ctrl Pts',(-61.070345096222,-77.1946513438504,
61.3082423398081));
#205078=CARTESIAN_POINT('Ctrl Pts',(-61.0381959870421,-76.3277426502109,
62.0387705491118));
#205079=CARTESIAN_POINT('Ctrl Pts',(-61.023791336302,-75.9669566102274,
62.3913690533349));
#205080=CARTESIAN_POINT('Ctrl Pts',(-60.9948506651892,-75.2863030073976,
63.1624605811165));
#205081=CARTESIAN_POINT('Ctrl Pts',(-60.980338142677,-74.9697649554248,
63.5819463534444));
#205082=CARTESIAN_POINT('Ctrl Pts',(-60.9477026164546,-74.341455457925,
64.5628978746868));
#205083=CARTESIAN_POINT('Ctrl Pts',(-60.9295233279679,-74.0474347307934,
65.1331353657493));
#205084=CARTESIAN_POINT('Ctrl Pts',(-60.8933588822817,-73.5725602068601,
66.3136804132178));
#205085=CARTESIAN_POINT('Ctrl Pts',(-60.8757973656961,-73.3913769943919,
66.9208860112263));
#205086=CARTESIAN_POINT('Ctrl Pts',(-60.8397638220275,-73.1382738855007,
68.1856499340229));
#205087=CARTESIAN_POINT('Ctrl Pts',(-60.8211917494364,-73.0715879518112,
68.841309849744));
#205088=CARTESIAN_POINT('Ctrl Pts',(-60.7640366499264,-73.0611151385496,
70.8504175195901));
#205089=CARTESIAN_POINT('Ctrl Pts',(-60.7271143757618,-73.3214825470434,
72.1901587832426));
#205090=CARTESIAN_POINT('Ctrl Pts',(-60.6884024535279,-73.8377218668054,
73.4492323338641));
#205091=CARTESIAN_POINT('Ctrl Pts',(-60.6881413650971,-73.8412149656867,
73.4577192753012));
#205092=CARTESIAN_POINT('Ctrl Pts',(-60.6878802914039,-73.8447192570083,
73.466201029925));
#205093=CARTESIAN_POINT('Origin',(-21.6548258024609,-75.,72.98888938658));
#205094=CARTESIAN_POINT('',(-23.7494631149408,-62.9850802834321,77.9529305028911));
#205095=CARTESIAN_POINT('',(-23.5675316904177,-62.985080294536,77.9529305294611));
#205096=CARTESIAN_POINT('',(-21.6548258024609,-62.9850802944281,77.9529305295057));
#205097=CARTESIAN_POINT('',(-23.5675316903009,-68.1939482861969,84.0648841531478));
#205098=CARTESIAN_POINT('Ctrl Pts',(-23.7494631142981,-62.9850802834266,
77.9529305028778));
#205099=CARTESIAN_POINT('Ctrl Pts',(-23.7335469728175,-63.2572812599135,
78.611763256806));
#205100=CARTESIAN_POINT('Ctrl Pts',(-23.7173356484375,-63.583267752548,
79.2472274989783));
#205101=CARTESIAN_POINT('Ctrl Pts',(-23.6789660693081,-64.4896165551071,
80.7050232770356));
#205102=CARTESIAN_POINT('Ctrl Pts',(-23.6573462260849,-65.1163076778375,
81.4929757686019));
#205103=CARTESIAN_POINT('Ctrl Pts',(-23.6129675706434,-66.5413261017482,
82.9118922601765));
#205104=CARTESIAN_POINT('Ctrl Pts',(-23.5899173818356,-67.3355222961797,
83.5373927807101));
#205105=CARTESIAN_POINT('Ctrl Pts',(-23.5675316903009,-68.1939482861969,
84.0648841531478));
#205106=CARTESIAN_POINT('Origin',(-23.5675316903009,-75.,72.98888938658));
#205107=CARTESIAN_POINT('Origin',(-21.6548258024609,-75.,72.98888938658));
#205108=CARTESIAN_POINT('',(-25.5628518781596,-62.9850802944281,77.9529305295057));
#205109=CARTESIAN_POINT('',(-25.2581222247366,-62.9850802944281,77.9529305295057));
#205110=CARTESIAN_POINT('',(-21.6548258024609,-62.9850802944281,77.9529305295057));
#205111=CARTESIAN_POINT('Ctrl Pts',(-25.5628518781596,-62.9850802944281,
77.9529305295057));
#205112=CARTESIAN_POINT('Ctrl Pts',(-25.5342348853663,-63.4755910199596,
79.1401581958963));
#205113=CARTESIAN_POINT('Ctrl Pts',(-25.5067802221842,-64.1402777289051,
80.2502980014423));
#205114=CARTESIAN_POINT('Ctrl Pts',(-25.4598723099547,-65.4624900254345,
81.8581750998699));
#205115=CARTESIAN_POINT('Ctrl Pts',(-25.4420110595249,-66.0209090968996,
82.4230970114663));
#205116=CARTESIAN_POINT('Ctrl Pts',(-25.4061623457359,-67.2631855963744,
83.468998148917));
#205117=CARTESIAN_POINT('Ctrl Pts',(-25.3882919641257,-67.948955156665,
83.9421414655667));
#205118=CARTESIAN_POINT('Ctrl Pts',(-25.3604186304515,-69.0425151706589,
84.5511188474739));
#205119=CARTESIAN_POINT('Ctrl Pts',(-25.3509160417769,-69.4195525323061,
84.7377352997636));
#205120=CARTESIAN_POINT('Ctrl Pts',(-25.3031624035224,-71.3605130656141,
85.5838769037993));
#205121=CARTESIAN_POINT('Ctrl Pts',(-25.2671492367614,-73.0338876517155,
85.9509106010213));
#205122=CARTESIAN_POINT('Ctrl Pts',(-25.211093783332,-75.5211982206036,
86.0024934260272));
#205123=CARTESIAN_POINT('Ctrl Pts',(-25.1932702125315,-76.3117954672579,
85.9466959719248));
#205124=CARTESIAN_POINT('Ctrl Pts',(-25.1573545097553,-77.9173095201321,
85.6848678053003));
#205125=CARTESIAN_POINT('Ctrl Pts',(-25.1393881007222,-78.7273131421505,
85.4711042328601));
#205126=CARTESIAN_POINT('Ctrl Pts',(-25.1114105692348,-79.905454109883,
85.035186013571));
#205127=CARTESIAN_POINT('Ctrl Pts',(-25.1019084706642,-80.2924279850967,
84.8702591362598));
#205128=CARTESIAN_POINT('Ctrl Pts',(-25.0541466985092,-82.1980757005559,
83.9464752146254));
#205129=CARTESIAN_POINT('Ctrl Pts',(-25.0181261672443,-83.5657348334043,
82.9140686343907));
#205130=CARTESIAN_POINT('Ctrl Pts',(-24.9617637202305,-85.2318804993534,
81.0483612746309));
#205131=CARTESIAN_POINT('Ctrl Pts',(-24.9436507628792,-85.710654373767,
80.4002570731339));
#205132=CARTESIAN_POINT('Ctrl Pts',(-24.9079838183037,-86.5466312994028,
79.0167666311897));
#205133=CARTESIAN_POINT('Ctrl Pts',(-24.8905073373037,-86.9006753634193,
78.2835953282236));
#205134=CARTESIAN_POINT('Ctrl Pts',(-24.8630645895268,-87.3306440284148,
77.1279872899302));
#205135=CARTESIAN_POINT('Ctrl Pts',(-24.8535596220528,-87.4580993038288,
76.7268933833987));
#205136=CARTESIAN_POINT('Ctrl Pts',(-24.8058503480045,-88.0001699063287,
74.6822528929101));
#205137=CARTESIAN_POINT('Ctrl Pts',(-24.7698813216615,-88.1099855999607,
72.9749547963028));
#205138=CARTESIAN_POINT('Ctrl Pts',(-24.7143843430216,-87.7889354780213,
70.5324051813258));
#205139=CARTESIAN_POINT('Ctrl Pts',(-24.6970419222637,-87.6212985854423,
69.7804588734143));
#205140=CARTESIAN_POINT('Ctrl Pts',(-24.6632901642082,-87.1584529888661,
68.3255961552898));
#205141=CARTESIAN_POINT('Ctrl Pts',(-24.6469281069572,-86.8660070905663,
67.6249218798878));
#205142=CARTESIAN_POINT('Ctrl Pts',(-24.6085627568924,-86.0594517133163,
66.0861333089881));
#205143=CARTESIAN_POINT('Ctrl Pts',(-24.586160384182,-85.5081015734761,
65.2727174091092));
#205144=CARTESIAN_POINT('Ctrl Pts',(-24.5478929218035,-84.3881486354314,
63.9660075581999));
#205145=CARTESIAN_POINT('Ctrl Pts',(-24.5317890202234,-83.8583716408209,
63.4453584440213));
#205146=CARTESIAN_POINT('Ctrl Pts',(-24.4786780417851,-81.9915516088788,
61.9008022575739));
#205147=CARTESIAN_POINT('Ctrl Pts',(-24.4404197776329,-80.5002502188647,
61.0903726254298));
#205148=CARTESIAN_POINT('Ctrl Pts',(-24.3944539989605,-78.4940872446607,
60.46016793533));
#205149=CARTESIAN_POINT('Ctrl Pts',(-24.3852625240197,-78.0862384647128,
60.3535169796922));
#205150=CARTESIAN_POINT('Ctrl Pts',(-24.3589735379833,-76.9284736377242,
60.110176267431));
#205151=CARTESIAN_POINT('Ctrl Pts',(-24.3416198348966,-76.170680721155,
60.0193181026919));
#205152=CARTESIAN_POINT('Ctrl Pts',(-24.315347669909,-74.9965402900159,
59.9823322175876));
#205153=CARTESIAN_POINT('Ctrl Pts',(-24.3062012240958,-74.5833920590936,
59.9890054637237));
#205154=CARTESIAN_POINT('Ctrl Pts',(-24.2791962632358,-73.3574014902427,
60.0673205172551));
#205155=CARTESIAN_POINT('Ctrl Pts',(-24.2616122208315,-72.5502449644129,
60.1957750471281));
#205156=CARTESIAN_POINT('Ctrl Pts',(-24.2174452577431,-70.6413697835284,
60.6869544138998));
#205157=CARTESIAN_POINT('Ctrl Pts',(-24.1913574606361,-69.5656309742676,
61.1228465529577));
#205158=CARTESIAN_POINT('Ctrl Pts',(-24.148103015785,-67.8509316396604,
62.1003517955149));
#205159=CARTESIAN_POINT('Ctrl Pts',(-24.1303270077391,-67.1799782752499,
62.5717550113518));
#205160=CARTESIAN_POINT('Ctrl Pts',(-24.0934607218758,-65.9342632283519,
63.6355618776124));
#205161=CARTESIAN_POINT('Ctrl Pts',(-24.0749439293734,-65.3625008128495,
64.2258447186017));
#205162=CARTESIAN_POINT('Ctrl Pts',(-24.0399256256379,-64.3721660207933,
65.4633093764349));
#205163=CARTESIAN_POINT('Ctrl Pts',(-24.0234209550608,-63.9478296127134,
66.1016021098746));
#205164=CARTESIAN_POINT('Ctrl Pts',(-23.9864808616788,-63.1492334947361,
67.5686511770807));
#205165=CARTESIAN_POINT('Ctrl Pts',(-23.9657965863761,-62.8006300155267,
68.4068572518267));
#205166=CARTESIAN_POINT('Ctrl Pts',(-23.928675173025,-62.3247219460287,
70.0030333536306));
#205167=CARTESIAN_POINT('Ctrl Pts',(-23.9121337744945,-62.1718251405703,
70.7492595751274));
#205168=CARTESIAN_POINT('Ctrl Pts',(-23.8584168754266,-61.8917373511402,
73.1862692369497));
#205169=CARTESIAN_POINT('Ctrl Pts',(-23.8198811582598,-62.0287767524375,
74.8896421089106));
#205170=CARTESIAN_POINT('Ctrl Pts',(-23.7736771942405,-62.6026642094907,
76.9237439180875));
#205171=CARTESIAN_POINT('Ctrl Pts',(-23.7645045072629,-62.7364962506747,
77.3228814711087));
#205172=CARTESIAN_POINT('Ctrl Pts',(-23.7532764802333,-62.9205454775805,
77.7945212353098));
#205173=CARTESIAN_POINT('Ctrl Pts',(-23.7513724844866,-62.9524258595896,
77.8738940340813));
#205174=CARTESIAN_POINT('Ctrl Pts',(-23.7494631142981,-62.9850802834266,
77.9529305028778));
#205175=CARTESIAN_POINT('',(-23.5675316904176,-62.0095472178182,72.4907563613072));
#205176=CARTESIAN_POINT('Origin',(-23.5675316903009,-75.,72.98888938658));
#205177=CARTESIAN_POINT('',(-23.5676924422401,-62.0098217648708,72.4836474449556));
#205178=CARTESIAN_POINT('Ctrl Pts',(-23.5675316904176,-62.0095472178182,
72.4907563613072));
#205179=CARTESIAN_POINT('Ctrl Pts',(-23.5675873235413,-62.0095822026889,
72.488392133029));
#205180=CARTESIAN_POINT('Ctrl Pts',(-23.5676429566649,-62.0096178329842,
72.4860278991301));
#205181=CARTESIAN_POINT('Ctrl Pts',(-23.5676985897885,-62.0096541087152,
72.483663659963));
#205182=CARTESIAN_POINT('',(-24.3504740810588,-87.0149185312533,68.0248454013453));
#205183=CARTESIAN_POINT('Ctrl Pts',(-23.5676924422401,-62.0098217648708,
72.4836474449556));
#205184=CARTESIAN_POINT('Ctrl Pts',(-23.579866516381,-62.0307601264892,
71.9453052627917));
#205185=CARTESIAN_POINT('Ctrl Pts',(-23.5921363130452,-62.0851436237892,
71.4087819670163));
#205186=CARTESIAN_POINT('Ctrl Pts',(-23.6163677338717,-62.2602046232303,
70.3453912998643));
#205187=CARTESIAN_POINT('Ctrl Pts',(-23.6283050919866,-62.3807372772904,
69.8195543991636));
#205188=CARTESIAN_POINT('Ctrl Pts',(-23.6548809171447,-62.7250745080482,
68.6550241764099));
#205189=CARTESIAN_POINT('Ctrl Pts',(-23.6693811451348,-62.9667724226921,
68.0232469123233));
#205190=CARTESIAN_POINT('Ctrl Pts',(-23.7137157498716,-63.827887483909,
66.2095881368179));
#205191=CARTESIAN_POINT('Ctrl Pts',(-23.744493151187,-64.5809484779854,
65.1010209222292));
#205192=CARTESIAN_POINT('Ctrl Pts',(-23.7829206451027,-65.7754626425724,
63.8191474354444));
#205193=CARTESIAN_POINT('Ctrl Pts',(-23.7920271109958,-66.0763872068843,
63.5260466635872));
#205194=CARTESIAN_POINT('Ctrl Pts',(-23.8386873210014,-67.6838550110502,
62.1053575149547));
#205195=CARTESIAN_POINT('Ctrl Pts',(-23.8784725722723,-69.1913825338534,
61.2314571897476));
#205196=CARTESIAN_POINT('Ctrl Pts',(-23.9304375078448,-71.4432011399058,
60.4679211891803));
#205197=CARTESIAN_POINT('Ctrl Pts',(-23.944451268879,-72.075814484835,60.3052546592798));
#205198=CARTESIAN_POINT('Ctrl Pts',(-23.9734151603135,-73.3657868000052,
60.0752384248514));
#205199=CARTESIAN_POINT('Ctrl Pts',(-23.9884516930089,-74.021451081523,
60.009079728374));
#205200=CARTESIAN_POINT('Ctrl Pts',(-24.0419614354673,-76.3858270044576,
59.9507329783212));
#205201=CARTESIAN_POINT('Ctrl Pts',(-24.0776364421922,-78.0840502811192,
60.2451583872043));
#205202=CARTESIAN_POINT('Ctrl Pts',(-24.1335183165893,-80.3902635205254,
61.1343653793985));
#205203=CARTESIAN_POINT('Ctrl Pts',(-24.1509196237142,-81.0780618491765,
61.4718643510552));
#205204=CARTESIAN_POINT('Ctrl Pts',(-24.191975435258,-82.6591166877362,
62.4289671184892));
#205205=CARTESIAN_POINT('Ctrl Pts',(-24.2148896691125,-83.5122415194365,
63.1037622587596));
#205206=CARTESIAN_POINT('Ctrl Pts',(-24.253375992345,-84.721255369222,64.33392126898));
#205207=CARTESIAN_POINT('Ctrl Pts',(-24.2680418990414,-85.1363207939457,
64.8239471121187));
#205208=CARTESIAN_POINT('Ctrl Pts',(-24.2940935767868,-85.8152657536147,
65.7574852536921));
#205209=CARTESIAN_POINT('Ctrl Pts',(-24.3055351499505,-86.0921844738963,
66.1898725772783));
#205210=CARTESIAN_POINT('Ctrl Pts',(-24.3281398473406,-86.5941062081981,
67.0862442270561));
#205211=CARTESIAN_POINT('Ctrl Pts',(-24.3392828333263,-86.8185276235538,
67.5495029661639));
#205212=CARTESIAN_POINT('Ctrl Pts',(-24.3504740810588,-87.0149185312533,
68.0248454013453));
#205213=CARTESIAN_POINT('Ctrl Pts',(-25.2581222247366,-62.9850802944281,
77.9529305295057));
#205214=CARTESIAN_POINT('Ctrl Pts',(-25.2371139399055,-63.3447308264597,
78.8234253823906));
#205215=CARTESIAN_POINT('Ctrl Pts',(-25.2154096398342,-63.7981918152589,
79.6529161930109));
#205216=CARTESIAN_POINT('Ctrl Pts',(-25.1819196289562,-64.660700850565,
80.889351340767));
#205217=CARTESIAN_POINT('Ctrl Pts',(-25.1697456138254,-65.0133303636238,
81.3306425360379));
#205218=CARTESIAN_POINT('Ctrl Pts',(-25.1201329901734,-66.5490449435483,
83.0149971167249));
#205219=CARTESIAN_POINT('Ctrl Pts',(-25.0805800079473,-67.9440247118269,
84.0412504740234));
#205220=CARTESIAN_POINT('Ctrl Pts',(-25.0292609529502,-70.0720240720413,
85.0353238642883));
#205221=CARTESIAN_POINT('Ctrl Pts',(-25.0156013108122,-70.6649759484139,
85.2611792869093));
#205222=CARTESIAN_POINT('Ctrl Pts',(-24.9750095399071,-72.4326606250719,
85.790316577514));
#205223=CARTESIAN_POINT('Ctrl Pts',(-24.9470863164347,-73.6361435723789,
85.9737863081481));
#205224=CARTESIAN_POINT('Ctrl Pts',(-24.9074472810636,-75.4215878797593,
85.994728634871));
#205225=CARTESIAN_POINT('Ctrl Pts',(-24.8950686466218,-75.9954684441146,
85.9634276729296));
#205226=CARTESIAN_POINT('Ctrl Pts',(-24.8452804596558,-78.2654540971995,
85.6880829550959));
#205227=CARTESIAN_POINT('Ctrl Pts',(-24.805767495012,-79.9081112242142,
85.1479662718454));
#205228=CARTESIAN_POINT('Ctrl Pts',(-24.7535182298214,-81.9910126324009,
83.9701726844078));
#205229=CARTESIAN_POINT('Ctrl Pts',(-24.7388535666975,-82.5560153403092,
83.5893363069171));
#205230=CARTESIAN_POINT('Ctrl Pts',(-24.69867188384,-83.9815521110443,82.4563454225764));
#205231=CARTESIAN_POINT('Ctrl Pts',(-24.6723892454678,-84.777191987148,
81.632234791459));
#205232=CARTESIAN_POINT('Ctrl Pts',(-24.6343728549608,-85.7938596513943,
80.2564610504218));
#205233=CARTESIAN_POINT('Ctrl Pts',(-24.6220757074884,-86.1021482587485,
79.7761802699739));
#205234=CARTESIAN_POINT('Ctrl Pts',(-24.5723410169992,-87.207375182649,
77.7764145952943));
#205235=CARTESIAN_POINT('Ctrl Pts',(-24.5327923771456,-87.7317495103957,
76.1262380632064));
#205236=CARTESIAN_POINT('Ctrl Pts',(-24.4727154955423,-88.0348717464135,
73.3931830848306));
#205237=CARTESIAN_POINT('Ctrl Pts',(-24.4504231768756,-88.0257007641021,
72.3544900133169));
#205238=CARTESIAN_POINT('Ctrl Pts',(-24.4014705356493,-87.7472570708071,
70.1930457333697));
#205239=CARTESIAN_POINT('Ctrl Pts',(-24.3753730910703,-87.4518616937928,
69.0824179201051));
#205240=CARTESIAN_POINT('Ctrl Pts',(-24.3504740810588,-87.0149185312533,
68.0248454013453));
#205241=CARTESIAN_POINT('Origin',(-21.6548258024609,-75.,72.98888938658));
#205242=CARTESIAN_POINT('',(-27.3772428998354,-62.9850802944281,77.9529305295057));
#205243=CARTESIAN_POINT('',(-27.071820154481,-62.9850802944281,77.9529305295057));
#205244=CARTESIAN_POINT('',(-21.6548258024609,-62.9850802944281,77.9529305295057));
#205245=CARTESIAN_POINT('',(-25.7929126252424,-63.0439273290319,67.8848479330954));
#205246=CARTESIAN_POINT('Ctrl Pts',(-27.3772428998354,-62.9850802944281,
77.9529305295057));
#205247=CARTESIAN_POINT('Ctrl Pts',(-27.3629199848378,-63.2318120975808,
78.5501179254876));
#205248=CARTESIAN_POINT('Ctrl Pts',(-27.3487777117857,-63.522825092598,
79.1283224359325));
#205249=CARTESIAN_POINT('Ctrl Pts',(-27.3167432374599,-64.2661879682576,
80.3659152905382));
#205250=CARTESIAN_POINT('Ctrl Pts',(-27.2988078339567,-64.7385404670655,
81.0099670876734));
#205251=CARTESIAN_POINT('Ctrl Pts',(-27.2639533653288,-65.7802537363062,
82.1864972295272));
#205252=CARTESIAN_POINT('Ctrl Pts',(-27.2470572222126,-66.3443972388745,
82.7192671324979));
#205253=CARTESIAN_POINT('Ctrl Pts',(-27.2168589103768,-67.4082327315602,
83.5577899268292));
#205254=CARTESIAN_POINT('Ctrl Pts',(-27.2038385483791,-67.8874041893299,
83.8860253769056));
#205255=CARTESIAN_POINT('Ctrl Pts',(-27.1718068558823,-69.1270605223102,
84.6184935410882));
#205256=CARTESIAN_POINT('Ctrl Pts',(-27.153075301976,-69.9087850165376,
84.9813302386246));
#205257=CARTESIAN_POINT('Ctrl Pts',(-27.1117001758038,-71.66304607755,85.5928937542637));
#205258=CARTESIAN_POINT('Ctrl Pts',(-27.0893691484628,-72.6402332820879,
85.8118264664918));
#205259=CARTESIAN_POINT('Ctrl Pts',(-27.058137931487,-74.0484977405738,
85.9607580948701));
#205260=CARTESIAN_POINT('Ctrl Pts',(-27.0489528614825,-74.4660695562597,
85.9846445075633));
#205261=CARTESIAN_POINT('Ctrl Pts',(-27.0232634372046,-75.6221972224645,
85.9949554812449));
#205262=CARTESIAN_POINT('Ctrl Pts',(-27.0066641163935,-76.3595533194901,
85.938658020911));
#205263=CARTESIAN_POINT('Ctrl Pts',(-26.9732026303469,-77.8473159642464,
85.6965409593076));
#205264=CARTESIAN_POINT('Ctrl Pts',(-26.9564213215728,-78.5940315824319,
85.5058598959331));
#205265=CARTESIAN_POINT('Ctrl Pts',(-26.9181105876825,-80.2172155340921,
84.9340381390371));
#205266=CARTESIAN_POINT('Ctrl Pts',(-26.8967824074917,-81.0774988763897,
84.5201489840251));
#205267=CARTESIAN_POINT('Ctrl Pts',(-26.8665733823097,-82.2385163399785,
83.7952627014091));
#205268=CARTESIAN_POINT('Ctrl Pts',(-26.8574151612361,-82.581339692512,
83.5575747475936));
#205269=CARTESIAN_POINT('Ctrl Pts',(-26.8292781695803,-83.5889167148567,
82.784705495114));
#205270=CARTESIAN_POINT('Ctrl Pts',(-26.8100732895193,-84.2129557697868,
82.2002385404895));
#205271=CARTESIAN_POINT('Ctrl Pts',(-26.7720941103241,-85.3424817764598,
80.9118601477142));
#205272=CARTESIAN_POINT('Ctrl Pts',(-26.753303317099,-85.8440847764827,
80.2101232663707));
#205273=CARTESIAN_POINT('Ctrl Pts',(-26.7247441938428,-86.4803841279954,
79.1023740556961));
#205274=CARTESIAN_POINT('Ctrl Pts',(-26.7154039726759,-86.6705802017023,
78.7309685675455));
#205275=CARTESIAN_POINT('Ctrl Pts',(-26.687516654797,-87.1869621156996,
77.5905170151558));
#205276=CARTESIAN_POINT('Ctrl Pts',(-26.6692841116462,-87.4572622715524,
76.7985652204479));
#205277=CARTESIAN_POINT('Ctrl Pts',(-26.6330705952091,-87.8335432407178,
75.2105135517567));
#205278=CARTESIAN_POINT('Ctrl Pts',(-26.615132157317,-87.9456009001331,
74.4195782733135));
#205279=CARTESIAN_POINT('Ctrl Pts',(-26.5802741026907,-88.0223050939786,
72.8498560610542));
#205280=CARTESIAN_POINT('Ctrl Pts',(-26.5633772541898,-87.9909070205461,
72.0745076002212));
#205281=CARTESIAN_POINT('Ctrl Pts',(-26.5331691083482,-87.8155575262993,
70.7308942610897));
#205282=CARTESIAN_POINT('Ctrl Pts',(-26.5201397300098,-87.7019475361671,
70.1608885789199));
#205283=CARTESIAN_POINT('Ctrl Pts',(-26.4880993897788,-87.3265303784449,
68.7703861214209));
#205284=CARTESIAN_POINT('Ctrl Pts',(-26.469367816656,-87.0206583434366,
67.9646590272421));
#205285=CARTESIAN_POINT('Ctrl Pts',(-26.4279358786798,-86.1915521415113,
66.2993188834545));
#205286=CARTESIAN_POINT('Ctrl Pts',(-26.4055508421172,-85.6436717340647,
65.4580546557962));
#205287=CARTESIAN_POINT('Ctrl Pts',(-26.3742637420243,-84.7377897463188,
64.3662303866109));
#205288=CARTESIAN_POINT('Ctrl Pts',(-26.3650766230423,-84.4554618402258,
64.0575380091121));
#205289=CARTESIAN_POINT('Ctrl Pts',(-26.3391925499099,-83.6288559059582,
63.2369483463782));
#205290=CARTESIAN_POINT('Ctrl Pts',(-26.3224035255189,-83.0546221804428,
62.7575366580548));
#205291=CARTESIAN_POINT('Ctrl Pts',(-26.288744657427,-81.8110707131792,
61.8892383843992));
#205292=CARTESIAN_POINT('Ctrl Pts',(-26.2719453307364,-81.1418023689104,
61.5053708406699));
#205293=CARTESIAN_POINT('Ctrl Pts',(-26.2323686082621,-79.5281026168419,
60.761456111086));
#205294=CARTESIAN_POINT('Ctrl Pts',(-26.2098478145725,-78.5677958794463,
60.4475697757339));
#205295=CARTESIAN_POINT('Ctrl Pts',(-26.178419829599,-77.170969302484,60.1646211098846));
#205296=CARTESIAN_POINT('Ctrl Pts',(-26.1692271293691,-76.7572395020834,
60.1014120225384));
#205297=CARTESIAN_POINT('Ctrl Pts',(-26.142814409925,-75.5754964523061,
59.9788397979898));
#205298=CARTESIAN_POINT('Ctrl Pts',(-26.1255100904786,-74.8042631984752,
59.9675882242852));
#205299=CARTESIAN_POINT('Ctrl Pts',(-26.0893601842626,-73.1784717009032,
60.0884070018804));
#205300=CARTESIAN_POINT('Ctrl Pts',(-26.0705793196808,-72.3288174455748,
60.237215234787));
#205301=CARTESIAN_POINT('Ctrl Pts',(-26.042047382451,-71.099380616013,60.5808957099613));
#205302=CARTESIAN_POINT('Ctrl Pts',(-26.0327257399638,-70.704253010256,
60.7120943079282));
#205303=CARTESIAN_POINT('Ctrl Pts',(-26.0048113758553,-69.5357311055653,
61.1634258318586));
#205304=CARTESIAN_POINT('Ctrl Pts',(-25.9865326585622,-68.7862798016467,
61.5394572572545));
#205305=CARTESIAN_POINT('Ctrl Pts',(-25.9489134971732,-67.3502583099147,
62.4427544177539));
#205306=CARTESIAN_POINT('Ctrl Pts',(-25.929558754459,-66.6695701650831,
62.9717312372613));
#205307=CARTESIAN_POINT('Ctrl Pts',(-25.8912172492533,-65.414719019039,
64.1638760616071));
#205308=CARTESIAN_POINT('Ctrl Pts',(-25.8721731650173,-64.8451986270309,
64.8256499656624));
#205309=CARTESIAN_POINT('Ctrl Pts',(-25.8427037871473,-64.0902272375414,
65.9053665055431));
#205310=CARTESIAN_POINT('Ctrl Pts',(-25.8327088204804,-63.8533448154717,
66.2843000645008));
#205311=CARTESIAN_POINT('Ctrl Pts',(-25.8127813124671,-63.4181321071454,
67.0675432220405));
#205312=CARTESIAN_POINT('Ctrl Pts',(-25.8028630731624,-63.2203515073318,
67.4714727024354));
#205313=CARTESIAN_POINT('Ctrl Pts',(-25.7929565710457,-63.0438884777109,
67.8848324446381));
#205314=CARTESIAN_POINT('Ctrl Pts',(-25.7925315892805,-63.0438921656051,
67.8848238058572));
#205315=CARTESIAN_POINT('Ctrl Pts',(-25.7738172320668,-62.7100470282805,
68.6668451962005));
#205316=CARTESIAN_POINT('Ctrl Pts',(-25.7554910654483,-62.4537335522494,
69.4797282856584));
#205317=CARTESIAN_POINT('Ctrl Pts',(-25.7174585685912,-62.1044834842583,
71.1393471814885));
#205318=CARTESIAN_POINT('Ctrl Pts',(-25.6982654760424,-62.0114982552743,
71.9819134464724));
#205319=CARTESIAN_POINT('Ctrl Pts',(-25.6580815311061,-61.9889913307642,
73.7950592766215));
#205320=CARTESIAN_POINT('Ctrl Pts',(-25.6373707278172,-62.0850391643306,
74.7609040481865));
#205321=CARTESIAN_POINT('Ctrl Pts',(-25.6073298168377,-62.3662814718529,
76.0762223461048));
#205322=CARTESIAN_POINT('Ctrl Pts',(-25.5988027409165,-62.4612419119342,
76.4417162546856));
#205323=CARTESIAN_POINT('Ctrl Pts',(-25.5810816491096,-62.691769055563,
77.1929608534078));
#205324=CARTESIAN_POINT('Ctrl Pts',(-25.5719178118878,-62.8296852896929,
77.5768138836555));
#205325=CARTESIAN_POINT('Ctrl Pts',(-25.5628518781596,-62.9850802944281,
77.9529305295057));
#205326=CARTESIAN_POINT('Ctrl Pts',(-27.071820154481,-62.9850802944281,
77.9529305295057));
#205327=CARTESIAN_POINT('Ctrl Pts',(-27.0605085630959,-63.1833381622568,
78.4327920565107));
#205328=CARTESIAN_POINT('Ctrl Pts',(-27.049101708122,-63.4103735747692,
78.9008494225221));
#205329=CARTESIAN_POINT('Ctrl Pts',(-27.0197226292045,-64.0551482435365,
80.0489594352128));
#205330=CARTESIAN_POINT('Ctrl Pts',(-27.0015063464426,-64.5081422844583,
80.7060954678677));
#205331=CARTESIAN_POINT('Ctrl Pts',(-26.9591716827354,-65.7149938805126,
82.1524482732041));
#205332=CARTESIAN_POINT('Ctrl Pts',(-26.9361717899996,-66.5135494821474,
82.8965785261809));
#205333=CARTESIAN_POINT('Ctrl Pts',(-26.8941455562996,-68.0553710478556,
84.0086129137462));
#205334=CARTESIAN_POINT('Ctrl Pts',(-26.8756807982664,-68.7585955380911,
84.4216064754456));
#205335=CARTESIAN_POINT('Ctrl Pts',(-26.8189728575791,-71.0278336113285,
85.4821576745034));
#205336=CARTESIAN_POINT('Ctrl Pts',(-26.7836306163197,-72.6849640066519,
85.8923956538304));
#205337=CARTESIAN_POINT('Ctrl Pts',(-26.7312779313272,-75.0002087808532,
86.0039922299509));
#205338=CARTESIAN_POINT('Ctrl Pts',(-26.7169492234306,-75.6276625140699,
85.9888486313766));
#205339=CARTESIAN_POINT('Ctrl Pts',(-26.6742994734323,-77.5315740273115,
85.8046950514129));
#205340=CARTESIAN_POINT('Ctrl Pts',(-26.6471833103362,-78.7861514616839,
85.491643868765));
#205341=CARTESIAN_POINT('Ctrl Pts',(-26.6020301352276,-80.6440099035058,
84.7222013166686));
#205342=CARTESIAN_POINT('Ctrl Pts',(-26.5854317026867,-81.2893519808264,
84.3893059529311));
#205343=CARTESIAN_POINT('Ctrl Pts',(-26.5450219156057,-82.8187606775407,
83.4308013914143));
#205344=CARTESIAN_POINT('Ctrl Pts',(-26.5221896286254,-83.6589081773433,
82.745418781419));
#205345=CARTESIAN_POINT('Ctrl Pts',(-26.4780446566162,-85.0340590756997,
81.3044740726327));
#205346=CARTESIAN_POINT('Ctrl Pts',(-26.4572014070912,-85.5923854343911,
80.580504548093));
#205347=CARTESIAN_POINT('Ctrl Pts',(-26.4036318025543,-86.8409453687443,
78.5523955472661));
#205348=CARTESIAN_POINT('Ctrl Pts',(-26.3728346457446,-87.3936828613449,
77.1790237108958));
#205349=CARTESIAN_POINT('Ctrl Pts',(-26.3244976065549,-87.8482483293957,
75.0816632665241));
#205350=CARTESIAN_POINT('Ctrl Pts',(-26.309023679321,-87.939693929986,74.4106851658523));
#205351=CARTESIAN_POINT('Ctrl Pts',(-26.2641235957008,-88.0551063728715,
72.4048400663272));
#205352=CARTESIAN_POINT('Ctrl Pts',(-26.236068088882,-87.9265379141445,
71.0701429435457));
#205353=CARTESIAN_POINT('Ctrl Pts',(-26.1966699289298,-87.4936517846722,
69.3715812651332));
#205354=CARTESIAN_POINT('Ctrl Pts',(-26.1871415785317,-87.3703257424435,
68.9700224056217));
#205355=CARTESIAN_POINT('Ctrl Pts',(-26.1506331525314,-86.8235764234751,
67.4553166560676));
#205356=CARTESIAN_POINT('Ctrl Pts',(-26.1251170343784,-86.2674471834665,
66.3963153222307));
#205357=CARTESIAN_POINT('Ctrl Pts',(-26.0806649581548,-85.0904635869507,
64.7501647272766));
#205358=CARTESIAN_POINT('Ctrl Pts',(-26.0619069099169,-84.5419049123381,
64.1206280516891));
#205359=CARTESIAN_POINT('Ctrl Pts',(-26.0155474042753,-83.0573098974036,
62.7152958766662));
#205360=CARTESIAN_POINT('Ctrl Pts',(-25.9895183091989,-82.0656527705764,
62.0096573407316));
#205361=CARTESIAN_POINT('Ctrl Pts',(-25.9446017362156,-80.2497908463196,
61.0667794260827));
#205362=CARTESIAN_POINT('Ctrl Pts',(-25.9258205977842,-79.4735168696853,
60.7543225526591));
#205363=CARTESIAN_POINT('Ctrl Pts',(-25.8792531495457,-77.5038511100906,
60.1742348887088));
#205364=CARTESIAN_POINT('Ctrl Pts',(-25.8530429820652,-76.2924140455704,
59.99603259637));
#205365=CARTESIAN_POINT('Ctrl Pts',(-25.7978641992104,-73.7784208884928,
59.9817283532629));
#205366=CARTESIAN_POINT('Ctrl Pts',(-25.7679576827344,-72.4890563234385,
60.1680641200768));
#205367=CARTESIAN_POINT('Ctrl Pts',(-25.7252345790055,-70.6399547469968,
60.7253599424343));
#205368=CARTESIAN_POINT('Ctrl Pts',(-25.7115677709163,-70.0455440165122,
60.9532121513621));
#205369=CARTESIAN_POINT('Ctrl Pts',(-25.6608585552909,-67.943733948015,
61.9410879475899));
#205370=CARTESIAN_POINT('Ctrl Pts',(-25.6219008261576,-66.5714049687478,
62.9487898662649));
#205371=CARTESIAN_POINT('Ctrl Pts',(-25.5674029111497,-64.8778510748112,
64.7908806333424));
#205372=CARTESIAN_POINT('Ctrl Pts',(-25.549760377948,-64.3835663112684,
65.441931124519));
#205373=CARTESIAN_POINT('Ctrl Pts',(-25.5071780938452,-63.377353860841,
67.0636464881761));
#205374=CARTESIAN_POINT('Ctrl Pts',(-25.4819488655821,-62.9205537432864,
68.0612702470938));
#205375=CARTESIAN_POINT('Ctrl Pts',(-25.4375428607864,-62.3153757048581,
69.9939712112621));
#205376=CARTESIAN_POINT('Ctrl Pts',(-25.417562809417,-62.1332992362535,
70.9110885375044));
#205377=CARTESIAN_POINT('Ctrl Pts',(-25.3726675196767,-61.9551318000054,
72.9188124367098));
#205378=CARTESIAN_POINT('Ctrl Pts',(-25.3476385525834,-61.9946232894889,
74.005599743831));
#205379=CARTESIAN_POINT('Ctrl Pts',(-25.3071797422959,-62.289856269085,
75.8216872342338));
#205380=CARTESIAN_POINT('Ctrl Pts',(-25.2909561985297,-62.4762348922606,
76.556496056355));
#205381=CARTESIAN_POINT('Ctrl Pts',(-25.268934758749,-62.8056646343085,
77.5008148037921));
#205382=CARTESIAN_POINT('Ctrl Pts',(-25.2635448812278,-62.8922473331595,
77.7282384805162));
#205383=CARTESIAN_POINT('Ctrl Pts',(-25.2581222247367,-62.9850802944281,
77.9529305295057));
#205384=CARTESIAN_POINT('Origin',(-21.6548258024609,-75.,72.98888938658));
#205385=CARTESIAN_POINT('',(-29.1914736244731,-62.9850802944281,77.9529305295057));
#205386=CARTESIAN_POINT('',(-28.8854250924612,-62.9850802944281,77.9529305295057));
#205387=CARTESIAN_POINT('',(-21.6548258024609,-62.9850802944281,77.9529305295057));
#205388=CARTESIAN_POINT('Ctrl Pts',(-29.1914736244731,-62.9850802944281,
77.9529305295057));
#205389=CARTESIAN_POINT('Ctrl Pts',(-29.1755621721884,-63.2591578354856,
78.6163052989917));
#205390=CARTESIAN_POINT('Ctrl Pts',(-29.1594040788803,-63.5877981516252,
79.2560679492924));
#205391=CARTESIAN_POINT('Ctrl Pts',(-29.1263368716955,-64.3743472329357,
80.5179243315183));
#205392=CARTESIAN_POINT('Ctrl Pts',(-29.1095424566542,-64.8380145192152,
81.1328999266125));
#205393=CARTESIAN_POINT('Ctrl Pts',(-29.0734221104526,-65.9292423739749,
82.3408723417191));
#205394=CARTESIAN_POINT('Ctrl Pts',(-29.054089877859,-66.5669919732695,
82.919781383801));
#205395=CARTESIAN_POINT('Ctrl Pts',(-29.0258111347309,-67.5927591563554,
83.6803490747793));
#205396=CARTESIAN_POINT('Ctrl Pts',(-29.0166214060534,-67.9401399587385,
83.9128494579239));
#205397=CARTESIAN_POINT('Ctrl Pts',(-28.9884263336115,-69.0353829579731,
84.5717936722388));
#205398=CARTESIAN_POINT('Ctrl Pts',(-28.9690997076129,-69.8148721486558,
84.9410760656296));
#205399=CARTESIAN_POINT('Ctrl Pts',(-28.9323737912149,-71.3688686424714,
85.4964360550529));
#205400=CARTESIAN_POINT('Ctrl Pts',(-28.9151159570361,-72.1353086370993,
85.6939031444884));
#205401=CARTESIAN_POINT('Ctrl Pts',(-28.880488831689,-73.6761769729656,
85.9442866240956));
#205402=CARTESIAN_POINT('Ctrl Pts',(-28.8631309851456,-74.4469406872649,
85.9999982835116));
#205403=CARTESIAN_POINT('Ctrl Pts',(-28.8300150987229,-75.9384665632339,
85.9749733885017));
#205404=CARTESIAN_POINT('Ctrl Pts',(-28.8142737633991,-76.6565950375665,
85.9030205174585));
#205405=CARTESIAN_POINT('Ctrl Pts',(-28.7822369910288,-78.0750298881094,
85.6405895141111));
#205406=CARTESIAN_POINT('Ctrl Pts',(-28.7659970656264,-78.7728339413504,
85.4503120997551));
#205407=CARTESIAN_POINT('Ctrl Pts',(-28.7328261718324,-80.175820507993,
84.9390213630989));
#205408=CARTESIAN_POINT('Ctrl Pts',(-28.7159965259154,-80.8754814233276,
84.6110012888045));
#205409=CARTESIAN_POINT('Ctrl Pts',(-28.6812698174062,-82.2249190080084,
83.8251807021196));
#205410=CARTESIAN_POINT('Ctrl Pts',(-28.6635084526963,-82.8702201885422,
83.3659944822798));
#205411=CARTESIAN_POINT('Ctrl Pts',(-28.626929441276,-84.1225480427867,
82.2904716196668));
#205412=CARTESIAN_POINT('Ctrl Pts',(-28.6081295274468,-84.7180178052968,
81.6664721582494));
#205413=CARTESIAN_POINT('Ctrl Pts',(-28.5795486684124,-85.5045511626666,
80.6588937726708));
#205414=CARTESIAN_POINT('Ctrl Pts',(-28.570193195534,-85.7456159824158,
80.3173476616895));
#205415=CARTESIAN_POINT('Ctrl Pts',(-28.5417559073132,-86.4308791313648,
79.2397502921107));
#205416=CARTESIAN_POINT('Ctrl Pts',(-28.523020235589,-86.8189264968287,
78.4707894383435));
#205417=CARTESIAN_POINT('Ctrl Pts',(-28.4867789070654,-87.4058188311497,
76.9499500513124));
#205418=CARTESIAN_POINT('Ctrl Pts',(-28.4694491703824,-87.6188456655288,
76.2074429441466));
#205419=CARTESIAN_POINT('Ctrl Pts',(-28.4332753495974,-87.9277554198034,
74.6055389112504));
#205420=CARTESIAN_POINT('Ctrl Pts',(-28.4144934450725,-88.0063975754321,
73.7465415249287));
#205421=CARTESIAN_POINT('Ctrl Pts',(-28.3859585213444,-87.9963025101264,
72.4698993914055));
#205422=CARTESIAN_POINT('Ctrl Pts',(-28.376634771575,-87.9730259155091,
72.0541011215623));
#205423=CARTESIAN_POINT('Ctrl Pts',(-28.3487236059692,-87.8430715098968,
70.8082898733804));
#205424=CARTESIAN_POINT('Ctrl Pts',(-28.3304501425691,-87.6762258924339,
69.986758647326));
#205425=CARTESIAN_POINT('Ctrl Pts',(-28.2930328738841,-87.1827848282919,
68.3732910096947));
#205426=CARTESIAN_POINT('Ctrl Pts',(-28.2738814873312,-86.8546556479647,
67.5860066595706));
#205427=CARTESIAN_POINT('Ctrl Pts',(-28.2359663672673,-86.0447706375438,
66.0785123439422));
#205428=CARTESIAN_POINT('Ctrl Pts',(-28.2171633117146,-85.5633401429903,
65.3628739021637));
#205429=CARTESIAN_POINT('Ctrl Pts',(-28.1885755944839,-84.7481969832629,
64.3779990500524));
#205430=CARTESIAN_POINT('Ctrl Pts',(-28.1792151542129,-84.4662578931964,
64.0689824667347));
#205431=CARTESIAN_POINT('Ctrl Pts',(-28.1507740214326,-83.560831951342,
63.1679663154694));
#205432=CARTESIAN_POINT('Ctrl Pts',(-28.1320394445061,-82.8931483779347,
62.623727785215));
#205433=CARTESIAN_POINT('Ctrl Pts',(-28.0954542648856,-81.5213277445394,
61.715468453194));
#205434=CARTESIAN_POINT('Ctrl Pts',(-28.0777905124525,-80.8279836820453,
61.3419003843233));
#205435=CARTESIAN_POINT('Ctrl Pts',(-28.0413029644768,-79.3138385090679,
60.6953481352096));
#205436=CARTESIAN_POINT('Ctrl Pts',(-28.0225071271223,-78.4909283062354,
60.4368466474481));
#205437=CARTESIAN_POINT('Ctrl Pts',(-27.993935632166,-77.2398238489032,
60.1764943159538));
#205438=CARTESIAN_POINT('Ctrl Pts',(-27.9845868043934,-76.8272524890396,
60.1111788856647));
#205439=CARTESIAN_POINT('Ctrl Pts',(-27.9567139655793,-75.5831669532874,
59.9752229935156));
#205440=CARTESIAN_POINT('Ctrl Pts',(-27.9385046600024,-74.7472853763196,
59.964615039217));
#205441=CARTESIAN_POINT('Ctrl Pts',(-27.9029475108486,-73.1509483478164,
60.0981690246326));
#205442=CARTESIAN_POINT('Ctrl Pts',(-27.885670168254,-72.3929009548486,
60.2298649264436));
#205443=CARTESIAN_POINT('Ctrl Pts',(-27.8515433038747,-70.9070939213903,
60.6260123463768));
#205444=CARTESIAN_POINT('Ctrl Pts',(-27.8347485680442,-70.1823530868346,
60.8900098978475));
#205445=CARTESIAN_POINT('Ctrl Pts',(-27.7953816908557,-68.5816472958152,
61.639862689273));
#205446=CARTESIAN_POINT('Ctrl Pts',(-27.7730563827175,-67.7297725838768,
62.1657900868321));
#205447=CARTESIAN_POINT('Ctrl Pts',(-27.7418310773711,-66.6183415033926,
63.0429088602213));
#205448=CARTESIAN_POINT('Ctrl Pts',(-27.7326462182551,-66.3028913888067,
63.3175384920493));
#205449=CARTESIAN_POINT('Ctrl Pts',(-27.7069767692208,-65.4691242607782,
64.1172488383875));
#205450=CARTESIAN_POINT('Ctrl Pts',(-27.6903969088421,-64.9814065792122,
64.6719553088264));
#205451=CARTESIAN_POINT('Ctrl Pts',(-27.6569542018304,-64.0863625099057,
65.8836730522086));
#205452=CARTESIAN_POINT('Ctrl Pts',(-27.6401732640537,-63.685186410512,
66.5416750410925));
#205453=CARTESIAN_POINT('Ctrl Pts',(-27.6019784637782,-62.9252502354484,
68.0800545492526));
#205454=CARTESIAN_POINT('Ctrl Pts',(-27.5807611369532,-62.5999289538605,
68.9721117127493));
#205455=CARTESIAN_POINT('Ctrl Pts',(-27.5506635777758,-62.2750570347021,
70.2963863309321));
#205456=CARTESIAN_POINT('Ctrl Pts',(-27.5415074160872,-62.1952730413356,
70.7057528316857));
#205457=CARTESIAN_POINT('Ctrl Pts',(-27.5132372864691,-62.0116317256353,
71.968680244846));
#205458=CARTESIAN_POINT('Ctrl Pts',(-27.493885655565,-61.9726032158218,
72.8292869784305));
#205459=CARTESIAN_POINT('Ctrl Pts',(-27.4557636926057,-62.0650170574753,
74.5466477551924));
#205460=CARTESIAN_POINT('Ctrl Pts',(-27.4369728765414,-62.196445098373,
75.399153925258));
#205461=CARTESIAN_POINT('Ctrl Pts',(-27.4084136951864,-62.5151810677153,
76.6362462977439));
#205462=CARTESIAN_POINT('Ctrl Pts',(-27.3990734339573,-62.6386037251102,
77.0348502593141));
#205463=CARTESIAN_POINT('Ctrl Pts',(-27.3855913578634,-62.8452187583533,
77.6037255106876));
#205464=CARTESIAN_POINT('Ctrl Pts',(-27.3814112768546,-62.9132742983489,
77.7791319544275));
#205465=CARTESIAN_POINT('Ctrl Pts',(-27.3772428998354,-62.9850802944281,
77.9529305295057));
#205466=CARTESIAN_POINT('',(-27.3009674773133,-63.0439273761962,67.8848561928422));
#205467=CARTESIAN_POINT('Ctrl Pts',(-27.3016104665866,-63.0438801073788,
67.8848520519528));
#205468=CARTESIAN_POINT('Ctrl Pts',(-27.2822043952599,-62.7048107611236,
68.6791161785564));
#205469=CARTESIAN_POINT('Ctrl Pts',(-27.2623604194506,-62.4457280137918,
69.5051981159832));
#205470=CARTESIAN_POINT('Ctrl Pts',(-27.2247684323744,-62.0997039577012,
71.1748968405862));
#205471=CARTESIAN_POINT('Ctrl Pts',(-27.2067907395125,-62.0093496555475,
72.0135779289911));
#205472=CARTESIAN_POINT('Ctrl Pts',(-27.1756917833625,-61.9948459983377,
73.4227544982765));
#205473=CARTESIAN_POINT('Ctrl Pts',(-27.1629591529323,-62.0261927256133,
73.9901809827204));
#205474=CARTESIAN_POINT('Ctrl Pts',(-27.1372091243939,-62.1630295671768,
75.1186928323105));
#205475=CARTESIAN_POINT('Ctrl Pts',(-27.1242209431371,-62.2685576332493,
75.6785454171776));
#205476=CARTESIAN_POINT('Ctrl Pts',(-27.0980726651425,-62.5617205545539,
76.8174027048613));
#205477=CARTESIAN_POINT('Ctrl Pts',(-27.0850145343578,-62.7538228583481,
77.3931971498224));
#205478=CARTESIAN_POINT('Ctrl Pts',(-27.071820154481,-62.9850802944281,
77.9529305295057));
#205479=CARTESIAN_POINT('Ctrl Pts',(-28.8854250924612,-62.9850802944281,
77.9529305295057));
#205480=CARTESIAN_POINT('Ctrl Pts',(-28.8824655793347,-63.0358772790107,
78.0758790856261));
#205481=CARTESIAN_POINT('Ctrl Pts',(-28.8795000358553,-63.0885757045039,
78.1980824181724));
#205482=CARTESIAN_POINT('Ctrl Pts',(-28.8672392884279,-63.3138460309727,
78.6991499770645));
#205483=CARTESIAN_POINT('Ctrl Pts',(-28.8579067524138,-63.502667170325,
79.0703865634795));
#205484=CARTESIAN_POINT('Ctrl Pts',(-28.8331156173381,-64.0532943620823,
80.0353275583397));
#205485=CARTESIAN_POINT('Ctrl Pts',(-28.8179202547627,-64.4454316197721,
80.6101584291343));
#205486=CARTESIAN_POINT('Ctrl Pts',(-28.7840050379732,-65.4080639597539,
81.8035269703564));
#205487=CARTESIAN_POINT('Ctrl Pts',(-28.7651855741755,-65.996414212715,
82.4036915784779));
#205488=CARTESIAN_POINT('Ctrl Pts',(-28.7276143167663,-67.2887154577256,
83.4892378536429));
#205489=CARTESIAN_POINT('Ctrl Pts',(-28.7091060250991,-67.9909505633124,
83.9704401572734));
#205490=CARTESIAN_POINT('Ctrl Pts',(-28.6710714995552,-69.489034416249,
84.7943820743572));
#205491=CARTESIAN_POINT('Ctrl Pts',(-28.6517323799731,-70.2823015206987,
85.1331773765378));
#205492=CARTESIAN_POINT('Ctrl Pts',(-28.6235498509551,-71.5008811970346,
85.5160569308502));
#205493=CARTESIAN_POINT('Ctrl Pts',(-28.6143826938631,-71.9043369166701,
85.6218078543965));
#205494=CARTESIAN_POINT('Ctrl Pts',(-28.5866663319979,-73.1293523489743,
85.880680528793));
#205495=CARTESIAN_POINT('Ctrl Pts',(-28.5678985716926,-73.9612676513088,
85.974212703464));
#205496=CARTESIAN_POINT('Ctrl Pts',(-28.531333297673,-75.605680191057,85.9999722142122));
#205497=CARTESIAN_POINT('Ctrl Pts',(-28.5136766214303,-76.4143968440435,
85.9370403358745));
#205498=CARTESIAN_POINT('Ctrl Pts',(-28.4765401100638,-78.059918010105,
85.6529057517265));
#205499=CARTESIAN_POINT('Ctrl Pts',(-28.4571926682296,-78.8912150091837,
85.422668558253));
#205500=CARTESIAN_POINT('Ctrl Pts',(-28.4290213078015,-80.0816420114004,
84.9617761961946));
#205501=CARTESIAN_POINT('Ctrl Pts',(-28.4198731218469,-80.462199939638,
84.793018997335));
#205502=CARTESIAN_POINT('Ctrl Pts',(-28.3921519553204,-81.5816459408153,
84.2308579975198));
#205503=CARTESIAN_POINT('Ctrl Pts',(-28.3733616829992,-82.2912915357417,
83.7841186163781));
#205504=CARTESIAN_POINT('Ctrl Pts',(-28.3356090360205,-83.6337639378527,
82.7458663572929));
#205505=CARTESIAN_POINT('Ctrl Pts',(-28.316851665917,-84.2605066764315,
82.1531406746028));
#205506=CARTESIAN_POINT('Ctrl Pts',(-28.2785424006694,-85.3875212687281,
80.8527031060992));
#205507=CARTESIAN_POINT('Ctrl Pts',(-28.2592282455856,-85.8850413062418,
80.1482225450452));
#205508=CARTESIAN_POINT('Ctrl Pts',(-28.2310242805193,-86.5156813028842,
79.0357238888119));
#205509=CARTESIAN_POINT('Ctrl Pts',(-28.2218167549783,-86.7043522748128,
78.6619186330587));
#205510=CARTESIAN_POINT('Ctrl Pts',(-28.1935087511738,-87.224423088215,
77.494667323832));
#205511=CARTESIAN_POINT('Ctrl Pts',(-28.174165356958,-87.4954779101746,
76.6769212038579));
#205512=CARTESIAN_POINT('Ctrl Pts',(-28.1354288842283,-87.8783888984185,
74.9725128564299));
#205513=CARTESIAN_POINT('Ctrl Pts',(-28.1160379031832,-87.9837419388559,
74.0889426736047));
#205514=CARTESIAN_POINT('Ctrl Pts',(-28.0780343535472,-88.0116076500931,
72.3857529019448));
#205515=CARTESIAN_POINT('Ctrl Pts',(-28.0597797126823,-87.9481231107597,
71.5705006207187));
#205516=CARTESIAN_POINT('Ctrl Pts',(-28.0233789710146,-87.665858585689,
69.9436118868057));
#205517=CARTESIAN_POINT('Ctrl Pts',(-28.004920380141,-87.4440862150033,
69.1363059541179));
#205518=CARTESIAN_POINT('Ctrl Pts',(-27.9768517933053,-86.996931562581,
67.9639966602238));
#205519=CARTESIAN_POINT('Ctrl Pts',(-27.9674592017099,-86.8285779729279,
67.5795770417272));
#205520=CARTESIAN_POINT('Ctrl Pts',(-27.9363387786485,-86.2034007776042,
66.3214313900472));
#205521=CARTESIAN_POINT('Ctrl Pts',(-27.9147711115775,-85.6659305417049,
65.4916152787042));
#205522=CARTESIAN_POINT('Ctrl Pts',(-27.8833998203224,-84.7745594953122,
64.4079550040323));
#205523=CARTESIAN_POINT('Ctrl Pts',(-27.8740344559414,-84.4938395378865,
64.0983629976914));
#205524=CARTESIAN_POINT('Ctrl Pts',(-27.8480890864951,-83.6686900736822,
63.2720783091558));
#205525=CARTESIAN_POINT('Ctrl Pts',(-27.8317104287565,-83.0937338446361,
62.7881989913403));
#205526=CARTESIAN_POINT('Ctrl Pts',(-27.7979650810881,-81.8512099718502,
61.9140300097616));
#205527=CARTESIAN_POINT('Ctrl Pts',(-27.7806504762213,-81.1841122769408,
61.5281589163973));
#205528=CARTESIAN_POINT('Ctrl Pts',(-27.7428609581753,-79.6382848471565,
60.8084786023036));
#205529=CARTESIAN_POINT('Ctrl Pts',(-27.7223959097572,-78.7495511502333,
60.5062226702327));
#205530=CARTESIAN_POINT('Ctrl Pts',(-27.6921817138872,-77.429474847673,
60.211125373953));
#205531=CARTESIAN_POINT('Ctrl Pts',(-27.6828380244843,-77.0187214407476,
60.1398285331527));
#205532=CARTESIAN_POINT('Ctrl Pts',(-27.6544110533982,-75.7525834549773,
59.9822785596287));
#205533=CARTESIAN_POINT('Ctrl Pts',(-27.6356910284017,-74.8914904492901,
59.9609756913596));
#205534=CARTESIAN_POINT('Ctrl Pts',(-27.5974446215772,-73.1765211424777,
60.0886827820958));
#205535=CARTESIAN_POINT('Ctrl Pts',(-27.5780981620778,-72.3268867517458,
60.2376195978667));
#205536=CARTESIAN_POINT('Ctrl Pts',(-27.5499260062608,-71.0974578197744,
60.581498901876));
#205537=CARTESIAN_POINT('Ctrl Pts',(-27.540775909522,-70.7023113279648,
60.712772486862));
#205538=CARTESIAN_POINT('Ctrl Pts',(-27.5130551559875,-69.533893804592,
61.1642803011753));
#205539=CARTESIAN_POINT('Ctrl Pts',(-27.4942668993613,-68.7845696208448,
61.5403913624682));
#205540=CARTESIAN_POINT('Ctrl Pts',(-27.4565944832196,-67.3511627671109,
62.4423309471043));
#205541=CARTESIAN_POINT('Ctrl Pts',(-27.4379095124625,-66.672649402451,
62.9694161330161));
#205542=CARTESIAN_POINT('Ctrl Pts',(-27.3994173835239,-65.4184273779293,
64.1597368892016));
#205543=CARTESIAN_POINT('Ctrl Pts',(-27.3798457176042,-64.8478964836777,
64.822171974088));
#205544=CARTESIAN_POINT('Ctrl Pts',(-27.3507575415468,-64.0916824146765,
65.9030914571655));
#205545=CARTESIAN_POINT('Ctrl Pts',(-27.3409191317284,-63.8544409354465,
66.2824419366119));
#205546=CARTESIAN_POINT('Ctrl Pts',(-27.3210268214252,-63.4186041746793,
67.0665787968306));
#205547=CARTESIAN_POINT('Ctrl Pts',(-27.3109849659766,-63.2205605326239,
67.4709825907912));
#205548=CARTESIAN_POINT('Ctrl Pts',(-27.3009162452285,-63.0438863592108,
67.8848374071685));
#205549=CARTESIAN_POINT('Origin',(-21.6548258024609,-75.,72.98888938658));
#205550=CARTESIAN_POINT('',(-31.0052564152503,-62.9850802944281,77.9529305295057));
#205551=CARTESIAN_POINT('',(-30.6991941617974,-62.9850802944281,77.9529305295057));
#205552=CARTESIAN_POINT('',(-21.6548258024609,-62.9850802944281,77.9529305295057));
#205553=CARTESIAN_POINT('Ctrl Pts',(-31.0052564152503,-62.9850802944281,
77.9529305295057));
#205554=CARTESIAN_POINT('Ctrl Pts',(-30.998890721168,-63.0941305563431,
78.2168747844095));
#205555=CARTESIAN_POINT('Ctrl Pts',(-30.992546634712,-63.211905957649,78.4772925112609));
#205556=CARTESIAN_POINT('Ctrl Pts',(-30.977020603939,-63.5219807092366,
79.1067278389773));
#205557=CARTESIAN_POINT('Ctrl Pts',(-30.9678790268683,-63.7235073326383,
79.470678282968));
#205558=CARTESIAN_POINT('Ctrl Pts',(-30.9397116448984,-64.3945669932255,
80.5562669748228));
#205559=CARTESIAN_POINT('Ctrl Pts',(-30.9203616937345,-64.9185583979383,
81.2414609983222));
#205560=CARTESIAN_POINT('Ctrl Pts',(-30.8821217527453,-66.0933516303725,
82.4972986267386));
#205561=CARTESIAN_POINT('Ctrl Pts',(-30.8634032798322,-66.7410769815901,
83.0650205822738));
#205562=CARTESIAN_POINT('Ctrl Pts',(-30.8349730262052,-67.7789653735092,
83.8069395387207));
#205563=CARTESIAN_POINT('Ctrl Pts',(-30.8256308472951,-68.1293227337512,
84.0327720483039));
#205564=CARTESIAN_POINT('Ctrl Pts',(-30.7955149464664,-69.2964528224528,
84.7080097513539));
#205565=CARTESIAN_POINT('Ctrl Pts',(-30.7751434413671,-70.1508200863168,
85.0865617937747));
#205566=CARTESIAN_POINT('Ctrl Pts',(-30.7452056164092,-71.4373644781035,
85.4982138897057));
#205567=CARTESIAN_POINT('Ctrl Pts',(-30.7358184244919,-71.8423845949013,
85.606537092857));
#205568=CARTESIAN_POINT('Ctrl Pts',(-30.7077965975312,-73.0667863961338,
85.8713481494891));
#205569=CARTESIAN_POINT('Ctrl Pts',(-30.6893835088621,-73.8967163923041,
85.9687904354329));
#205570=CARTESIAN_POINT('Ctrl Pts',(-30.6530238437094,-75.5455739484342,
86.0030124810472));
#205571=CARTESIAN_POINT('Ctrl Pts',(-30.6347672198482,-76.3606887553969,
85.9431769171672));
#205572=CARTESIAN_POINT('Ctrl Pts',(-30.5969613111317,-78.0319612450622,
85.6609303910857));
#205573=CARTESIAN_POINT('Ctrl Pts',(-30.5777484996156,-78.8820214190536,
85.4268680252424));
#205574=CARTESIAN_POINT('Ctrl Pts',(-30.5391876937375,-80.5030966674773,
84.7979716319442));
#205575=CARTESIAN_POINT('Ctrl Pts',(-30.5198459968039,-81.2714860176536,
84.4084764121768));
#205576=CARTESIAN_POINT('Ctrl Pts',(-30.4915427153229,-82.3484255275656,
83.7208822183712));
#205577=CARTESIAN_POINT('Ctrl Pts',(-30.4823380508623,-82.6899721208454,
83.4788539719696));
#205578=CARTESIAN_POINT('Ctrl Pts',(-30.4541354293864,-83.6964098417668,
82.6900575269572));
#205579=CARTESIAN_POINT('Ctrl Pts',(-30.4348190771385,-84.3192090680501,
82.0934233462604));
#205580=CARTESIAN_POINT('Ctrl Pts',(-30.3979038826536,-85.3972083610225,
80.8333015749217));
#205581=CARTESIAN_POINT('Ctrl Pts',(-30.3804678067385,-85.8589996796079,
80.1804721619447));
#205582=CARTESIAN_POINT('Ctrl Pts',(-30.3437108636977,-86.6877136293555,
78.7452595555407));
#205583=CARTESIAN_POINT('Ctrl Pts',(-30.3243708426616,-87.042570297055,
77.9603033557304));
#205584=CARTESIAN_POINT('Ctrl Pts',(-30.2960721159481,-87.451123536123,
76.7498013011091));
#205585=CARTESIAN_POINT('Ctrl Pts',(-30.2868702150667,-87.5656716688902,
76.3472865609622));
#205586=CARTESIAN_POINT('Ctrl Pts',(-30.2586689271407,-87.8559252135777,
75.1020439280308));
#205587=CARTESIAN_POINT('Ctrl Pts',(-30.2393505283487,-87.9675689660564,
74.2468159420369));
#205588=CARTESIAN_POINT('Ctrl Pts',(-30.2024711015591,-88.0182879167508,
72.5908060001859));
#205589=CARTESIAN_POINT('Ctrl Pts',(-30.1850687819595,-87.9694642594319,
71.7942011149537));
#205590=CARTESIAN_POINT('Ctrl Pts',(-30.1483453184102,-87.7170528784014,
70.1578113597426));
#205591=CARTESIAN_POINT('Ctrl Pts',(-30.129005666849,-87.5021665916542,
69.3236095689898));
#205592=CARTESIAN_POINT('Ctrl Pts',(-30.0976361792611,-87.0149633074977,
67.9938113137064));
#205593=CARTESIAN_POINT('Ctrl Pts',(-30.0854255918818,-86.7899758709906,
67.4837449317751));
#205594=CARTESIAN_POINT('Ctrl Pts',(-30.0559991048539,-86.176409896406,
66.3042153825508));
#205595=CARTESIAN_POINT('Ctrl Pts',(-30.038604703564,-85.759443167482,65.6519020193313));
#205596=CARTESIAN_POINT('Ctrl Pts',(-30.0033441253496,-84.789625849535,
64.3967389026165));
#205597=CARTESIAN_POINT('Ctrl Pts',(-29.9856049016184,-84.2328945423459,
63.8010997569562));
#205598=CARTESIAN_POINT('Ctrl Pts',(-29.9582198007299,-83.3120931500439,
62.9847381498667));
#205599=CARTESIAN_POINT('Ctrl Pts',(-29.9488670351272,-82.9868916860702,
62.7232430077088));
#205600=CARTESIAN_POINT('Ctrl Pts',(-29.9181246703679,-81.8746058136736,
61.9137490513676));
#205601=CARTESIAN_POINT('Ctrl Pts',(-29.8971567085003,-81.0395098635633,
61.4371254331555));
#205602=CARTESIAN_POINT('Ctrl Pts',(-29.8568706494704,-79.3706319919682,
60.7154828891975));
#205603=CARTESIAN_POINT('Ctrl Pts',(-29.837515411314,-78.5497294698801,
60.4534055255968));
#205604=CARTESIAN_POINT('Ctrl Pts',(-29.8057525708868,-77.1480165547809,
60.1547552842987));
#205605=CARTESIAN_POINT('Ctrl Pts',(-29.7931778075746,-76.5797519590921,
60.0724906885349));
#205606=CARTESIAN_POINT('Ctrl Pts',(-29.7633617608987,-75.2363492402821,
59.9680193058401));
#205607=CARTESIAN_POINT('Ctrl Pts',(-29.7459400975722,-74.4609644233192,
59.9770349905027));
#205608=CARTESIAN_POINT('Ctrl Pts',(-29.7105146841467,-72.8756579113476,
60.1374783268624));
#205609=CARTESIAN_POINT('Ctrl Pts',(-29.6926466581456,-72.0699435804465,
60.2969092162341));
#205610=CARTESIAN_POINT('Ctrl Pts',(-29.6557636623742,-70.4817919903966,
60.770556621236));
#205611=CARTESIAN_POINT('Ctrl Pts',(-29.6369550883942,-69.7039845516747,
61.0870368054686));
#205612=CARTESIAN_POINT('Ctrl Pts',(-29.6028427678378,-68.3384995671798,
61.8031764171198));
#205613=CARTESIAN_POINT('Ctrl Pts',(-29.5874452410841,-67.7425489572604,
62.1803202522952));
#205614=CARTESIAN_POINT('Ctrl Pts',(-29.5624436415863,-66.8475595708902,
62.8542470383659));
#205615=CARTESIAN_POINT('Ctrl Pts',(-29.5531115347342,-66.5272597426852,
63.1204582288388));
#205616=CARTESIAN_POINT('Ctrl Pts',(-29.5237793391725,-65.5579295318565,
64.0081358404112));
#205617=CARTESIAN_POINT('Ctrl Pts',(-29.5041537322335,-64.9602157775129,
64.6817025881481));
#205618=CARTESIAN_POINT('Ctrl Pts',(-29.4651861012681,-63.9357819911559,
66.1098130782895));
#205619=CARTESIAN_POINT('Ctrl Pts',(-29.4458405951834,-63.5053245953175,
66.856104093393));
#205620=CARTESIAN_POINT('Ctrl Pts',(-29.4175265459778,-62.9794073986883,
68.0209322914322));
#205621=CARTESIAN_POINT('Ctrl Pts',(-29.4083153639602,-62.8256744199076,
68.4105664141887));
#205622=CARTESIAN_POINT('Ctrl Pts',(-29.3801097432522,-62.4142571445577,
69.6215155846038));
#205623=CARTESIAN_POINT('Ctrl Pts',(-29.3607985206994,-62.2190493172461,
70.4615552278131));
#205624=CARTESIAN_POINT('Ctrl Pts',(-29.3224102244011,-61.9969896193244,
72.1714716312305));
#205625=CARTESIAN_POINT('Ctrl Pts',(-29.3035783644143,-61.9714118259082,
73.037208427361));
#205626=CARTESIAN_POINT('Ctrl Pts',(-29.265745472525,-62.0904804272812,
74.7336990427337));
#205627=CARTESIAN_POINT('Ctrl Pts',(-29.2469537725319,-62.2295006742594,
75.5607405632176));
#205628=CARTESIAN_POINT('Ctrl Pts',(-29.2192323662553,-62.5551834904872,
76.7703707735546));
#205629=CARTESIAN_POINT('Ctrl Pts',(-29.2100854648056,-62.6825569506798,
77.1666467030544));
#205630=CARTESIAN_POINT('Ctrl Pts',(-29.1977659444505,-62.8786772013591,
77.6892895044013));
#205631=CARTESIAN_POINT('Ctrl Pts',(-29.1946243175987,-62.9308090557598,
77.8215729206249));
#205632=CARTESIAN_POINT('Ctrl Pts',(-29.1914736244731,-62.9850802944281,
77.9529305295057));
#205633=CARTESIAN_POINT('Ctrl Pts',(-30.6991941617974,-62.9850802944281,
77.9529305295057));
#205634=CARTESIAN_POINT('Ctrl Pts',(-30.6834875022977,-63.2546150961368,
78.6053100942889));
#205635=CARTESIAN_POINT('Ctrl Pts',(-30.6680646534122,-63.5769357250135,
79.2348940795638));
#205636=CARTESIAN_POINT('Ctrl Pts',(-30.6351661799762,-64.3585113190455,
80.4964509355169));
#205637=CARTESIAN_POINT('Ctrl Pts',(-30.617686959713,-64.8265610851101,
81.1194423482921));
#205638=CARTESIAN_POINT('Ctrl Pts',(-30.5812917504611,-65.9230302133756,
82.3348469913923));
#205639=CARTESIAN_POINT('Ctrl Pts',(-30.5625565966539,-66.5604279558448,
82.9142072904607));
#205640=CARTESIAN_POINT('Ctrl Pts',(-30.5341175409341,-67.5858569784203,
83.6755700981386));
#205641=CARTESIAN_POINT('Ctrl Pts',(-30.524759796166,-67.9332224300424,
83.9083818207445));
#205642=CARTESIAN_POINT('Ctrl Pts',(-30.4961757833447,-69.0281749019354,
84.5680775452673));
#205643=CARTESIAN_POINT('Ctrl Pts',(-30.4773744419406,-69.8074164205763,
84.9378379287985));
#205644=CARTESIAN_POINT('Ctrl Pts',(-30.4407631920056,-71.363013246297,
85.49486628652));
#205645=CARTESIAN_POINT('Ctrl Pts',(-30.4229673875379,-72.1314036944881,
85.6931514335511));
#205646=CARTESIAN_POINT('Ctrl Pts',(-30.3882077810968,-73.6741446105418,
85.9440701974626));
#205647=CARTESIAN_POINT('Ctrl Pts',(-30.3713805720921,-74.4447547431935,
85.9998966561631));
#205648=CARTESIAN_POINT('Ctrl Pts',(-30.3381954147462,-75.9384620544506,
85.9751027001332));
#205649=CARTESIAN_POINT('Ctrl Pts',(-30.3219380215226,-76.6589057223357,
85.9028536120398));
#205650=CARTESIAN_POINT('Ctrl Pts',(-30.2898766920797,-78.0783486956509,
85.6397139236142));
#205651=CARTESIAN_POINT('Ctrl Pts',(-30.2741277391873,-78.7749469039115,
85.4496026577444));
#205652=CARTESIAN_POINT('Ctrl Pts',(-30.2410058827323,-80.17670479936,84.9386341964782));
#205653=CARTESIAN_POINT('Ctrl Pts',(-30.2236501801243,-80.8762842245382,
84.6105912010411));
#205654=CARTESIAN_POINT('Ctrl Pts',(-30.1889939369837,-82.2264106548325,
83.8242530979522));
#205655=CARTESIAN_POINT('Ctrl Pts',(-30.1717043987287,-82.8723858416748,
83.3644214828119));
#205656=CARTESIAN_POINT('Ctrl Pts',(-30.1349447443021,-84.1251055584975,
82.2879618490551));
#205657=CARTESIAN_POINT('Ctrl Pts',(-30.1156198528516,-84.720402534393,
81.6638006619738));
#205658=CARTESIAN_POINT('Ctrl Pts',(-30.0874233500389,-85.5067000810964,
80.6559535241312));
#205659=CARTESIAN_POINT('Ctrl Pts',(-30.0782309027172,-85.7477067400808,
80.3142848458829));
#205660=CARTESIAN_POINT('Ctrl Pts',(-30.0499477074069,-86.432701672043,
79.2364185980071));
#205661=CARTESIAN_POINT('Ctrl Pts',(-30.0306136796111,-86.8205316189747,
78.4673298953421));
#205662=CARTESIAN_POINT('Ctrl Pts',(-29.9943582613737,-87.4084050070124,
76.9426142362739));
#205663=CARTESIAN_POINT('Ctrl Pts',(-29.9774277284058,-87.6219691973624,
76.1961243245901));
#205664=CARTESIAN_POINT('Ctrl Pts',(-29.9410515613661,-87.9296922244751,
74.5899724056542));
#205665=CARTESIAN_POINT('Ctrl Pts',(-29.9217091327305,-88.0073005875433,
73.7308796686119));
#205666=CARTESIAN_POINT('Ctrl Pts',(-29.8935307168148,-87.9956649448971,
72.4539048682318));
#205667=CARTESIAN_POINT('Ctrl Pts',(-29.8843706324287,-87.9718515197332,
72.0377932595794));
#205668=CARTESIAN_POINT('Ctrl Pts',(-29.8566521965401,-87.8403258599408,
70.7924099816888));
#205669=CARTESIAN_POINT('Ctrl Pts',(-29.8378757243073,-87.6726051772351,
69.9716799218347));
#205670=CARTESIAN_POINT('Ctrl Pts',(-29.8008659262362,-87.1840607839475,
68.3807326608909));
#205671=CARTESIAN_POINT('Ctrl Pts',(-29.7827974452962,-86.8656900947358,
67.6137753751178));
#205672=CARTESIAN_POINT('Ctrl Pts',(-29.7452214015567,-86.0723171916274,
66.1227272554252));
#205673=CARTESIAN_POINT('Ctrl Pts',(-29.7258844671488,-85.5937076972293,
65.4051068092107));
#205674=CARTESIAN_POINT('Ctrl Pts',(-29.69769942545,-84.7831071765765,64.4177329142406));
#205675=CARTESIAN_POINT('Ctrl Pts',(-29.6885278844453,-84.5031384581846,
64.1083337404917));
#205676=CARTESIAN_POINT('Ctrl Pts',(-29.6608129837716,-83.6194854807112,
63.2215199236546));
#205677=CARTESIAN_POINT('Ctrl Pts',(-29.642050821599,-82.9745871531718,
62.6882592595166));
#205678=CARTESIAN_POINT('Ctrl Pts',(-29.6057630222183,-81.622457439973,
61.7737650850085));
#205679=CARTESIAN_POINT('Ctrl Pts',(-29.5883632773671,-80.9221760565283,
61.3887258931024));
#205680=CARTESIAN_POINT('Ctrl Pts',(-29.5534121049914,-79.4809533117132,
60.761014219963));
#205681=CARTESIAN_POINT('Ctrl Pts',(-29.5359768303154,-78.7446455743179,
60.5158180760146));
#205682=CARTESIAN_POINT('Ctrl Pts',(-29.5059736902797,-77.4249776149149,
60.2038333839358));
#205683=CARTESIAN_POINT('Ctrl Pts',(-29.4932246054559,-76.8507107369019,
60.1081656154282));
#205684=CARTESIAN_POINT('Ctrl Pts',(-29.4612737537624,-75.4163655160643,
59.967146810556));
#205685=CARTESIAN_POINT('Ctrl Pts',(-29.4419130739226,-74.5545228835481,
59.9681102913339));
#205686=CARTESIAN_POINT('Ctrl Pts',(-29.4005791689679,-72.6975463410855,
60.1548729748301));
#205687=CARTESIAN_POINT('Ctrl Pts',(-29.3785386832832,-71.7110658675101,
60.3715921265403));
#205688=CARTESIAN_POINT('Ctrl Pts',(-29.3466721256527,-70.3641054547977,
60.8363818267652));
#205689=CARTESIAN_POINT('Ctrl Pts',(-29.3372957503625,-69.9755182409595,
60.9918254576043));
#205690=CARTESIAN_POINT('Ctrl Pts',(-29.3109609411101,-68.8961026251919,
61.4852749580094));
#205691=CARTESIAN_POINT('Ctrl Pts',(-29.2941686401751,-68.2268157522594,
61.8661788100289));
#205692=CARTESIAN_POINT('Ctrl Pts',(-29.257940853399,-66.8878720503737,
62.7940971908772));
#205693=CARTESIAN_POINT('Ctrl Pts',(-29.2385928281301,-66.2310421640931,
63.3532370354826));
#205694=CARTESIAN_POINT('Ctrl Pts',(-29.2104223633023,-65.3457869125314,
64.2728569247223));
#205695=CARTESIAN_POINT('Ctrl Pts',(-29.2012756705988,-65.0718384593771,
64.5862314377127));
#205696=CARTESIAN_POINT('Ctrl Pts',(-29.1735542263521,-64.2935483120385,
65.5678390535729));
#205697=CARTESIAN_POINT('Ctrl Pts',(-29.1547622954661,-63.8382237515122,
66.2721318653139));
#205698=CARTESIAN_POINT('Ctrl Pts',(-29.1169163552933,-63.0564883780533,
67.7831284393971));
#205699=CARTESIAN_POINT('Ctrl Pts',(-29.0980723811611,-62.7368132410658,
68.5886992064822));
#205700=CARTESIAN_POINT('Ctrl Pts',(-29.0596712387894,-62.2632974701733,
70.2472623241974));
#205701=CARTESIAN_POINT('Ctrl Pts',(-29.0403605035061,-62.1098190770359,
71.0959136064054));
#205702=CARTESIAN_POINT('Ctrl Pts',(-29.0121546226142,-62.0079551746448,
72.370799304808));
#205703=CARTESIAN_POINT('Ctrl Pts',(-29.002942850328,-61.9947894974669,
72.7894815358302));
#205704=CARTESIAN_POINT('Ctrl Pts',(-28.9746278241255,-62.016337702273,
74.067379836155));
#205705=CARTESIAN_POINT('Ctrl Pts',(-28.9552819832539,-62.1160057774037,
74.9231370905748));
#205706=CARTESIAN_POINT('Ctrl Pts',(-28.9192277040408,-62.4629931277269,
76.5118656446705));
#205707=CARTESIAN_POINT('Ctrl Pts',(-28.9024715478143,-62.6924955033703,
77.2447609816684));
#205708=CARTESIAN_POINT('Ctrl Pts',(-28.8854250924612,-62.9850802944281,
77.9529305295057));
#205709=CARTESIAN_POINT('Origin',(-21.6548258024609,-75.,72.98888938658));
#205710=CARTESIAN_POINT('',(-32.819270903196,-62.9850802944281,77.9529305295057));
#205711=CARTESIAN_POINT('',(-32.5134098057851,-62.9850802944281,77.9529305295057));
#205712=CARTESIAN_POINT('',(-21.6548258024609,-62.9850802944281,77.9529305295057));
#205713=CARTESIAN_POINT('',(-31.8032572668915,-84.3357280630092,63.9421119750625));
#205714=CARTESIAN_POINT('Ctrl Pts',(-31.8032572668915,-84.3357280630092,
63.9421119750625));
#205715=CARTESIAN_POINT('Ctrl Pts',(-31.8137268296502,-84.6662804770869,
64.2832221083208));
#205716=CARTESIAN_POINT('Ctrl Pts',(-31.8242105474278,-84.9778883827939,
64.6421916720238));
#205717=CARTESIAN_POINT('Ctrl Pts',(-31.8452661078821,-85.558044034709,
65.3895689566823));
#205718=CARTESIAN_POINT('Ctrl Pts',(-31.8558207746628,-85.8264924884276,
65.7771611941525));
#205719=CARTESIAN_POINT('Ctrl Pts',(-31.8870392024047,-86.5581835076886,
66.9668434036295));
#205720=CARTESIAN_POINT('Ctrl Pts',(-31.9072090633639,-86.9574808246518,
67.804750359145));
#205721=CARTESIAN_POINT('Ctrl Pts',(-31.9438558392689,-87.5045856463217,
69.361228744241));
#205722=CARTESIAN_POINT('Ctrl Pts',(-31.9601457568728,-87.6872416449994,
70.0634020317026));
#205723=CARTESIAN_POINT('Ctrl Pts',(-31.993669338487,-87.9440636466703,
71.5509028311772));
#205724=CARTESIAN_POINT('Ctrl Pts',(-32.0108132108122,-88.007278414284,
72.3352026728299));
#205725=CARTESIAN_POINT('Ctrl Pts',(-32.041413459719,-87.9933581299314,
73.7111701669863));
#205726=CARTESIAN_POINT('Ctrl Pts',(-32.0546718044928,-87.9471161615131,
74.3008439158162));
#205727=CARTESIAN_POINT('Ctrl Pts',(-32.0851344571267,-87.7478091296771,
75.6524738326175));
#205728=CARTESIAN_POINT('Ctrl Pts',(-32.1020536637848,-87.5662736943747,
76.4079661630273));
#205729=CARTESIAN_POINT('Ctrl Pts',(-32.1370010492423,-87.0627838574,77.9010874580178));
#205730=CARTESIAN_POINT('Ctrl Pts',(-32.1550099680091,-86.7375957907177,
78.6341778642299));
#205731=CARTESIAN_POINT('Ctrl Pts',(-32.1912934650356,-85.9396264269875,
80.0614936447038));
#205732=CARTESIAN_POINT('Ctrl Pts',(-32.2095283583469,-85.4629113018594,
80.7493438556071));
#205733=CARTESIAN_POINT('Ctrl Pts',(-32.2401738889961,-84.5742243220643,
81.7994869097814));
#205734=CARTESIAN_POINT('Ctrl Pts',(-32.2523110403474,-84.1995002523804,
82.1900628608691));
#205735=CARTESIAN_POINT('Ctrl Pts',(-32.2737175034811,-83.4924804529018,
82.8404954068366));
#205736=CARTESIAN_POINT('Ctrl Pts',(-32.2829621282018,-83.1698192144293,
83.109680843072));
#205737=CARTESIAN_POINT('Ctrl Pts',(-32.3106727048045,-82.1666891250305,
83.8672771165417));
#205738=CARTESIAN_POINT('Ctrl Pts',(-32.3292499662116,-81.4515148297491,
84.3060753253936));
#205739=CARTESIAN_POINT('Ctrl Pts',(-32.3662481136558,-79.9652516271433,
85.0310242120193));
#205740=CARTESIAN_POINT('Ctrl Pts',(-32.3841858647311,-79.1992642429188,
85.3190523791631));
#205741=CARTESIAN_POINT('Ctrl Pts',(-32.4220642430902,-77.5452463858179,
85.7688466228141));
#205742=CARTESIAN_POINT('Ctrl Pts',(-32.4422074650899,-76.6570952085571,
85.9140432257214));
#205743=CARTESIAN_POINT('Ctrl Pts',(-32.4792994256479,-74.9927441127254,
86.0116521763215));
#205744=CARTESIAN_POINT('Ctrl Pts',(-32.4960937321176,-74.2219013652736,
85.988388222726));
#205745=CARTESIAN_POINT('Ctrl Pts',(-32.529353314226,-72.7348060805604,
85.81070167596));
#205746=CARTESIAN_POINT('Ctrl Pts',(-32.5457254327998,-72.0204897610094,
85.6637655202297));
#205747=CARTESIAN_POINT('Ctrl Pts',(-32.579257934671,-70.5726847695437,
85.2367297597932));
#205748=CARTESIAN_POINT('Ctrl Pts',(-32.5963180037202,-69.8445870749277,
84.9485064312127));
#205749=CARTESIAN_POINT('Ctrl Pts',(-32.6269769784201,-68.6132659357982,
84.3276132039394));
#205750=CARTESIAN_POINT('Ctrl Pts',(-32.6403853306936,-68.0989226873159,
84.0221191075195));
#205751=CARTESIAN_POINT('Ctrl Pts',(-32.6630886340244,-67.2613979801993,
83.4431226889983));
#205752=CARTESIAN_POINT('Ctrl Pts',(-32.6723570558202,-66.9271902569869,
83.187256821882));
#205753=CARTESIAN_POINT('Ctrl Pts',(-32.7088904509961,-65.6616023646648,
82.117080093252));
#205754=CARTESIAN_POINT('Ctrl Pts',(-32.7366344037597,-64.8359994051929,
81.1878295620108));
#205755=CARTESIAN_POINT('Ctrl Pts',(-32.7731968005128,-63.924608112052,
79.8086445818466));
#205756=CARTESIAN_POINT('Ctrl Pts',(-32.7823439576573,-63.7118757009843,
79.450438499197));
#205757=CARTESIAN_POINT('Ctrl Pts',(-32.8007461567169,-63.3213674514892,
78.7145499636195));
#205758=CARTESIAN_POINT('Ctrl Pts',(-32.8099846903507,-63.1439812735294,
78.3375330035928));
#205759=CARTESIAN_POINT('Ctrl Pts',(-32.819270903196,-62.9850802944281,
77.9529305295057));
#205760=CARTESIAN_POINT('Ctrl Pts',(-31.8032546359728,-84.3357281078424,
63.9421120213277));
#205761=CARTESIAN_POINT('Ctrl Pts',(-31.7929017891933,-84.0137418231872,
63.6098416131334));
#205762=CARTESIAN_POINT('Ctrl Pts',(-31.7825782414718,-83.6742452764102,
63.2949969769354));
#205763=CARTESIAN_POINT('Ctrl Pts',(-31.762142865887,-82.9657881833782,
62.7050617455991));
#205764=CARTESIAN_POINT('Ctrl Pts',(-31.7520438876031,-82.5975654591075,
62.4301067000986));
#205765=CARTESIAN_POINT('Ctrl Pts',(-31.7220978906036,-81.4682498818366,
61.6765559885635));
#205766=CARTESIAN_POINT('Ctrl Pts',(-31.701905426842,-80.6712518671031,
61.2567099106229));
#205767=CARTESIAN_POINT('Ctrl Pts',(-31.6687054766057,-79.2851099112889,
60.7010161848905));
#205768=CARTESIAN_POINT('Ctrl Pts',(-31.6556315862844,-78.7183126943624,
60.5177969698974));
#205769=CARTESIAN_POINT('Ctrl Pts',(-31.6235092294182,-77.3059802936444,
60.1661409326779));
#205770=CARTESIAN_POINT('Ctrl Pts',(-31.6041600695629,-76.4524164504797,
60.0416541758202));
#205771=CARTESIAN_POINT('Ctrl Pts',(-31.5670832372624,-74.7868628847689,
59.9656208321883));
#205772=CARTESIAN_POINT('Ctrl Pts',(-31.5494826207861,-73.9792130438151,
60.0039389183364));
#205773=CARTESIAN_POINT('Ctrl Pts',(-31.5129772878929,-72.3534111569085,
60.2337707384166));
#205774=CARTESIAN_POINT('Ctrl Pts',(-31.4942105742096,-71.5396614362397,
60.4300854548566));
#205775=CARTESIAN_POINT('Ctrl Pts',(-31.4664944723401,-70.3564077373968,
60.8393694015009));
#205776=CARTESIAN_POINT('Ctrl Pts',(-31.4573265264178,-69.9692181927887,
60.9945148918131));
#205777=CARTESIAN_POINT('Ctrl Pts',(-31.4291434374201,-68.8077276326911,
61.526072404452));
#205778=CARTESIAN_POINT('Ctrl Pts',(-31.4098046293393,-68.0627862461729,
61.9609491845076));
#205779=CARTESIAN_POINT('Ctrl Pts',(-31.3715448957847,-66.6707011023987,
62.9708420211181));
#205780=CARTESIAN_POINT('Ctrl Pts',(-31.352820942403,-66.026857096905,63.5431921538024));
#205781=CARTESIAN_POINT('Ctrl Pts',(-31.3244008168015,-65.1616248295522,
64.4812402729385));
#205782=CARTESIAN_POINT('Ctrl Pts',(-31.3150537873411,-64.893933566602,
64.801023931398));
#205783=CARTESIAN_POINT('Ctrl Pts',(-31.2846353628715,-64.0711633671607,
65.8858559643348));
#205784=CARTESIAN_POINT('Ctrl Pts',(-31.2639758907107,-63.5840156743489,
66.6985915452734));
#205785=CARTESIAN_POINT('Ctrl Pts',(-31.2239921695654,-62.8300913154623,
68.3378479345733));
#205786=CARTESIAN_POINT('Ctrl Pts',(-31.2046388496943,-62.5492623479359,
69.1524847619243));
#205787=CARTESIAN_POINT('Ctrl Pts',(-31.1763003470951,-62.2541577943955,
70.396740923088));
#205788=CARTESIAN_POINT('Ctrl Pts',(-31.167074447028,-62.1772042064713,
70.8090646931028));
#205789=CARTESIAN_POINT('Ctrl Pts',(-31.1388631048973,-62.0035560249431,
72.0765788918956));
#205790=CARTESIAN_POINT('Ctrl Pts',(-31.119565396247,-61.9716734969528,
72.9382579515243));
#205791=CARTESIAN_POINT('Ctrl Pts',(-31.0808490166685,-62.0797097403603,
74.6734180662941));
#205792=CARTESIAN_POINT('Ctrl Pts',(-31.0617070857034,-62.2230046580078,
75.5423030227853));
#205793=CARTESIAN_POINT('Ctrl Pts',(-31.029900986821,-62.5970165804909,
76.9220559866024));
#205794=CARTESIAN_POINT('Ctrl Pts',(-31.0175294395029,-62.7748319708431,
77.4440474132357));
#205795=CARTESIAN_POINT('Ctrl Pts',(-31.0052564152503,-62.9850802944281,
77.9529305295057));
#205796=CARTESIAN_POINT('Ctrl Pts',(-32.5134098057851,-62.9850802944281,
77.9529305295057));
#205797=CARTESIAN_POINT('Ctrl Pts',(-32.5076053766535,-63.0852617434361,
78.1954087908987));
#205798=CARTESIAN_POINT('Ctrl Pts',(-32.5017802649863,-63.1928105147828,
78.4349197211954));
#205799=CARTESIAN_POINT('Ctrl Pts',(-32.4838237910791,-63.5451785962135,
79.1599913731993));
#205800=CARTESIAN_POINT('Ctrl Pts',(-32.4716239056369,-63.813181450543,
79.6334752954121));
#205801=CARTESIAN_POINT('Ctrl Pts',(-32.442315516669,-64.5315142181605,
80.7352684005586));
#205802=CARTESIAN_POINT('Ctrl Pts',(-32.4254786019266,-65.0097267370101,
81.3429317606586));
#205803=CARTESIAN_POINT('Ctrl Pts',(-32.3909713539776,-66.0764202871788,
82.4748668122886));
#205804=CARTESIAN_POINT('Ctrl Pts',(-32.3733389564417,-66.6642977390282,
82.995392432135));
#205805=CARTESIAN_POINT('Ctrl Pts',(-32.3374292549746,-67.9675929300343,
83.9543629803537));
#205806=CARTESIAN_POINT('Ctrl Pts',(-32.3192073754178,-68.6857914976066,
84.3830607366462));
#205807=CARTESIAN_POINT('Ctrl Pts',(-32.291326621253,-69.8172587654147,
84.918402285109));
#205808=CARTESIAN_POINT('Ctrl Pts',(-32.2819823861496,-70.2027807287757,
85.0785862771025));
#205809=CARTESIAN_POINT('Ctrl Pts',(-32.2534174636685,-71.4048932028122,
85.5114924043552));
#205810=CARTESIAN_POINT('Ctrl Pts',(-32.2346243519322,-72.2413974206223,
85.7219366544957));
#205811=CARTESIAN_POINT('Ctrl Pts',(-32.1970943895163,-73.9163500386038,
85.9703877836411));
#205812=CARTESIAN_POINT('Ctrl Pts',(-32.178350446336,-74.7499965381135,
86.0131394055838));
#205813=CARTESIAN_POINT('Ctrl Pts',(-32.1413374836823,-76.4170147775859,
85.9384356609712));
#205814=CARTESIAN_POINT('Ctrl Pts',(-32.1230775115974,-77.2464955062173,
85.8205668316705));
#205815=CARTESIAN_POINT('Ctrl Pts',(-32.0951739658194,-78.4636969776953,
85.5258852841211));
#205816=CARTESIAN_POINT('Ctrl Pts',(-32.085844592053,-78.8635482433997,
85.4084890933288));
#205817=CARTESIAN_POINT('Ctrl Pts',(-32.0573013444042,-80.0701001412522,
84.9903267017186));
#205818=CARTESIAN_POINT('Ctrl Pts',(-32.0385165171516,-80.8531448342645,
84.6285246885511));
#205819=CARTESIAN_POINT('Ctrl Pts',(-32.0003877748412,-82.3352085699554,
83.7561132100218));
#205820=CARTESIAN_POINT('Ctrl Pts',(-31.9810362370968,-83.0306905604942,
83.2478562689681));
#205821=CARTESIAN_POINT('Ctrl Pts',(-31.9434043043225,-84.2968599059186,
82.1143586018015));
#205822=CARTESIAN_POINT('Ctrl Pts',(-31.9250226552402,-84.8670083633218,
81.4946488408057));
#205823=CARTESIAN_POINT('Ctrl Pts',(-31.8913008487649,-85.7783267450898,
80.2881430609645));
#205824=CARTESIAN_POINT('Ctrl Pts',(-31.8762028643039,-86.1411164443342,
79.7214196296445));
#205825=CARTESIAN_POINT('Ctrl Pts',(-31.8521446795649,-86.6550981991082,
78.7622750048645));
#205826=CARTESIAN_POINT('Ctrl Pts',(-31.8429987285859,-86.8339861382299,
78.3861172138805));
#205827=CARTESIAN_POINT('Ctrl Pts',(-31.8138207580393,-87.3432442577997,
77.1676574911561));
#205828=CARTESIAN_POINT('Ctrl Pts',(-31.793529191697,-87.6039568424936,
76.2991814038458));
#205829=CARTESIAN_POINT('Ctrl Pts',(-31.7542862800609,-87.9325327509782,
74.5663075747454));
#205830=CARTESIAN_POINT('Ctrl Pts',(-31.7355537691597,-88.0085120462363,
73.7081052595353));
#205831=CARTESIAN_POINT('Ctrl Pts',(-31.7071035079715,-87.9947289921439,
72.430020848856));
#205832=CARTESIAN_POINT('Ctrl Pts',(-31.6977308116469,-87.9699889375341,
72.0118011787893));
#205833=CARTESIAN_POINT('Ctrl Pts',(-31.6691269442241,-87.8329027110215,
70.7401793866785));
#205834=CARTESIAN_POINT('Ctrl Pts',(-31.6503158982419,-87.6560195593421,
69.8961139094583));
#205835=CARTESIAN_POINT('Ctrl Pts',(-31.6120804853365,-87.1363994018851,
68.2499349011304));
#205836=CARTESIAN_POINT('Ctrl Pts',(-31.5925892045241,-86.7938770755704,
67.4522536129843));
#205837=CARTESIAN_POINT('Ctrl Pts',(-31.5548346790839,-85.9694660877567,
65.9624419093435));
#205838=CARTESIAN_POINT('Ctrl Pts',(-31.5365502141308,-85.494589124122,
65.2711334018083));
#205839=CARTESIAN_POINT('Ctrl Pts',(-31.5086330202524,-84.6891200693539,
64.3116785261865));
#205840=CARTESIAN_POINT('Ctrl Pts',(-31.4993140041212,-84.4065224252938,
64.0061074697714));
#205841=CARTESIAN_POINT('Ctrl Pts',(-31.4707861257568,-83.4958975907463,
63.1116359011595));
#205842=CARTESIAN_POINT('Ctrl Pts',(-31.4520065931275,-82.8236812233962,
62.5710956883294));
#205843=CARTESIAN_POINT('Ctrl Pts',(-31.4150123713188,-81.4264517085648,
61.6595801380764));
#205844=CARTESIAN_POINT('Ctrl Pts',(-31.3968335975869,-80.7102333464946,
61.2822349818434));
#205845=CARTESIAN_POINT('Ctrl Pts',(-31.3603815270131,-79.1917448914674,
60.6549203171202));
#205846=CARTESIAN_POINT('Ctrl Pts',(-31.3421407050194,-78.3909075940815,
60.4111601434876));
#205847=CARTESIAN_POINT('Ctrl Pts',(-31.3142483880798,-77.1636092287094,
60.1634234396562));
#205848=CARTESIAN_POINT('Ctrl Pts',(-31.3049113604121,-76.7512490389828,
60.1006425146734));
#205849=CARTESIAN_POINT('Ctrl Pts',(-31.2763568826858,-75.480682155363,
59.9693138771131));
#205850=CARTESIAN_POINT('Ctrl Pts',(-31.2575678912659,-74.6181058614249,
59.9660417654655));
#205851=CARTESIAN_POINT('Ctrl Pts',(-31.2212335497617,-72.9864717788575,
60.1221898828707));
#205852=CARTESIAN_POINT('Ctrl Pts',(-31.2037330422133,-72.219625510468,
60.2658489202725));
#205853=CARTESIAN_POINT('Ctrl Pts',(-31.1673159191293,-70.6432895169942,
60.7105594863258));
#205854=CARTESIAN_POINT('Ctrl Pts',(-31.1485808352973,-69.8414825742706,
61.0252771805082));
#205855=CARTESIAN_POINT('Ctrl Pts',(-31.1201415341838,-68.7045718189878,
61.6072261041865));
#205856=CARTESIAN_POINT('Ctrl Pts',(-31.1107834724493,-68.3419367698086,
61.8154893693561));
#205857=CARTESIAN_POINT('Ctrl Pts',(-31.082199021831,-67.2653733681447,
62.5048137772382));
#205858=CARTESIAN_POINT('Ctrl Pts',(-31.0633974799748,-66.5886292737129,
63.0395610118058));
#205859=CARTESIAN_POINT('Ctrl Pts',(-31.0255413684423,-65.3595946174076,
64.2263624187867));
#205860=CARTESIAN_POINT('Ctrl Pts',(-31.0064524824918,-64.8086145122379,
64.8737831689563));
#205861=CARTESIAN_POINT('Ctrl Pts',(-30.9690972310508,-63.8473904397092,
66.2569751884845));
#205862=CARTESIAN_POINT('Ctrl Pts',(-30.9508258173321,-63.4375302189977,
66.9881669649071));
#205863=CARTESIAN_POINT('Ctrl Pts',(-30.9229157934444,-62.9331182219311,
68.1346509919764));
#205864=CARTESIAN_POINT('Ctrl Pts',(-30.9135911765594,-62.7838849288901,
68.5234893095958));
#205865=CARTESIAN_POINT('Ctrl Pts',(-30.8850549659496,-62.3841643947466,
69.7360280741739));
#205866=CARTESIAN_POINT('Ctrl Pts',(-30.8662726182641,-62.1965672448327,
70.5779713737612));
#205867=CARTESIAN_POINT('Ctrl Pts',(-30.8291649365254,-61.9961730712194,
72.239492048222));
#205868=CARTESIAN_POINT('Ctrl Pts',(-30.8108665953323,-61.9747608962482,
73.054081626788));
#205869=CARTESIAN_POINT('Ctrl Pts',(-30.7742958529931,-62.0858921114305,
74.6987386395822));
#205870=CARTESIAN_POINT('Ctrl Pts',(-30.7560509418798,-62.2224047141963,
75.5247984193269));
#205871=CARTESIAN_POINT('Ctrl Pts',(-30.7281561875893,-62.5444063035,76.7348072071708));
#205872=CARTESIAN_POINT('Ctrl Pts',(-30.7188207626434,-62.6708981172921,
77.1321924653583));
#205873=CARTESIAN_POINT('Ctrl Pts',(-30.706059194963,-62.8699996949342,
77.6672262769554));
#205874=CARTESIAN_POINT('Ctrl Pts',(-30.7026204047894,-62.9262841051138,
77.8106207715354));
#205875=CARTESIAN_POINT('Ctrl Pts',(-30.6991941617974,-62.9850802944281,
77.9529305295057));
#205876=CARTESIAN_POINT('Origin',(-21.6548258024609,-75.,72.98888938658));
#205877=CARTESIAN_POINT('',(-34.6333744106366,-62.9850802944281,77.9529305295057));
#205878=CARTESIAN_POINT('',(-34.3273949797549,-62.9850802944281,77.9529305295057));
#205879=CARTESIAN_POINT('',(-21.6548258024609,-62.9850802944281,77.9529305295057));
#205880=CARTESIAN_POINT('Ctrl Pts',(-32.819270903196,-62.9850802944281,
77.9529305295057));
#205881=CARTESIAN_POINT('Ctrl Pts',(-32.8303488181902,-62.7955206140402,
77.4941220156964));
#205882=CARTESIAN_POINT('Ctrl Pts',(-32.8414992495208,-62.6322673893811,
77.0245186000302));
#205883=CARTESIAN_POINT('Ctrl Pts',(-32.8618815752937,-62.3816084436316,
76.1435119333727));
#205884=CARTESIAN_POINT('Ctrl Pts',(-32.8710913751594,-62.2865225690053,
75.7353309164621));
#205885=CARTESIAN_POINT('Ctrl Pts',(-32.9028830983415,-62.0275972955214,
74.3168337901965));
#205886=CARTESIAN_POINT('Ctrl Pts',(-32.9257513877221,-61.9633350804462,
73.2922177203429));
#205887=CARTESIAN_POINT('Ctrl Pts',(-32.9578895657514,-62.0430373705422,
71.8516723340877));
#205888=CARTESIAN_POINT('Ctrl Pts',(-32.9671254965868,-62.0865020708477,
71.433989150719));
#205889=CARTESIAN_POINT('Ctrl Pts',(-32.9948120157051,-62.2768003706303,
70.1925542543176));
#205890=CARTESIAN_POINT('Ctrl Pts',(-33.0133768145488,-62.4829681329178,
69.3801222078165));
#205891=CARTESIAN_POINT('Ctrl Pts',(-33.0503473708614,-63.0417179721099,
67.8250052856451));
#205892=CARTESIAN_POINT('Ctrl Pts',(-33.0682709487124,-63.3894385363193,
67.0845625800919));
#205893=CARTESIAN_POINT('Ctrl Pts',(-33.1060393670685,-64.257983751471,
65.6128504297507));
#205894=CARTESIAN_POINT('Ctrl Pts',(-33.1260757069405,-64.7896612828076,
64.8928516144764));
#205895=CARTESIAN_POINT('Ctrl Pts',(-33.1650532965956,-65.9697286661664,
63.5977881523641));
#205896=CARTESIAN_POINT('Ctrl Pts',(-33.1837862151397,-66.6101315099571,
63.0215078096652));
#205897=CARTESIAN_POINT('Ctrl Pts',(-33.2122343360639,-67.6399968300279,
62.2648258556167));
#205898=CARTESIAN_POINT('Ctrl Pts',(-33.2216040891035,-67.9890639397373,
62.03343596658));
#205899=CARTESIAN_POINT('Ctrl Pts',(-33.2502042061045,-69.0878649514756,
61.3791175769157));
#205900=CARTESIAN_POINT('Ctrl Pts',(-33.2690133164106,-69.8689186312676,
61.0134082367942));
#205901=CARTESIAN_POINT('Ctrl Pts',(-33.3071691200651,-71.4935665018307,
60.4410481577551));
#205902=CARTESIAN_POINT('Ctrl Pts',(-33.3265758030914,-72.3332640196519,
60.2361678442363));
#205903=CARTESIAN_POINT('Ctrl Pts',(-33.3642463882863,-74.0155149179557,
59.9992482292248));
#205904=CARTESIAN_POINT('Ctrl Pts',(-33.3825281393287,-74.8533245389361,
59.9628200418645));
#205905=CARTESIAN_POINT('Ctrl Pts',(-33.4104438619237,-76.1042568462207,
60.0291941259602));
#205906=CARTESIAN_POINT('Ctrl Pts',(-33.419764058336,-76.5184087177558,
60.0711682849701));
#205907=CARTESIAN_POINT('Ctrl Pts',(-33.4482936964434,-77.7807708737798,
60.2606638026717));
#205908=CARTESIAN_POINT('Ctrl Pts',(-33.4670738130376,-78.6169260116809,
60.4725696178896));
#205909=CARTESIAN_POINT('Ctrl Pts',(-33.5040917123383,-80.186566440543,
61.0409253788097));
#205910=CARTESIAN_POINT('Ctrl Pts',(-33.5222954330852,-80.9197737703172,
61.3867091394883));
#205911=CARTESIAN_POINT('Ctrl Pts',(-33.5587722642639,-82.3350289286893,
62.2234390524097));
#205912=CARTESIAN_POINT('Ctrl Pts',(-33.5770139410402,-83.0113491242323,
62.7167978539842));
#205913=CARTESIAN_POINT('Ctrl Pts',(-33.6049067692322,-83.947247329626,
63.5485221842696));
#205914=CARTESIAN_POINT('Ctrl Pts',(-33.6142434632672,-84.2453394212993,
63.8402574857912));
#205915=CARTESIAN_POINT('Ctrl Pts',(-33.6427974541876,-85.1142196463574,
64.7765228903436));
#205916=CARTESIAN_POINT('Ctrl Pts',(-33.6615862595611,-85.6354756538642,
65.4637939289738));
#205917=CARTESIAN_POINT('Ctrl Pts',(-33.6989489121466,-86.5159865149227,
66.9009770269514));
#205918=CARTESIAN_POINT('Ctrl Pts',(-33.7175161856982,-86.8790333380158,
67.6438747237403));
#205919=CARTESIAN_POINT('Ctrl Pts',(-33.7543538268296,-87.4631659122686,
69.1983991735322));
#205920=CARTESIAN_POINT('Ctrl Pts',(-33.7726078625132,-87.6809979278511,
70.0071749752059));
#205921=CARTESIAN_POINT('Ctrl Pts',(-33.8005079783443,-87.8888404294256,
71.2420764442562));
#205922=CARTESIAN_POINT('Ctrl Pts',(-33.809839765355,-87.9381973326846,
71.6559933457568));
#205923=CARTESIAN_POINT('Ctrl Pts',(-33.838386567099,-88.0283126189074,
72.9298890005096));
#205924=CARTESIAN_POINT('Ctrl Pts',(-33.8571726839098,-88.0036620133458,
73.792124332821));
#205925=CARTESIAN_POINT('Ctrl Pts',(-33.8952999643647,-87.7844960111742,
75.4978903978681));
#205926=CARTESIAN_POINT('Ctrl Pts',(-33.9146515604325,-87.5907485760449,
76.3372431692137));
#205927=CARTESIAN_POINT('Ctrl Pts',(-33.9522825945386,-87.0466716428339,
77.9470330997242));
#205928=CARTESIAN_POINT('Ctrl Pts',(-33.9706588111517,-86.7012516996233,
78.7148129789149));
#205929=CARTESIAN_POINT('Ctrl Pts',(-34.0044349709995,-85.9492394717942,
80.0294294550852));
#205930=CARTESIAN_POINT('Ctrl Pts',(-34.0195937256319,-85.5692184286172,
80.5880129405775));
#205931=CARTESIAN_POINT('Ctrl Pts',(-34.043710710229,-84.8873714723516,
81.4395211634468));
#205932=CARTESIAN_POINT('Ctrl Pts',(-34.0528566120177,-84.6117142724853,
81.7517794012562));
#205933=CARTESIAN_POINT('Ctrl Pts',(-34.0820230580383,-83.6915922207639,
82.6983197720169));
#205934=CARTESIAN_POINT('Ctrl Pts',(-34.1023028966374,-82.9957727870719,
83.2789044967711));
#205935=CARTESIAN_POINT('Ctrl Pts',(-34.1415336101152,-81.5318018742164,
84.2616092303533));
#205936=CARTESIAN_POINT('Ctrl Pts',(-34.1602661380666,-80.7724706946262,
84.6686683284463));
#205937=CARTESIAN_POINT('Ctrl Pts',(-34.1887163037608,-79.5917631926907,
85.1581547926365));
#205938=CARTESIAN_POINT('Ctrl Pts',(-34.1980888676959,-79.1974632258503,
85.2997224612759));
#205939=CARTESIAN_POINT('Ctrl Pts',(-34.226692568603,-77.974250045081,85.6732864127809));
#205940=CARTESIAN_POINT('Ctrl Pts',(-34.2455035275443,-77.1285653983452,
85.842266498186));
#205941=CARTESIAN_POINT('Ctrl Pts',(-34.2837353197113,-75.4107807541226,
86.0112103592688));
#205942=CARTESIAN_POINT('Ctrl Pts',(-34.303222750951,-74.5428430101874,
86.0096644763363));
#205943=CARTESIAN_POINT('Ctrl Pts',(-34.3409734567497,-72.8490955860084,
85.8369924859513));
#205944=CARTESIAN_POINT('Ctrl Pts',(-34.3592577985796,-72.0267989571312,
85.6719578850047));
#205945=CARTESIAN_POINT('Ctrl Pts',(-34.387174925936,-70.8280184635038,
85.3082890592474));
#205946=CARTESIAN_POINT('Ctrl Pts',(-34.3964939957936,-70.4359795751436,
85.168493438659));
#205947=CARTESIAN_POINT('Ctrl Pts',(-34.4250219543035,-69.2556313471897,
84.6825903025585));
#205948=CARTESIAN_POINT('Ctrl Pts',(-34.4438015134082,-68.4944285088169,
84.2768454922166));
#205949=CARTESIAN_POINT('Ctrl Pts',(-34.4799213390761,-67.1399896053986,
83.3720786407645));
#205950=CARTESIAN_POINT('Ctrl Pts',(-34.4971936814418,-66.5401658817086,
82.8894741616409));
#205951=CARTESIAN_POINT('Ctrl Pts',(-34.5333759273023,-65.367339869463,
81.7610094243801));
#205952=CARTESIAN_POINT('Ctrl Pts',(-34.5521118107064,-64.808776374574,
81.1053664770553));
#205953=CARTESIAN_POINT('Ctrl Pts',(-34.5805483990371,-64.0808503345902,
80.0561870098963));
#205954=CARTESIAN_POINT('Ctrl Pts',(-34.5899029774752,-63.859392651258,
79.7016676413947));
#205955=CARTESIAN_POINT('Ctrl Pts',(-34.6107233525533,-63.4046850825134,
78.8890800647395));
#205956=CARTESIAN_POINT('Ctrl Pts',(-34.6220712822401,-63.1808895977458,
78.4268655734003));
#205957=CARTESIAN_POINT('Ctrl Pts',(-34.6333744106366,-62.9850802944281,
77.9529305295057));
#205958=CARTESIAN_POINT('',(-33.3112143094267,-84.3357243294104,63.9421081222156));
#205959=CARTESIAN_POINT('Ctrl Pts',(-33.3112143094267,-84.3357243294104,
63.9421081222156));
#205960=CARTESIAN_POINT('Ctrl Pts',(-33.3011567376052,-84.018179448338,
63.6144212482569));
#205961=CARTESIAN_POINT('Ctrl Pts',(-33.2910868185285,-83.6836026922541,
63.3036812712545));
#205962=CARTESIAN_POINT('Ctrl Pts',(-33.270859537395,-82.9856613046251,
62.7207607284952));
#205963=CARTESIAN_POINT('Ctrl Pts',(-33.2607172534439,-82.6229961362875,
62.448719518442));
#205964=CARTESIAN_POINT('Ctrl Pts',(-33.2307972855461,-81.512313296332,
61.7029412195651));
#205965=CARTESIAN_POINT('Ctrl Pts',(-33.2114694583803,-80.7293167802803,
61.2859930717215));
#205966=CARTESIAN_POINT('Ctrl Pts',(-33.1787998006508,-79.3646935367683,
60.7293474205624));
#205967=CARTESIAN_POINT('Ctrl Pts',(-33.1656257625774,-78.8048353287375,
60.5442060876235));
#205968=CARTESIAN_POINT('Ctrl Pts',(-33.1332173327621,-77.4010069115259,
60.1835986577919));
#205969=CARTESIAN_POINT('Ctrl Pts',(-33.1144159002237,-76.5484568928008,
60.0527930603133));
#205970=CARTESIAN_POINT('Ctrl Pts',(-33.0778011775325,-74.8982943026596,
59.9651786904443));
#205971=CARTESIAN_POINT('Ctrl Pts',(-33.0600016200892,-74.1051527881878,
59.9955595269195));
#205972=CARTESIAN_POINT('Ctrl Pts',(-33.0252332862106,-72.5548874686548,
60.1976288909055));
#205973=CARTESIAN_POINT('Ctrl Pts',(-33.0084016440632,-71.8004344901442,
60.3651931764459));
#205974=CARTESIAN_POINT('Ctrl Pts',(-32.975214203434,-70.3764937256837,
60.8173862440033));
#205975=CARTESIAN_POINT('Ctrl Pts',(-32.958959216202,-69.7071313681547,
61.0931828662537));
#205976=CARTESIAN_POINT('Ctrl Pts',(-32.9336299287227,-68.6924594078672,
61.6139391600983));
#205977=CARTESIAN_POINT('Ctrl Pts',(-32.9244502411375,-68.3301624071969,
61.8225189264437));
#205978=CARTESIAN_POINT('Ctrl Pts',(-32.8933811493513,-67.1446714713373,
62.5833361158591));
#205979=CARTESIAN_POINT('Ctrl Pts',(-32.8712073444619,-66.374713381374,
63.2120734643514));
#205980=CARTESIAN_POINT('Ctrl Pts',(-32.8320021167915,-65.1468740655802,
64.4737079533328));
#205981=CARTESIAN_POINT('Ctrl Pts',(-32.8152101770762,-64.6601117225579,
65.0718749085846));
#205982=CARTESIAN_POINT('Ctrl Pts',(-32.7811254811386,-63.8001707228227,
66.34429060657));
#205983=CARTESIAN_POINT('Ctrl Pts',(-32.7638894358816,-63.4281548857308,
67.0156773275925));
#205984=CARTESIAN_POINT('Ctrl Pts',(-32.7283732978745,-62.779158084489,
68.4781778667905));
#205985=CARTESIAN_POINT('Ctrl Pts',(-32.7101654750316,-62.5150246908457,
69.2712427072861));
#205986=CARTESIAN_POINT('Ctrl Pts',(-32.6794071690772,-62.2064347626964,
70.6173912999878));
#205987=CARTESIAN_POINT('Ctrl Pts',(-32.6671274699066,-62.1179749693231,
71.1578394958046));
#205988=CARTESIAN_POINT('Ctrl Pts',(-32.6377330249469,-61.9874232454337,
72.470434962504));
#205989=CARTESIAN_POINT('Ctrl Pts',(-32.6208908717924,-61.9795960428579,
73.2439011138986));
#205990=CARTESIAN_POINT('Ctrl Pts',(-32.5863479185737,-62.1023105176637,
74.7960616240076));
#205991=CARTESIAN_POINT('Ctrl Pts',(-32.5686834978556,-62.2349407008807,
75.5714306412647));
#205992=CARTESIAN_POINT('Ctrl Pts',(-32.5385701469869,-62.5836904218178,
76.8827731080568));
#205993=CARTESIAN_POINT('Ctrl Pts',(-32.5260500510614,-62.7669161892439,
77.4248881279713));
#205994=CARTESIAN_POINT('Ctrl Pts',(-32.5134098057851,-62.9850802944281,
77.9529305295057));
#205995=CARTESIAN_POINT('Ctrl Pts',(-34.3273949797549,-62.9850802944281,
77.9529305295057));
#205996=CARTESIAN_POINT('Ctrl Pts',(-34.322307377864,-63.0729887704614,
78.1657033995463));
#205997=CARTESIAN_POINT('Ctrl Pts',(-34.3172056192574,-63.1665708141729,
78.3761933206329));
#205998=CARTESIAN_POINT('Ctrl Pts',(-34.2949390915263,-63.5977531412717,
79.2804559285437));
#205999=CARTESIAN_POINT('Ctrl Pts',(-34.277572804023,-63.9910798857048,
79.9458085247177));
#206000=CARTESIAN_POINT('Ctrl Pts',(-34.2485826539232,-64.7549730486861,
81.009425030582));
#206001=CARTESIAN_POINT('Ctrl Pts',(-34.2367826841871,-65.0957150793225,
81.4265852338732));
#206002=CARTESIAN_POINT('Ctrl Pts',(-34.2063795532183,-66.0288964681025,
82.4343718864558));
#206003=CARTESIAN_POINT('Ctrl Pts',(-34.187609460991,-66.6542234883961,
82.9911810079837));
#206004=CARTESIAN_POINT('Ctrl Pts',(-34.1509267743499,-67.9861547229964,
83.9647400989129));
#206005=CARTESIAN_POINT('Ctrl Pts',(-34.1331613516227,-68.6873916773296,
84.3824975576726));
#206006=CARTESIAN_POINT('Ctrl Pts',(-34.0959087150043,-70.2003621110454,
85.1010273626399));
#206007=CARTESIAN_POINT('Ctrl Pts',(-34.0765638445927,-71.0123672528302,
85.3920827438407));
#206008=CARTESIAN_POINT('Ctrl Pts',(-34.0483887293973,-72.2510451174338,
85.7017399515547));
#206009=CARTESIAN_POINT('Ctrl Pts',(-34.0392342437792,-72.6595527561254,
85.7832486538415));
#206010=CARTESIAN_POINT('Ctrl Pts',(-34.0115144072217,-73.8981770415323,
85.9690727208953));
#206011=CARTESIAN_POINT('Ctrl Pts',(-33.992731310687,-74.7351255792752,
86.0130592131825));
#206012=CARTESIAN_POINT('Ctrl Pts',(-33.955371706001,-76.4132424902395,
85.9393476777313));
#206013=CARTESIAN_POINT('Ctrl Pts',(-33.9369789651583,-77.2504069684253,
85.8203857576482));
#206014=CARTESIAN_POINT('Ctrl Pts',(-33.8990573661833,-78.9062080321851,
85.4179625902074));
#206015=CARTESIAN_POINT('Ctrl Pts',(-33.8797302592748,-79.7200570759932,
85.1322576993896));
#206016=CARTESIAN_POINT('Ctrl Pts',(-33.8515355843574,-80.8782039104047,
84.5915279003849));
#206017=CARTESIAN_POINT('Ctrl Pts',(-33.8423466167696,-81.2479763059521,
84.3966627677644));
#206018=CARTESIAN_POINT('Ctrl Pts',(-33.8140691160097,-82.3476574494015,
83.7476140687488));
#206019=CARTESIAN_POINT('Ctrl Pts',(-33.794737390197,-83.0424713065999,
83.2386147866756));
#206020=CARTESIAN_POINT('Ctrl Pts',(-33.7586549670554,-84.2527959019681,
82.1526192558822));
#206021=CARTESIAN_POINT('Ctrl Pts',(-33.7418987501866,-84.7771788972721,
81.590921545649));
#206022=CARTESIAN_POINT('Ctrl Pts',(-33.705709722028,-85.7783300496831,
80.3079062206409));
#206023=CARTESIAN_POINT('Ctrl Pts',(-33.6863603081552,-86.239020039698,
79.5786423791186));
#206024=CARTESIAN_POINT('Ctrl Pts',(-33.6581918465749,-86.810452983774,
78.4373873382913));
#206025=CARTESIAN_POINT('Ctrl Pts',(-33.649048647938,-86.9786866665247,
78.056827364037));
#206026=CARTESIAN_POINT('Ctrl Pts',(-33.6213266156159,-87.4296937897356,
76.8880187355971));
#206027=CARTESIAN_POINT('Ctrl Pts',(-33.6025309162896,-87.6548839720965,
76.0799076396883));
#206028=CARTESIAN_POINT('Ctrl Pts',(-33.5644788453735,-87.9531301665975,
74.3957530123024));
#206029=CARTESIAN_POINT('Ctrl Pts',(-33.5454440944437,-88.0183734434914,
73.5225609866536));
#206030=CARTESIAN_POINT('Ctrl Pts',(-33.5068404281006,-87.9731061851425,
71.7895146102885));
#206031=CARTESIAN_POINT('Ctrl Pts',(-33.4875369900912,-87.8653463592952,
70.9339299399998));
#206032=CARTESIAN_POINT('Ctrl Pts',(-33.455659801239,-87.5436039213937,
69.5247130520752));
#206033=CARTESIAN_POINT('Ctrl Pts',(-33.4427790960703,-87.3749552248436,
68.9635945389235));
#206034=CARTESIAN_POINT('Ctrl Pts',(-33.4102418702305,-86.86065891033,67.5950562137833));
#206035=CARTESIAN_POINT('Ctrl Pts',(-33.3905592101602,-86.4700061757207,
66.8076568513819));
#206036=CARTESIAN_POINT('Ctrl Pts',(-33.3613177814963,-85.7637965985004,
65.6852895329601));
#206037=CARTESIAN_POINT('Ctrl Pts',(-33.3514322408723,-85.5049510413509,
65.3176514742272));
#206038=CARTESIAN_POINT('Ctrl Pts',(-33.3314378047931,-84.9482909039063,
64.608183372074));
#206039=CARTESIAN_POINT('Ctrl Pts',(-33.3213410375762,-84.6505963140764,
64.2670367278378));
#206040=CARTESIAN_POINT('Ctrl Pts',(-33.3112169404745,-84.3357242889639,
63.9421080804773));
#206041=CARTESIAN_POINT('Origin',(-21.6548258024609,-75.,72.98888938658));
#206042=CARTESIAN_POINT('',(-36.4473639743914,-62.9850802944281,77.9529305295057));
#206043=CARTESIAN_POINT('',(-36.1412950695185,-62.9850802944281,77.9529305295057));
#206044=CARTESIAN_POINT('',(-21.6548258024609,-62.9850802944281,77.9529305295057));
#206045=CARTESIAN_POINT('Ctrl Pts',(-34.6333744106366,-62.9850802944281,
77.9529305295057));
#206046=CARTESIAN_POINT('Ctrl Pts',(-34.641014498302,-62.8527275341519,
77.6325851210486));
#206047=CARTESIAN_POINT('Ctrl Pts',(-34.648658393585,-62.7331612112141,
77.3068853604773));
#206048=CARTESIAN_POINT('Ctrl Pts',(-34.6738484033682,-62.3844575639027,
76.2249071551718));
#206049=CARTESIAN_POINT('Ctrl Pts',(-34.6915963640586,-62.2112043754734,
75.452710937918));
#206050=CARTESIAN_POINT('Ctrl Pts',(-34.7263102933167,-62.0093905987928,
73.9048043248658));
#206051=CARTESIAN_POINT('Ctrl Pts',(-34.7431409118205,-61.977935394032,
73.132664809404));
#206052=CARTESIAN_POINT('Ctrl Pts',(-34.7762781355656,-62.04983480117,71.6426752969835));
#206053=CARTESIAN_POINT('Ctrl Pts',(-34.7924822107337,-62.1443232499337,
70.9271815436608));
#206054=CARTESIAN_POINT('Ctrl Pts',(-34.8245199273994,-62.4511959471291,
69.5177537052481));
#206055=CARTESIAN_POINT('Ctrl Pts',(-34.8402934076462,-62.6632973062741,
68.826313272693));
#206056=CARTESIAN_POINT('Ctrl Pts',(-34.8734422301294,-63.2184076373919,
67.4401181719159));
#206057=CARTESIAN_POINT('Ctrl Pts',(-34.8907994054739,-63.5682537311863,
66.7511050425069));
#206058=CARTESIAN_POINT('Ctrl Pts',(-34.9254355268895,-64.3960513698163,
65.4270899112198));
#206059=CARTESIAN_POINT('Ctrl Pts',(-34.9427031652233,-64.8752333752963,
64.7965975180037));
#206060=CARTESIAN_POINT('Ctrl Pts',(-34.9794395177757,-65.9894981678966,
63.5787263238995));
#206061=CARTESIAN_POINT('Ctrl Pts',(-34.9987656114795,-66.6318937865852,
63.0031434729509));
#206062=CARTESIAN_POINT('Ctrl Pts',(-35.0269611300522,-67.6636752702301,
62.2486428642757));
#206063=CARTESIAN_POINT('Ctrl Pts',(-35.0361517023118,-68.0126159078625,
62.0184281755644));
#206064=CARTESIAN_POINT('Ctrl Pts',(-35.0644318262356,-69.1111911860981,
61.3673496406319));
#206065=CARTESIAN_POINT('Ctrl Pts',(-35.0837646191923,-69.891955638007,
61.0036431588981));
#206066=CARTESIAN_POINT('Ctrl Pts',(-35.1199264595699,-71.4301373127408,
60.4649172600748));
#206067=CARTESIAN_POINT('Ctrl Pts',(-35.1367626891198,-72.1786144365612,
60.2753694852728));
#206068=CARTESIAN_POINT('Ctrl Pts',(-35.173037667012,-73.7890534336014,
60.0168418106224));
#206069=CARTESIAN_POINT('Ctrl Pts',(-35.1923839804215,-74.6500948468182,
59.9651423694528));
#206070=CARTESIAN_POINT('Ctrl Pts',(-35.2205570259387,-75.9257643229752,
60.015217496338));
#206071=CARTESIAN_POINT('Ctrl Pts',(-35.2297080309738,-76.3405954064536,
60.0515014817868));
#206072=CARTESIAN_POINT('Ctrl Pts',(-35.2574286342686,-77.5817451575349,
60.2204054800453));
#206073=CARTESIAN_POINT('Ctrl Pts',(-35.2762157314665,-78.3976980433205,
60.4129114044301));
#206074=CARTESIAN_POINT('Ctrl Pts',(-35.3137924594775,-79.9969053829984,
60.9573297758994));
#206075=CARTESIAN_POINT('Ctrl Pts',(-35.3323865848766,-80.7753222813578,
61.3109979284769));
#206076=CARTESIAN_POINT('Ctrl Pts',(-35.3705224384596,-82.2580658579586,
62.1694288005398));
#206077=CARTESIAN_POINT('Ctrl Pts',(-35.3898426630841,-82.9580299352939,
62.6733662304289));
#206078=CARTESIAN_POINT('Ctrl Pts',(-35.4180426924495,-83.9165515457928,
63.5194670507581));
#206079=CARTESIAN_POINT('Ctrl Pts',(-35.4272420436857,-84.2165071128488,
63.811152891912));
#206080=CARTESIAN_POINT('Ctrl Pts',(-35.4555365740011,-85.0883345805226,
64.7448662989507));
#206081=CARTESIAN_POINT('Ctrl Pts',(-35.4748750177734,-85.6110660533947,
65.4295455524948));
#206082=CARTESIAN_POINT('Ctrl Pts',(-35.5114915873723,-86.4781358579965,
66.8343076133079));
#206083=CARTESIAN_POINT('Ctrl Pts',(-35.528786138212,-86.8314863636126,
67.5444043405089));
#206084=CARTESIAN_POINT('Ctrl Pts',(-35.5655511241808,-87.4295650057268,
69.0842497084332));
#206085=CARTESIAN_POINT('Ctrl Pts',(-35.5848757378552,-87.6606854241181,
69.9152347545338));
#206086=CARTESIAN_POINT('Ctrl Pts',(-35.613072463526,-87.8795653599801,
71.1746596303435));
#206087=CARTESIAN_POINT('Ctrl Pts',(-35.6222653382204,-87.9312255737478,
71.5895901507472));
#206088=CARTESIAN_POINT('Ctrl Pts',(-35.650549234005,-88.0277575135514,
72.8630698603536));
#206089=CARTESIAN_POINT('Ctrl Pts',(-35.6698835411671,-88.0075990639256,
73.7241801138767));
#206090=CARTESIAN_POINT('Ctrl Pts',(-35.7061605505144,-87.8078514639825,
75.3470532851727));
#206091=CARTESIAN_POINT('Ctrl Pts',(-35.7231128427644,-87.6443181674053,
76.1070974524996));
#206092=CARTESIAN_POINT('Ctrl Pts',(-35.7595123339326,-87.1585564748513,
77.6696917195567));
#206093=CARTESIAN_POINT('Ctrl Pts',(-35.7788538251116,-86.8221704847922,
78.4639876877875));
#206094=CARTESIAN_POINT('Ctrl Pts',(-35.8070334463051,-86.2101080968332,
79.5848778072634));
#206095=CARTESIAN_POINT('Ctrl Pts',(-35.8161955912507,-85.9929688662903,
79.9407396568493));
#206096=CARTESIAN_POINT('Ctrl Pts',(-35.8439134584175,-85.2901079930823,
80.9771252094763));
#206097=CARTESIAN_POINT('Ctrl Pts',(-35.8626874326064,-84.7555150715976,
81.6218578649759));
#206098=CARTESIAN_POINT('Ctrl Pts',(-35.8995680862153,-83.5789696633293,
82.7908559248002));
#206099=CARTESIAN_POINT('Ctrl Pts',(-35.9175169020216,-82.9414147917895,
83.314159654687));
#206100=CARTESIAN_POINT('Ctrl Pts',(-35.9549652882549,-81.5448404094005,
84.2541220410596));
#206101=CARTESIAN_POINT('Ctrl Pts',(-35.9743054945147,-80.7850554546446,
84.6625154958597));
#206102=CARTESIAN_POINT('Ctrl Pts',(-36.0024867155247,-79.6056918100297,
85.1528231393263));
#206103=CARTESIAN_POINT('Ctrl Pts',(-36.0116516105019,-79.213401698831,
85.2942104870982));
#206104=CARTESIAN_POINT('Ctrl Pts',(-36.0393686733256,-78.0163844616726,
85.6616678334622));
#206105=CARTESIAN_POINT('Ctrl Pts',(-36.0581392624687,-77.1960005555216,
85.8292731567654));
#206106=CARTESIAN_POINT('Ctrl Pts',(-36.0948471111402,-75.55421159348,86.0026489499043));
#206107=CARTESIAN_POINT('Ctrl Pts',(-36.1126358407721,-74.7369291072049,
86.0117880164174));
#206108=CARTESIAN_POINT('Ctrl Pts',(-36.1499133610179,-73.0666734822116,
85.8730912847391));
#206109=CARTESIAN_POINT('Ctrl Pts',(-36.1692576616452,-72.218336304354,
85.7169201557518));
#206110=CARTESIAN_POINT('Ctrl Pts',(-36.1974335686496,-70.9916550333374,
85.3625121108948));
#206111=CARTESIAN_POINT('Ctrl Pts',(-36.2065893919981,-70.5974235216031,
85.227790030333));
#206112=CARTESIAN_POINT('Ctrl Pts',(-36.2343089130728,-69.4330841646863,
84.7663449543757));
#206113=CARTESIAN_POINT('Ctrl Pts',(-36.2530904484636,-68.6873616889725,
84.3840459911954));
#206114=CARTESIAN_POINT('Ctrl Pts',(-36.2903665959047,-67.2764011976082,
83.4794373193744));
#206115=CARTESIAN_POINT('Ctrl Pts',(-36.3086819562941,-66.6148714946546,
82.9586035611532));
#206116=CARTESIAN_POINT('Ctrl Pts',(-36.3465211473052,-65.3868126826264,
81.7824650483401));
#206117=CARTESIAN_POINT('Ctrl Pts',(-36.3658507308723,-64.8260169830175,
81.1270970334503));
#206118=CARTESIAN_POINT('Ctrl Pts',(-36.3940432043561,-64.0953648788812,
80.0785506280071));
#206119=CARTESIAN_POINT('Ctrl Pts',(-36.4032280887483,-63.8732812127073,
79.7246515881299));
#206120=CARTESIAN_POINT('Ctrl Pts',(-36.424041948537,-63.4125683625356,
78.9053348831349));
#206121=CARTESIAN_POINT('Ctrl Pts',(-36.4356882557931,-63.1843405800142,
78.4352182992673));
#206122=CARTESIAN_POINT('Ctrl Pts',(-36.4473639743914,-62.9850802944281,
77.9529305295057));
#206123=CARTESIAN_POINT('Ctrl Pts',(-36.1412950695185,-62.9850802944281,
77.9529305295057));
#206124=CARTESIAN_POINT('Ctrl Pts',(-36.1298525502769,-63.1803591218897,
78.425581614498));
#206125=CARTESIAN_POINT('Ctrl Pts',(-36.1184583697945,-63.4034749546776,
78.886580639856));
#206126=CARTESIAN_POINT('Ctrl Pts',(-36.0979502789426,-63.8572044270931,
79.6980294849889));
#206127=CARTESIAN_POINT('Ctrl Pts',(-36.0887627234557,-64.078500159393,
80.0525495582584));
#206128=CARTESIAN_POINT('Ctrl Pts',(-36.0604875345533,-64.8060087068991,
81.1018877758815));
#206129=CARTESIAN_POINT('Ctrl Pts',(-36.0411567591116,-65.3643328811862,
81.7577039564323));
#206130=CARTESIAN_POINT('Ctrl Pts',(-36.0051415928358,-66.5334898549632,
82.8834150934476));
#206131=CARTESIAN_POINT('Ctrl Pts',(-35.9884531675195,-67.1293477687627,
83.3636796870078));
#206132=CARTESIAN_POINT('Ctrl Pts',(-35.9542340750339,-68.4078798433051,
84.220309833931));
#206133=CARTESIAN_POINT('Ctrl Pts',(-35.9367849374942,-69.0891474589492,
84.5933144326596));
#206134=CARTESIAN_POINT('Ctrl Pts',(-35.9065947947129,-70.3398260948869,
85.1392086252321));
#206135=CARTESIAN_POINT('Ctrl Pts',(-35.8936717610195,-70.8954921615821,
85.3379984834587));
#206136=CARTESIAN_POINT('Ctrl Pts',(-35.8631504303883,-72.2199572693316,
85.7125134739772));
#206137=CARTESIAN_POINT('Ctrl Pts',(-35.8454515742033,-72.9950638305585,
85.8574350415196));
#206138=CARTESIAN_POINT('Ctrl Pts',(-35.8119077179018,-74.4986160864227,
85.999339158326));
#206139=CARTESIAN_POINT('Ctrl Pts',(-35.7961055625979,-75.2231526572785,
86.0070843134678));
#206140=CARTESIAN_POINT('Ctrl Pts',(-35.7629303779634,-76.7135634606904,
85.8985059243922));
#206141=CARTESIAN_POINT('Ctrl Pts',(-35.7455770783725,-77.4760531957894,
85.7741799705351));
#206142=CARTESIAN_POINT('Ctrl Pts',(-35.710886806919,-78.9912201978066,
85.3864273889758));
#206143=CARTESIAN_POINT('Ctrl Pts',(-35.693560322958,-79.7398287285188,
85.1199576918447));
#206144=CARTESIAN_POINT('Ctrl Pts',(-35.6567613892564,-81.240323217721,
84.4256128705099));
#206145=CARTESIAN_POINT('Ctrl Pts',(-35.6374385682394,-81.9833735426707,
83.987652175025));
#206146=CARTESIAN_POINT('Ctrl Pts',(-35.609240444434,-83.0150055342737,
83.2326392252354));
#206147=CARTESIAN_POINT('Ctrl Pts',(-35.6000448628727,-83.3402164835095,
82.969646531436));
#206148=CARTESIAN_POINT('Ctrl Pts',(-35.5717565267856,-84.29350749714,82.1195554590688));
#206149=CARTESIAN_POINT('Ctrl Pts',(-35.5524204684057,-84.8765420593404,
81.4854917354083));
#206150=CARTESIAN_POINT('Ctrl Pts',(-35.5160044028697,-85.8626912887872,
80.1731711400995));
#206151=CARTESIAN_POINT('Ctrl Pts',(-35.4989119626645,-86.275235827812,
79.5066367552329));
#206152=CARTESIAN_POINT('Ctrl Pts',(-35.4623624776624,-87.0104486362849,
78.0376025408581));
#206153=CARTESIAN_POINT('Ctrl Pts',(-35.4430274023172,-87.3182033186538,
77.2317962421226));
#206154=CARTESIAN_POINT('Ctrl Pts',(-35.4148403390291,-87.6535935030626,
75.9989728902198));
#206155=CARTESIAN_POINT('Ctrl Pts',(-35.4056652296747,-87.7436649065816,
75.5913950649829));
#206156=CARTESIAN_POINT('Ctrl Pts',(-35.3779516203089,-87.9546667311608,
74.3575301165006));
#206157=CARTESIAN_POINT('Ctrl Pts',(-35.3591941298354,-88.0157992054867,
73.5232336120756));
#206158=CARTESIAN_POINT('Ctrl Pts',(-35.3231332789316,-87.9783573860045,
71.9013534622564));
#206159=CARTESIAN_POINT('Ctrl Pts',(-35.305943613096,-87.8886388157082,
71.1171279053155));
#206160=CARTESIAN_POINT('Ctrl Pts',(-35.2712619772891,-87.57143980227,69.5895381066747));
#206161=CARTESIAN_POINT('Ctrl Pts',(-35.2538720546943,-87.3472935931955,
68.8487163896592));
#206162=CARTESIAN_POINT('Ctrl Pts',(-35.2245121336728,-86.8517196601871,
67.6182549098334));
#206163=CARTESIAN_POINT('Ctrl Pts',(-35.212363976353,-86.6120863114997,
67.1180779594422));
#206164=CARTESIAN_POINT('Ctrl Pts',(-35.1810619928782,-85.9212762507082,
65.885082061825));
#206165=CARTESIAN_POINT('Ctrl Pts',(-35.161725612669,-85.4279893299815,
65.1789353483755));
#206166=CARTESIAN_POINT('Ctrl Pts',(-35.1252832688943,-84.3586469278054,
63.9318707316406));
#206167=CARTESIAN_POINT('Ctrl Pts',(-35.1081643422314,-83.7959127433042,
63.3844224239668));
#206168=CARTESIAN_POINT('Ctrl Pts',(-35.0715865582653,-82.5189577011011,
62.3490750784855));
#206169=CARTESIAN_POINT('Ctrl Pts',(-35.0522527705251,-81.7984371772448,
61.8748605922018));
#206170=CARTESIAN_POINT('Ctrl Pts',(-35.0240643659055,-80.6668092325737,
61.2815674948093));
#206171=CARTESIAN_POINT('Ctrl Pts',(-35.0148868659841,-80.2881379141312,
61.1057201981099));
#206172=CARTESIAN_POINT('Ctrl Pts',(-34.987174173883,-79.1288382149548,
60.6337712453924));
#206173=CARTESIAN_POINT('Ctrl Pts',(-34.968419872004,-78.3275164411888,
60.3942925768916));
#206174=CARTESIAN_POINT('Ctrl Pts',(-34.932511525472,-76.7423163818132,
60.0825130771705));
#206175=CARTESIAN_POINT('Ctrl Pts',(-34.9154629905747,-75.9638072250017,
60.0011529314397));
#206176=CARTESIAN_POINT('Ctrl Pts',(-34.8809560702276,-74.4114376289477,
59.979331990741));
#206177=CARTESIAN_POINT('Ctrl Pts',(-34.8635905575498,-73.6407223218485,
60.0371575924769));
#206178=CARTESIAN_POINT('Ctrl Pts',(-34.8346132052656,-72.3493295968927,
60.2506430475948));
#206179=CARTESIAN_POINT('Ctrl Pts',(-34.8228253346168,-71.8249137096747,
60.3711319717456));
#206180=CARTESIAN_POINT('Ctrl Pts',(-34.7924331535153,-70.5083867782047,
60.7609136513772));
#206181=CARTESIAN_POINT('Ctrl Pts',(-34.7736616693852,-69.7320391158638,
61.0747568939945));
#206182=CARTESIAN_POINT('Ctrl Pts',(-34.7369083697422,-68.2662767014208,
61.838765999511));
#206183=CARTESIAN_POINT('Ctrl Pts',(-34.7190775380642,-67.5786125791408,
62.2841569611463));
#206184=CARTESIAN_POINT('Ctrl Pts',(-34.681755071938,-66.2623542678585,
63.3248345387022));
#206185=CARTESIAN_POINT('Ctrl Pts',(-34.6624118173452,-65.6420146154581,
63.9242035761149));
#206186=CARTESIAN_POINT('Ctrl Pts',(-34.63423449118,-64.816078613799,64.898079971304));
#206187=CARTESIAN_POINT('Ctrl Pts',(-34.6250762620786,-64.5621204161471,
65.2284691985156));
#206188=CARTESIAN_POINT('Ctrl Pts',(-34.5973573387338,-63.8474596197001,
66.2569088915288));
#206189=CARTESIAN_POINT('Ctrl Pts',(-34.5785786450852,-63.4377788028716,
66.9877441412928));
#206190=CARTESIAN_POINT('Ctrl Pts',(-34.5414527763825,-62.765387999806,
68.5157453771292));
#206191=CARTESIAN_POINT('Ctrl Pts',(-34.5232767236405,-62.5038197776782,
69.3091836367251));
#206192=CARTESIAN_POINT('Ctrl Pts',(-34.4855859796664,-62.1302729106898,
70.9614529881757));
#206193=CARTESIAN_POINT('Ctrl Pts',(-34.4662521462287,-62.0243222102277,
71.8174926686515));
#206194=CARTESIAN_POINT('Ctrl Pts',(-34.4380637884215,-61.9937367843572,
73.0948472448445));
#206195=CARTESIAN_POINT('Ctrl Pts',(-34.4288863722571,-62.0038381402737,
73.5122311710028));
#206196=CARTESIAN_POINT('Ctrl Pts',(-34.4011736473037,-62.0942980487042,
74.7606449122937));
#206197=CARTESIAN_POINT('Ctrl Pts',(-34.3824192329003,-62.2345891096477,
75.5851425473809));
#206198=CARTESIAN_POINT('Ctrl Pts',(-34.3516267721921,-62.5970931805737,
76.922270003251));
#206199=CARTESIAN_POINT('Ctrl Pts',(-34.3395609378567,-62.7748651755682,
77.4441277816481));
#206200=CARTESIAN_POINT('Ctrl Pts',(-34.3273949797549,-62.9850802944281,
77.9529305295057));
#206201=CARTESIAN_POINT('Origin',(-21.6548258024609,-75.,72.98888938658));
#206202=CARTESIAN_POINT('',(-39.5675364832709,-62.9850802944281,77.9529305295057));
#206203=CARTESIAN_POINT('',(-39.5675364832709,-70.0359588570743,60.9739696810081));
#206204=CARTESIAN_POINT('Origin',(-39.5675364832709,-75.,72.98888938658));
#206205=CARTESIAN_POINT('Origin',(-39.5675364832709,-75.,72.98888938658));
#206206=CARTESIAN_POINT('',(-39.3655152556871,-62.9850803327788,77.9529306223294));
#206207=CARTESIAN_POINT('',(-21.6548258024609,-62.9850802944281,77.9529305295057));
#206208=CARTESIAN_POINT('',(-39.378281183842,-62.0210675376173,72.249083919906));
#206209=CARTESIAN_POINT('Ctrl Pts',(-39.3655152559408,-62.985080332779,
77.95293062233));
#206210=CARTESIAN_POINT('Ctrl Pts',(-39.367974326097,-62.6134372726655,
77.0534091840336));
#206211=CARTESIAN_POINT('Ctrl Pts',(-39.3710406973607,-62.3439836733896,
76.1149984769994));
#206212=CARTESIAN_POINT('Ctrl Pts',(-39.3753005433957,-62.0195887932955,
74.1956296276191));
#206213=CARTESIAN_POINT('Ctrl Pts',(-39.376513824047,-61.9656804043715,
73.2207797100456));
#206214=CARTESIAN_POINT('Ctrl Pts',(-39.3782811843755,-62.0210675372952,
72.2490839198886));
#206215=CARTESIAN_POINT('',(-38.9114901702032,-62.0210675376382,72.2490839198538));
#206216=CARTESIAN_POINT('',(-38.9115960243709,-62.0210675372924,72.2490839198855));
#206217=CARTESIAN_POINT('',(-38.6651607695592,-62.9850797267618,77.9529291555314));
#206218=CARTESIAN_POINT('Ctrl Pts',(-38.9114901696398,-62.0210675372996,
72.2490839198104));
#206219=CARTESIAN_POINT('Ctrl Pts',(-38.87002296087,-61.9656824369655,73.2207440507031));
#206220=CARTESIAN_POINT('Ctrl Pts',(-38.8281416219942,-62.0195861640916,
74.1955869480229));
#206221=CARTESIAN_POINT('Ctrl Pts',(-38.7459661857041,-62.3439713077193,
76.1149524347908));
#206222=CARTESIAN_POINT('Ctrl Pts',(-38.7059499709518,-62.6134267199739,
77.0533833312218));
#206223=CARTESIAN_POINT('Ctrl Pts',(-38.6651607695592,-62.9850797267618,
77.9529291555314));
#206224=CARTESIAN_POINT('',(-37.9553013365568,-62.9850802944281,77.9529305295057));
#206225=CARTESIAN_POINT('',(-21.6548258024609,-62.9850802944281,77.9529305295057));
#206226=CARTESIAN_POINT('',(-39.3215010433097,-79.7259927877122,85.0994220373138));
#206227=CARTESIAN_POINT('Ctrl Pts',(-39.321506023786,-79.7261416975021,
85.0993635579381));
#206228=CARTESIAN_POINT('Ctrl Pts',(-39.3113482514596,-80.1554579332872,
84.9318218634802));
#206229=CARTESIAN_POINT('Ctrl Pts',(-39.3011776717826,-80.5755604755536,
84.7415702126412));
#206230=CARTESIAN_POINT('Ctrl Pts',(-39.2807471898218,-81.3908301718727,
84.3187887005437));
#206231=CARTESIAN_POINT('Ctrl Pts',(-39.2705028353935,-81.7855868463675,
84.086868401655));
#206232=CARTESIAN_POINT('Ctrl Pts',(-39.2402664687624,-82.9136640432723,
83.341390069044));
#206233=CARTESIAN_POINT('Ctrl Pts',(-39.2207367675194,-83.6071304006881,
82.7724295103021));
#206234=CARTESIAN_POINT('Ctrl Pts',(-39.187736279067,-84.6541971890334,
81.7152027972093));
#206235=CARTESIAN_POINT('Ctrl Pts',(-39.1744557107486,-85.0423775040713,
81.2655263007179));
#206236=CARTESIAN_POINT('Ctrl Pts',(-39.1419599814079,-85.9149008766984,
80.1026338823808));
#206237=CARTESIAN_POINT('Ctrl Pts',(-39.1231751559109,-86.3617101374352,
79.3647788138448));
#206238=CARTESIAN_POINT('Ctrl Pts',(-39.0850463360107,-87.1024487154548,
77.8126986476469));
#206239=CARTESIAN_POINT('Ctrl Pts',(-39.0656944288797,-87.3947616178232,
77.0024020414012));
#206240=CARTESIAN_POINT('Ctrl Pts',(-39.0374375807919,-87.7069281015113,
75.7651521671601));
#206241=CARTESIAN_POINT('Ctrl Pts',(-39.0282836838252,-87.789387623988,
75.356424408735));
#206242=CARTESIAN_POINT('Ctrl Pts',(-38.9983274833698,-87.9935104378332,
74.0149112619828));
#206243=CARTESIAN_POINT('Ctrl Pts',(-38.9772513454028,-88.0336861114053,
73.0727804455865));
#206244=CARTESIAN_POINT('Ctrl Pts',(-38.9371909475701,-87.9154135641783,
71.276891516979));
#206245=CARTESIAN_POINT('Ctrl Pts',(-38.9184592518008,-87.7739999514192,
70.426903035325));
#206246=CARTESIAN_POINT('Ctrl Pts',(-38.8866396546053,-87.4009417144042,
69.046570325221));
#206247=CARTESIAN_POINT('Ctrl Pts',(-38.8738402023574,-87.2160830328018,
68.5064182412333));
#206248=CARTESIAN_POINT('Ctrl Pts',(-38.8517581241255,-86.8344064686362,
67.5922694312997));
#206249=CARTESIAN_POINT('Ctrl Pts',(-38.842500800169,-86.6537393020338,
67.2124680051155));
#206250=CARTESIAN_POINT('Ctrl Pts',(-38.8061998248951,-85.875068985673,
65.7613622926709));
#206251=CARTESIAN_POINT('Ctrl Pts',(-38.7786800607374,-85.1451132647971,
64.768126542228));
#206252=CARTESIAN_POINT('Ctrl Pts',(-38.7423424310481,-83.9954923090845,
63.5945030620776));
#206253=CARTESIAN_POINT('Ctrl Pts',(-38.7331950830006,-83.6899982218031,
63.311218801858));
#206254=CARTESIAN_POINT('Ctrl Pts',(-38.7037868133542,-82.6714131616104,
62.4538702915295));
#206255=CARTESIAN_POINT('Ctrl Pts',(-38.6832615333122,-81.9111407800835,
61.9402098646618));
#206256=CARTESIAN_POINT('Ctrl Pts',(-38.6437753971098,-80.3443935727869,
61.1071315502257));
#206257=CARTESIAN_POINT('Ctrl Pts',(-38.6250431938578,-79.5473707885441,
60.7798707466158));
#206258=CARTESIAN_POINT('Ctrl Pts',(-38.593322866449,-78.1819243201014,
60.3716252262562));
#206259=CARTESIAN_POINT('Ctrl Pts',(-38.5806266647946,-77.6299494353271,
60.245131674304));
#206260=CARTESIAN_POINT('Ctrl Pts',(-38.5507812147664,-76.3080766280265,
60.031770524167));
#206261=CARTESIAN_POINT('Ctrl Pts',(-38.5339097461974,-75.5351845042424,
59.9769113524817));
#206262=CARTESIAN_POINT('Ctrl Pts',(-38.4986388165814,-73.9454075635035,
60.0060198059474));
#206263=CARTESIAN_POINT('Ctrl Pts',(-38.4802511787274,-73.1320287720359,
60.0978945506683));
#206264=CARTESIAN_POINT('Ctrl Pts',(-38.4435802277085,-71.5127828458182,
60.4373529622181));
#206265=CARTESIAN_POINT('Ctrl Pts',(-38.4252687805447,-70.7114301394952,
60.6880794174666));
#206266=CARTESIAN_POINT('Ctrl Pts',(-38.3908818187426,-69.2903855024502,
61.2885760400576));
#206267=CARTESIAN_POINT('Ctrl Pts',(-38.3750346592167,-68.6643789927797,
61.6153699446988));
#206268=CARTESIAN_POINT('Ctrl Pts',(-38.3502514172104,-67.7158356397337,
62.2132591234165));
#206269=CARTESIAN_POINT('Ctrl Pts',(-38.3411059210818,-67.3745706508539,
62.451997730562));
#206270=CARTESIAN_POINT('Ctrl Pts',(-38.3120645038886,-66.3351145766857,
63.2561560128368));
#206271=CARTESIAN_POINT('Ctrl Pts',(-38.2919120963771,-65.6837250195085,
63.8777237668502));
#206272=CARTESIAN_POINT('Ctrl Pts',(-38.2528138845757,-64.5444767098619,
65.2158174645238));
#206273=CARTESIAN_POINT('Ctrl Pts',(-38.2340811610396,-64.0536021176555,
65.9238349903496));
#206274=CARTESIAN_POINT('Ctrl Pts',(-38.2056320505399,-63.4328818764009,
67.0410306554381));
#206275=CARTESIAN_POINT('Ctrl Pts',(-38.1962609427299,-63.247361092142,
67.4165718556594));
#206276=CARTESIAN_POINT('Ctrl Pts',(-38.1676590872137,-62.7369249334442,
68.5892179736311));
#206277=CARTESIAN_POINT('Ctrl Pts',(-38.1488490860104,-62.4727150568358,
69.4101671134101));
#206278=CARTESIAN_POINT('Ctrl Pts',(-38.1106568670412,-62.1096053559418,
71.0957219055625));
#206279=CARTESIAN_POINT('Ctrl Pts',(-38.0912114977267,-62.0123094454613,
71.9562987720156));
#206280=CARTESIAN_POINT('Ctrl Pts',(-38.0535025268716,-61.9902344102795,
73.6567680186461));
#206281=CARTESIAN_POINT('Ctrl Pts',(-38.0352195326587,-62.0601682096371,
74.4924929792126));
#206282=CARTESIAN_POINT('Ctrl Pts',(-38.0073031348116,-62.2843834657231,
75.7249738972242));
#206283=CARTESIAN_POINT('Ctrl Pts',(-37.9979834780239,-62.3784455771531,
76.13045353721));
#206284=CARTESIAN_POINT('Ctrl Pts',(-37.9774552473509,-62.6286908492328,
77.0142109704468));
#206285=CARTESIAN_POINT('Ctrl Pts',(-37.9663643192439,-62.7934308888043,
77.4890640638799));
#206286=CARTESIAN_POINT('Ctrl Pts',(-37.9553013365568,-62.9850802944281,
77.9529305295057));
#206287=CARTESIAN_POINT('Ctrl Pts',(-39.3215011869246,-79.7258751176041,
85.0994675880042));
#206288=CARTESIAN_POINT('Ctrl Pts',(-39.3236712637677,-78.9367247383293,
85.4074154067982));
#206289=CARTESIAN_POINT('Ctrl Pts',(-39.3262569458996,-78.1193599427749,
85.6374944349639));
#206290=CARTESIAN_POINT('Ctrl Pts',(-39.3301175566084,-76.4652632035647,
85.9328892466976));
#206291=CARTESIAN_POINT('Ctrl Pts',(-39.3314200360406,-75.632920357202,
86.0001740554809));
#206292=CARTESIAN_POINT('Ctrl Pts',(-39.3355204404005,-73.1131187980923,
85.9613804639162));
#206293=CARTESIAN_POINT('Ctrl Pts',(-39.3415199539802,-71.4474475515615,
85.6073365102985));
#206294=CARTESIAN_POINT('Ctrl Pts',(-39.3463525919956,-69.1288448774416,
84.6175275196918));
#206295=CARTESIAN_POINT('Ctrl Pts',(-39.3473555822715,-68.395046064557,
84.2169902570332));
#206296=CARTESIAN_POINT('Ctrl Pts',(-39.3513429793926,-66.6498730320518,
83.0337632759551));
#206297=CARTESIAN_POINT('Ctrl Pts',(-39.3558794304813,-65.7059415961714,
82.1673740340386));
#206298=CARTESIAN_POINT('Ctrl Pts',(-39.3612997924157,-64.1112620960786,
80.2011041664734));
#206299=CARTESIAN_POINT('Ctrl Pts',(-39.3623386810063,-63.4651609951521,
79.114913433967));
#206300=CARTESIAN_POINT('Ctrl Pts',(-39.3655152559408,-62.985080332779,
77.95293062233));
#206301=CARTESIAN_POINT('Origin',(-23.4378585958609,-75.,72.98888938658));
#206302=CARTESIAN_POINT('',(-23.3083467243891,-63.2246325280382,77.8539778944304));
#206303=CARTESIAN_POINT('',(-23.4378585958609,-63.1049274015129,77.9034149284856));
#206304=CARTESIAN_POINT('',(-23.5671968062386,-68.218371728628,84.0797707272727));
#206305=CARTESIAN_POINT('Ctrl Pts',(-23.5672140314447,-68.2183351228444,
84.0798326058898));
#206306=CARTESIAN_POINT('Ctrl Pts',(-23.5673199177301,-68.2102006987572,
84.0748587333312));
#206307=CARTESIAN_POINT('Ctrl Pts',(-23.5674258040155,-68.202071746649,
84.06987591173));
#206308=CARTESIAN_POINT('Ctrl Pts',(-23.5675316903009,-68.1939482861969,
84.0648841531478));
#206309=CARTESIAN_POINT('',(-22.5675364824894,-63.000102062494,73.0394432284656));
#206310=CARTESIAN_POINT('Ctrl Pts',(-23.5671139309305,-68.2185478493422,
84.079473011853));
#206311=CARTESIAN_POINT('Ctrl Pts',(-23.5554441969661,-68.9062950368486,
84.4863247226585));
#206312=CARTESIAN_POINT('Ctrl Pts',(-23.5440549453205,-69.6305093949009,
84.8293747514801));
#206313=CARTESIAN_POINT('Ctrl Pts',(-23.5205294743053,-71.1540214987534,
85.3850651834414));
#206314=CARTESIAN_POINT('Ctrl Pts',(-23.5081796031131,-71.9514883296778,
85.5920974487091));
#206315=CARTESIAN_POINT('Ctrl Pts',(-23.4721296505077,-74.35151918976,85.9772996965807));
#206316=CARTESIAN_POINT('Ctrl Pts',(-23.4493257715468,-75.9787816509572,
85.9346245406171));
#206317=CARTESIAN_POINT('Ctrl Pts',(-23.4007516068439,-79.1437407796599,
85.2427926589473));
#206318=CARTESIAN_POINT('Ctrl Pts',(-23.3776454762801,-80.6572582810957,
84.5970625631179));
#206319=CARTESIAN_POINT('Ctrl Pts',(-23.3403526762986,-82.7109372940715,
83.2069683034375));
#206320=CARTESIAN_POINT('Ctrl Pts',(-23.3274897439032,-83.3662661428184,
82.6607486085139));
#206321=CARTESIAN_POINT('Ctrl Pts',(-23.3030014708831,-84.5258213302876,
81.4799624604339));
#206322=CARTESIAN_POINT('Ctrl Pts',(-23.2913605641575,-85.034784190624,
80.8531966773007));
#206323=CARTESIAN_POINT('Ctrl Pts',(-23.2731488040619,-85.70765912193,79.8406857186429));
#206324=CARTESIAN_POINT('Ctrl Pts',(-23.2669076997059,-85.9180739647768,
79.4879801447709));
#206325=CARTESIAN_POINT('Ctrl Pts',(-23.2363418036893,-86.8645556832143,
77.7111294603388));
#206326=CARTESIAN_POINT('Ctrl Pts',(-23.2132436084908,-87.3467226492629,
76.1605022589695));
#206327=CARTESIAN_POINT('Ctrl Pts',(-23.175941245244,-87.6147143249459,
73.7273574819035));
#206328=CARTESIAN_POINT('Ctrl Pts',(-23.1630923328797,-87.6230646296848,
72.8851889496547));
#206329=CARTESIAN_POINT('Ctrl Pts',(-23.1386272326453,-87.4767343480143,
71.2588084415927));
#206330=CARTESIAN_POINT('Ctrl Pts',(-23.1269905153998,-87.3310985127237,
70.4759290443774));
#206331=CARTESIAN_POINT('Ctrl Pts',(-23.1023462125104,-86.8837716791826,
68.9167373502622));
#206332=CARTESIAN_POINT('Ctrl Pts',(-23.0894884991715,-86.5768021364199,
68.1451374417125));
#206333=CARTESIAN_POINT('Ctrl Pts',(-23.0647799643539,-85.829283593617,
66.7003125165248));
#206334=CARTESIAN_POINT('Ctrl Pts',(-23.0529403525711,-85.3948197790364,
66.0267421448464));
#206335=CARTESIAN_POINT('Ctrl Pts',(-23.0283692983425,-84.3849372613321,
64.7498100788465));
#206336=CARTESIAN_POINT('Ctrl Pts',(-23.0154222549053,-83.8071005077573,
64.1532084285903));
#206337=CARTESIAN_POINT('Ctrl Pts',(-22.99053842165,-82.5722329130375,63.1087924579781));
#206338=CARTESIAN_POINT('Ctrl Pts',(-22.9786497998761,-81.9214231764334,
62.6567224664527));
#206339=CARTESIAN_POINT('Ctrl Pts',(-22.9417990983281,-79.7924045565062,
61.461416929723));
#206340=CARTESIAN_POINT('Ctrl Pts',(-22.9159564408366,-78.2107189619208,
60.9523140322316));
#206341=CARTESIAN_POINT('Ctrl Pts',(-22.8848941253731,-76.1771949820816,
60.7213246443215));
#206342=CARTESIAN_POINT('Ctrl Pts',(-22.8788053233581,-75.7757640352971,
60.695510659312));
#206343=CARTESIAN_POINT('Ctrl Pts',(-22.8601629334115,-74.5656541370941,
60.677377622671));
#206344=CARTESIAN_POINT('Ctrl Pts',(-22.8473408710596,-73.7577827747063,
60.745396728485));
#206345=CARTESIAN_POINT('Ctrl Pts',(-22.8226463499019,-72.1947956389624,
61.0335899700935));
#206346=CARTESIAN_POINT('Ctrl Pts',(-22.8107879232795,-71.4409244896018,
61.2483269085628));
#206347=CARTESIAN_POINT('Ctrl Pts',(-22.7739585650263,-69.2056667543144,
62.1240879218911));
#206348=CARTESIAN_POINT('Ctrl Pts',(-22.7483049277877,-67.8343233531809,
63.0075631318264));
#206349=CARTESIAN_POINT('Ctrl Pts',(-22.6985290046577,-65.5116117864563,
65.258515032746));
#206350=CARTESIAN_POINT('Ctrl Pts',(-22.6726909441823,-64.5903204088739,
66.6031378681104));
#206351=CARTESIAN_POINT('Ctrl Pts',(-22.6412225596302,-63.7954162090267,
68.4717174240335));
#206352=CARTESIAN_POINT('Ctrl Pts',(-22.6347891537382,-63.6522165345406,
68.863354422744));
#206353=CARTESIAN_POINT('Ctrl Pts',(-22.6081787237398,-63.1534172450102,
70.484438895471));
#206354=CARTESIAN_POINT('Ctrl Pts',(-22.5874829697694,-62.9747724558953,
71.7617031373275));
#206355=CARTESIAN_POINT('Ctrl Pts',(-22.5675364824894,-63.000102062494,
73.0394432284656));
#206356=CARTESIAN_POINT('',(-22.5675364829333,-75.6109359992393,84.9729941181988));
#206357=CARTESIAN_POINT('Origin',(-22.5675364832709,-75.,72.98888938658));
#206358=CARTESIAN_POINT('Ctrl Pts',(-22.5675364828275,-75.6109290148012,
84.9733322994732));
#206359=CARTESIAN_POINT('Ctrl Pts',(-22.5821246641341,-75.3281574487842,
85.0023542290885));
#206360=CARTESIAN_POINT('Ctrl Pts',(-22.596630345575,-75.043842888071,85.0212811334549));
#206361=CARTESIAN_POINT('Ctrl Pts',(-22.611072664767,-74.7587116498909,
85.0300127005126));
#206362=CARTESIAN_POINT('Ctrl Pts',(-22.6255527714042,-74.47283438326,85.0387671131816));
#206363=CARTESIAN_POINT('Ctrl Pts',(-22.6399691837917,-74.1861364033111,
85.037272755658));
#206364=CARTESIAN_POINT('Ctrl Pts',(-22.654341190157,-73.8993534342203,
85.0254808020076));
#206365=CARTESIAN_POINT('Ctrl Pts',(-22.6687338767193,-73.6121578067898,
85.013671880655));
#206366=CARTESIAN_POINT('Ctrl Pts',(-22.6830820293738,-73.3248771873067,
84.9915357218143));
#206367=CARTESIAN_POINT('Ctrl Pts',(-22.6974050197305,-73.0382505277424,
84.9590756102511));
#206368=CARTESIAN_POINT('Ctrl Pts',(-22.7117584358991,-72.7510149975009,
84.9265465448435));
#206369=CARTESIAN_POINT('Ctrl Pts',(-22.7260865827536,-72.464436447571,
84.8836496437199));
#206370=CARTESIAN_POINT('Ctrl Pts',(-22.7404089556177,-72.1792549800472,
84.8304404268251));
#206371=CARTESIAN_POINT('Ctrl Pts',(-22.7449598340071,-72.0886396755893,
84.8135334046727));
#206372=CARTESIAN_POINT('Ctrl Pts',(-22.7495101294396,-71.9981653826167,
84.7955856168891));
#206373=CARTESIAN_POINT('Ctrl Pts',(-22.7540604673341,-71.9078557089599,
84.7765999369993));
#206374=CARTESIAN_POINT('Ctrl Pts',(-22.7682603128447,-71.6260341291668,
84.7173529695006));
#206375=CARTESIAN_POINT('Ctrl Pts',(-22.7824601583553,-71.3458242246531,
84.6479966081915));
#206376=CARTESIAN_POINT('Ctrl Pts',(-22.7966600038659,-71.0679483801829,
84.5686364662497));
#206377=CARTESIAN_POINT('Ctrl Pts',(-22.8108441312213,-70.7903801232612,
84.4893641699843));
#206378=CARTESIAN_POINT('Ctrl Pts',(-22.8250282585766,-70.515141007826,
84.4001102585464));
#206379=CARTESIAN_POINT('Ctrl Pts',(-22.8392123859319,-70.2429441245523,
84.3010315317623));
#206380=CARTESIAN_POINT('Ctrl Pts',(-22.853385763729,-69.9709535279384,
84.202027892611));
#206381=CARTESIAN_POINT('Ctrl Pts',(-22.8675591415261,-69.7020007974385,
84.0932143694529));
#206382=CARTESIAN_POINT('Ctrl Pts',(-22.8817325193231,-69.4367868456689,
83.9747983265722));
#206383=CARTESIAN_POINT('Ctrl Pts',(-22.8958952491312,-69.1717721403508,
83.8564712457396));
#206384=CARTESIAN_POINT('Ctrl Pts',(-22.9100579789394,-68.9104908376335,
83.7285561304041));
#206385=CARTESIAN_POINT('Ctrl Pts',(-22.9242207087475,-68.653628106899,
83.591309932742));
#206386=CARTESIAN_POINT('Ctrl Pts',(-22.938372891472,-68.3969566636294,
83.4541659432794));
#206387=CARTESIAN_POINT('Ctrl Pts',(-22.9525250741966,-68.144697447945,
83.3077048435254));
#206388=CARTESIAN_POINT('Ctrl Pts',(-22.9666772569212,-67.8975164005641,
83.1522319476065));
#206389=CARTESIAN_POINT('Ctrl Pts',(-22.9808147545176,-67.6505918426178,
82.9969203794091));
#206390=CARTESIAN_POINT('Ctrl Pts',(-22.9949522521141,-67.4087351462392,
82.8326158057185));
#206391=CARTESIAN_POINT('Ctrl Pts',(-23.0090897497105,-67.1725890602893,
82.6596701102742));
#206392=CARTESIAN_POINT('Ctrl Pts',(-23.0232178305834,-66.9366002668442,
82.486839610733));
#206393=CARTESIAN_POINT('Ctrl Pts',(-23.0373459114563,-66.7063146993105,
82.3053796080079));
#206394=CARTESIAN_POINT('Ctrl Pts',(-23.0514739923292,-66.4823493669846,
82.1156872009453));
#206395=CARTESIAN_POINT('Ctrl Pts',(-23.0655889575852,-66.2585919499107,
81.9261708923182));
#206396=CARTESIAN_POINT('Ctrl Pts',(-23.0797039228413,-66.041143249399,
81.7284375853738));
#206397=CARTESIAN_POINT('Ctrl Pts',(-23.0938188880973,-65.830590911148,
81.5229273256862));
#206398=CARTESIAN_POINT('Ctrl Pts',(-23.1038933836672,-65.6803100878887,
81.3762452642536));
#206399=CARTESIAN_POINT('Ctrl Pts',(-23.1139678792372,-65.5335419290588,
81.2256022909387));
#206400=CARTESIAN_POINT('Ctrl Pts',(-23.1240423748071,-65.3904905950289,
81.0711715801781));
#206401=CARTESIAN_POINT('Ctrl Pts',(-23.1381651212176,-65.1899567121992,
80.854685727271));
#206402=CARTESIAN_POINT('Ctrl Pts',(-23.1522876470479,-64.9967312179457,
80.6307580746604));
#206403=CARTESIAN_POINT('Ctrl Pts',(-23.1663998896931,-64.8113536809775,
80.3998921770478));
#206404=CARTESIAN_POINT('Ctrl Pts',(-23.180471970665,-64.62650370524,80.1696832948376));
#206405=CARTESIAN_POINT('Ctrl Pts',(-23.1945338268978,-64.4494572724507,
79.9325757540484));
#206406=CARTESIAN_POINT('Ctrl Pts',(-23.2085754814533,-64.2807160422135,
79.6891085031234));
#206407=CARTESIAN_POINT('Ctrl Pts',(-23.2225931230921,-64.1122633797579,
79.4460576104554));
#206408=CARTESIAN_POINT('Ctrl Pts',(-23.2365906320891,-63.9520877249764,
79.1966688991191));
#206409=CARTESIAN_POINT('Ctrl Pts',(-23.2505580826038,-63.8006520861989,
78.9415158489573));
#206410=CARTESIAN_POINT('Ctrl Pts',(-23.2644919766452,-63.649580268003,
78.6869757980333));
#206411=CARTESIAN_POINT('Ctrl Pts',(-23.2783959564603,-63.5072066914697,
78.426699247846));
#206412=CARTESIAN_POINT('Ctrl Pts',(-23.2922601675768,-63.3739524299285,
78.1612901952514));
#206413=CARTESIAN_POINT('Ctrl Pts',(-23.2975737953982,-63.3228811107241,
78.059568942302));
#206414=CARTESIAN_POINT('Ctrl Pts',(-23.3028815815994,-63.2731489095241,
77.9570941250166));
#206415=CARTESIAN_POINT('Ctrl Pts',(-23.3081829713997,-63.2247779436,77.8539010146614));
#206416=CARTESIAN_POINT('Origin',(-54.462516693425,-83.3223805071439,69.5544896765311));
#206417=CARTESIAN_POINT('',(-55.3469857987243,-91.723644464318,66.083453584911));
#206418=CARTESIAN_POINT('',(-55.5509564659454,-91.7236201228015,66.0833946695129));
#206419=CARTESIAN_POINT('',(-54.462516693425,-91.723644464317,66.0834535849087));
#206420=CARTESIAN_POINT('',(-55.3469876474783,-91.7236667394131,66.0835074998375));
#206421=CARTESIAN_POINT('Ctrl Pts',(-55.3469857987243,-91.7236444643189,
66.0834535849133));
#206422=CARTESIAN_POINT('Ctrl Pts',(-55.346986520562,-91.7236531615995,
66.0834746357314));
#206423=CARTESIAN_POINT('Ctrl Pts',(-55.34698692564,-91.723658042266,66.0834864489593));
#206424=CARTESIAN_POINT('Ctrl Pts',(-55.3469876474783,-91.7236667394131,
66.0835074998375));
#206425=CARTESIAN_POINT('',(-55.5974859706232,-91.412754510303,73.6987840815407));
#206426=CARTESIAN_POINT('Ctrl Pts',(-55.5958816852329,-91.4127370632666,
73.6988181411009));
#206427=CARTESIAN_POINT('Ctrl Pts',(-55.5642543225697,-91.8629650956877,
72.819904863597));
#206428=CARTESIAN_POINT('Ctrl Pts',(-55.5337095641794,-92.1669780783263,
71.8734645115866));
#206429=CARTESIAN_POINT('Ctrl Pts',(-55.4920076933008,-92.3608742713118,
70.5747597609729));
#206430=CARTESIAN_POINT('Ctrl Pts',(-55.4815921437647,-92.3916148160222,
70.2504131744611));
#206431=CARTESIAN_POINT('Ctrl Pts',(-55.4607410660172,-92.4182954809193,
69.5965855223249));
#206432=CARTESIAN_POINT('Ctrl Pts',(-55.4503222021789,-92.4138665426036,
69.2675652529914));
#206433=CARTESIAN_POINT('Ctrl Pts',(-55.4246589713448,-92.3587245966684,
68.4543773063775));
#206434=CARTESIAN_POINT('Ctrl Pts',(-55.409556102247,-92.2869555829917,
67.9726706635948));
#206435=CARTESIAN_POINT('Ctrl Pts',(-55.3785950880418,-92.0647860076726,
67.0155987805646));
#206436=CARTESIAN_POINT('Ctrl Pts',(-55.3627155406804,-91.9131659682807,
66.5421780378772));
#206437=CARTESIAN_POINT('Ctrl Pts',(-55.3469876474783,-91.7236667394131,
66.0835074998375));
#206438=CARTESIAN_POINT('',(-55.7997963168797,-91.4127793742771,73.6987355424395));
#206439=CARTESIAN_POINT('',(-55.7986426798444,-91.4127669427988,73.6987598112127));
#206440=CARTESIAN_POINT('Ctrl Pts',(-55.8013975426224,-91.412796628927,
73.698701857855));
#206441=CARTESIAN_POINT('Ctrl Pts',(-55.7703307595378,-91.8629858380135,
72.8198332392404));
#206442=CARTESIAN_POINT('Ctrl Pts',(-55.738609114948,-92.1669747337267,
71.873445907533));
#206443=CARTESIAN_POINT('Ctrl Pts',(-55.6969348134739,-92.3608675733566,
70.5748181414705));
#206444=CARTESIAN_POINT('Ctrl Pts',(-55.6866939433116,-92.391610150729,
70.250473608271));
#206445=CARTESIAN_POINT('Ctrl Pts',(-55.6660029351568,-92.4182926717337,
69.596708773076));
#206446=CARTESIAN_POINT('Ctrl Pts',(-55.6555661301364,-92.4138699937926,
69.2677545658029));
#206447=CARTESIAN_POINT('Ctrl Pts',(-55.6294909009479,-92.3587621242832,
68.4547261711261));
#206448=CARTESIAN_POINT('Ctrl Pts',(-55.6137725475604,-92.2870277037053,
67.9731075839917));
#206449=CARTESIAN_POINT('Ctrl Pts',(-55.5823353923309,-92.0648910629054,
67.0159225655132));
#206450=CARTESIAN_POINT('Ctrl Pts',(-55.5667469045371,-91.9132233140617,
66.542308496053));
#206451=CARTESIAN_POINT('Ctrl Pts',(-55.5509584931268,-91.7236444643153,
66.0834535849044));
#206452=CARTESIAN_POINT('Origin',(-54.462516693425,-83.3223805071439,69.5544896765311));
#206453=CARTESIAN_POINT('',(-53.7366673713217,-91.723644464317,66.0834535849087));
#206454=CARTESIAN_POINT('Ctrl Pts',(-55.5509564659454,-91.7236201228015,
66.0833946695129));
#206455=CARTESIAN_POINT('Ctrl Pts',(-55.5253406144712,-91.4160335965772,
65.3389298524642));
#206456=CARTESIAN_POINT('Ctrl Pts',(-55.499177208642,-91.0108624303868,
64.6386582185305));
#206457=CARTESIAN_POINT('Ctrl Pts',(-55.4649203412003,-90.3546999993681,
63.7883894770221));
#206458=CARTESIAN_POINT('Ctrl Pts',(-55.4564180486514,-90.1813120932266,
63.5831843472978));
#206459=CARTESIAN_POINT('Ctrl Pts',(-55.4139500320902,-89.2736657850213,
62.6007636815008));
#206460=CARTESIAN_POINT('Ctrl Pts',(-55.3792856629007,-88.4153855626199,
61.9496622562324));
#206461=CARTESIAN_POINT('Ctrl Pts',(-55.3295877163154,-87.0236837526852,
61.2373934801853));
#206462=CARTESIAN_POINT('Ctrl Pts',(-55.3139307707429,-86.5659575586731,
61.0484365270062));
#206463=CARTESIAN_POINT('Ctrl Pts',(-55.2817007715712,-85.6100419548281,
60.7422595286418));
#206464=CARTESIAN_POINT('Ctrl Pts',(-55.2651677518206,-85.1127393687324,
60.6279334855877));
#206465=CARTESIAN_POINT('Ctrl Pts',(-55.2318058404901,-84.0844658784889,
60.4809698156442));
#206466=CARTESIAN_POINT('Ctrl Pts',(-55.2151595260833,-83.5549019378558,
60.4519914605089));
#206467=CARTESIAN_POINT('Ctrl Pts',(-55.1888140433165,-82.7288173444309,
60.4789553904715));
#206468=CARTESIAN_POINT('Ctrl Pts',(-55.1792958474904,-82.432457690611,
60.503209361488));
#206469=CARTESIAN_POINT('Ctrl Pts',(-55.1508190163822,-81.5555431189953,
60.6184660617054));
#206470=CARTESIAN_POINT('Ctrl Pts',(-55.1318383003285,-80.9820421247767,
60.7512479253814));
#206471=CARTESIAN_POINT('Ctrl Pts',(-55.0961446844521,-79.9156960526322,
61.1097895713274));
#206472=CARTESIAN_POINT('Ctrl Pts',(-55.0791754766682,-79.4222373340945,
61.3260426781999));
#206473=CARTESIAN_POINT('Ctrl Pts',(-55.0438935942482,-78.45655296532,61.8557352858212));
#206474=CARTESIAN_POINT('Ctrl Pts',(-55.0256364353789,-77.9885983572908,
62.1722223704164));
#206475=CARTESIAN_POINT('Ctrl Pts',(-54.9915987477152,-77.1614187804716,
62.8516079108152));
#206476=CARTESIAN_POINT('Ctrl Pts',(-54.975718254108,-76.7974323150567,
63.2053850855324));
#206477=CARTESIAN_POINT('Ctrl Pts',(-54.9403850939478,-76.0674404738522,
64.0443477157309));
#206478=CARTESIAN_POINT('Ctrl Pts',(-54.9208907207808,-75.7166775474428,
64.5396028529349));
#206479=CARTESIAN_POINT('Ctrl Pts',(-54.8839584790557,-75.1452993913132,
65.5458567131022));
#206480=CARTESIAN_POINT('Ctrl Pts',(-54.8667561360868,-74.9170969844313,
66.0494924928167));
#206481=CARTESIAN_POINT('Ctrl Pts',(-54.83998383377,-74.6389915050204,66.8497939573887));
#206482=CARTESIAN_POINT('Ctrl Pts',(-54.8306045323765,-74.5556733575306,
67.1334428927245));
#206483=CARTESIAN_POINT('Ctrl Pts',(-54.8021658342044,-74.3464359145047,
67.9998759261224));
#206484=CARTESIAN_POINT('Ctrl Pts',(-54.7830927686022,-74.2638476955701,
68.5914704138563));
#206485=CARTESIAN_POINT('Ctrl Pts',(-54.7469068017329,-74.2172592799442,
69.7425478357616));
#206486=CARTESIAN_POINT('Ctrl Pts',(-54.7295252927433,-74.2458093029776,
70.2991043775261));
#206487=CARTESIAN_POINT('Ctrl Pts',(-54.6965489919458,-74.3938205201781,
71.3274016364934));
#206488=CARTESIAN_POINT('Ctrl Pts',(-54.6810877967896,-74.5005601325604,
71.7990126971426));
#206489=CARTESIAN_POINT('Ctrl Pts',(-54.6493649564325,-74.7992884554055,
72.7572393588683));
#206490=CARTESIAN_POINT('Ctrl Pts',(-54.633222982179,-74.9967973872929,
73.2403241082785));
#206491=CARTESIAN_POINT('Ctrl Pts',(-54.5991420837953,-75.4918730210743,
74.2053133978508));
#206492=CARTESIAN_POINT('Ctrl Pts',(-54.5812202360521,-75.7952380768797,
74.6817818149948));
#206493=CARTESIAN_POINT('Ctrl Pts',(-54.5453238306149,-76.4884066377811,
75.5750969417076));
#206494=CARTESIAN_POINT('Ctrl Pts',(-54.5277297748132,-76.8772124124529,
75.9896059893803));
#206495=CARTESIAN_POINT('Ctrl Pts',(-54.4819257350201,-77.9740545973449,
76.9591547834969));
#206496=CARTESIAN_POINT('Ctrl Pts',(-54.4532575477271,-78.7302245928105,
77.4504226526004));
#206497=CARTESIAN_POINT('Ctrl Pts',(-54.4107330167955,-79.9661825106565,
78.0149052710252));
#206498=CARTESIAN_POINT('Ctrl Pts',(-54.3964014837232,-80.4003698580541,
78.1744984640816));
#206499=CARTESIAN_POINT('Ctrl Pts',(-54.3591923632934,-81.5395675299457,
78.497215353792));
#206500=CARTESIAN_POINT('Ctrl Pts',(-54.3360840119932,-82.2553141229639,
78.6105448520134));
#206501=CARTESIAN_POINT('Ctrl Pts',(-54.2946909823775,-83.5740771167809,
78.6607025923809));
#206502=CARTESIAN_POINT('Ctrl Pts',(-54.2761788315971,-84.172040314975,
78.6244701487551));
#206503=CARTESIAN_POINT('Ctrl Pts',(-54.2388429635918,-85.3389900226743,
78.4372802732549));
#206504=CARTESIAN_POINT('Ctrl Pts',(-54.2201325490364,-85.9056061561151,
78.289341054598));
#206505=CARTESIAN_POINT('Ctrl Pts',(-54.1869301714564,-86.8954795985849,
77.9260696013056));
#206506=CARTESIAN_POINT('Ctrl Pts',(-54.1723247323716,-87.3236339645411,
77.7300851767745));
#206507=CARTESIAN_POINT('Ctrl Pts',(-54.1396768312147,-88.2308002103648,
77.2264331940259));
#206508=CARTESIAN_POINT('Ctrl Pts',(-54.1215896175882,-88.700016029907,
76.9051579967057));
#206509=CARTESIAN_POINT('Ctrl Pts',(-54.0855118501413,-89.570195644652,
76.1811678713697));
#206510=CARTESIAN_POINT('Ctrl Pts',(-54.0679007931629,-89.9696053805803,
75.7804403591979));
#206511=CARTESIAN_POINT('Ctrl Pts',(-54.0318246827696,-90.699775972651,
74.8969280704418));
#206512=CARTESIAN_POINT('Ctrl Pts',(-54.0133105817151,-91.0264078359865,
74.4140740692207));
#206513=CARTESIAN_POINT('Ctrl Pts',(-53.9563753481728,-91.8772605937634,
72.8523420103975));
#206514=CARTESIAN_POINT('Ctrl Pts',(-53.9193773143486,-92.2366885164993,
71.6985282926277));
#206515=CARTESIAN_POINT('Ctrl Pts',(-53.8422853477732,-92.4884677919132,
69.3122004932929));
#206516=CARTESIAN_POINT('Ctrl Pts',(-53.8049835202226,-92.3760370261865,
68.1028845572067));
#206517=CARTESIAN_POINT('Ctrl Pts',(-53.7563177440248,-91.9434278986667,
66.6559697698948));
#206518=CARTESIAN_POINT('Ctrl Pts',(-53.7464297999027,-91.840622165608,
66.3665853414526));
#206519=CARTESIAN_POINT('Ctrl Pts',(-53.7366673713217,-91.723644464317,
66.0834535849086));
#206520=CARTESIAN_POINT('',(-53.5332787937082,-91.723644464317,66.0834535849087));
#206521=CARTESIAN_POINT('',(-54.462516693425,-91.723644464317,66.0834535849087));
#206522=CARTESIAN_POINT('Ctrl Pts',(-53.5332787937083,-91.723644464317,
66.0834535849087));
#206523=CARTESIAN_POINT('Ctrl Pts',(-53.5657195167862,-92.1151475890021,
67.0310441612429));
#206524=CARTESIAN_POINT('Ctrl Pts',(-53.5973634442256,-92.3439610858943,
68.0391740587059));
#206525=CARTESIAN_POINT('Ctrl Pts',(-53.6681363979854,-92.4634382006625,
70.255572182143));
#206526=CARTESIAN_POINT('Ctrl Pts',(-53.7048128836741,-92.2928176317638,
71.4470291134669));
#206527=CARTESIAN_POINT('Ctrl Pts',(-53.7523402620046,-91.7996496083399,
72.8486549360197));
#206528=CARTESIAN_POINT('Ctrl Pts',(-53.7617426504722,-91.688776709542,
73.1208650366088));
#206529=CARTESIAN_POINT('Ctrl Pts',(-53.786786451322,-91.3554824097816,
73.8376344762896));
#206530=CARTESIAN_POINT('Ctrl Pts',(-53.8022949064406,-91.1094803549804,
74.2701164367684));
#206531=CARTESIAN_POINT('Ctrl Pts',(-53.8370000681781,-90.4915686602744,
75.1750728200328));
#206532=CARTESIAN_POINT('Ctrl Pts',(-53.8562507375944,-90.1056750278917,
75.6352062660166));
#206533=CARTESIAN_POINT('Ctrl Pts',(-53.8946704780553,-89.2476479911463,
76.4741486924331));
#206534=CARTESIAN_POINT('Ctrl Pts',(-53.9134537974272,-88.7773537289431,
76.8506354911319));
#206535=CARTESIAN_POINT('Ctrl Pts',(-53.9611704438665,-87.5172814248607,
77.6689760138519));
#206536=CARTESIAN_POINT('Ctrl Pts',(-53.9903650904549,-86.6923511147316,
78.0448008327604));
#206537=CARTESIAN_POINT('Ctrl Pts',(-54.0282062972691,-85.544557337223,
78.373603744593));
#206538=CARTESIAN_POINT('Ctrl Pts',(-54.0374535786892,-85.2597131482222,
78.4405227968045));
#206539=CARTESIAN_POINT('Ctrl Pts',(-54.0785753892556,-83.9888409347452,
78.6750690874694));
#206540=CARTESIAN_POINT('Ctrl Pts',(-54.1109468515645,-82.9823063063651,
78.6930609778407));
#206541=CARTESIAN_POINT('Ctrl Pts',(-54.1802667378603,-80.8218350429073,
78.3737049174265));
#206542=CARTESIAN_POINT('Ctrl Pts',(-54.2185359795977,-79.6955562779002,
77.9733633739001));
#206543=CARTESIAN_POINT('Ctrl Pts',(-54.2745230928638,-78.1805513773695,
77.0728314772297));
#206544=CARTESIAN_POINT('Ctrl Pts',(-54.2928997770395,-77.7127025180204,
76.7305175286025));
#206545=CARTESIAN_POINT('Ctrl Pts',(-54.32985904433,-76.8563102293101,75.9686688065897));
#206546=CARTESIAN_POINT('Ctrl Pts',(-54.348232801788,-76.4683492925215,
75.55232514257));
#206547=CARTESIAN_POINT('Ctrl Pts',(-54.3843160526939,-75.7754913847371,
74.6530862583423));
#206548=CARTESIAN_POINT('Ctrl Pts',(-54.4022512089587,-75.472048291573,
74.172227659856));
#206549=CARTESIAN_POINT('Ctrl Pts',(-54.437648539979,-74.9736500514926,
73.1895548373869));
#206550=CARTESIAN_POINT('Ctrl Pts',(-54.4549919408042,-74.7743974936499,
72.6924811395345));
#206551=CARTESIAN_POINT('Ctrl Pts',(-54.4875469135902,-74.479453168947,
71.715164396541));
#206552=CARTESIAN_POINT('Ctrl Pts',(-54.5028358478436,-74.3765284857388,
71.2390119239194));
#206553=CARTESIAN_POINT('Ctrl Pts',(-54.5349881372755,-74.2429215168278,
70.2378493047272));
#206554=CARTESIAN_POINT('Ctrl Pts',(-54.5518339283031,-74.2186352695932,
69.7137693766174));
#206555=CARTESIAN_POINT('Ctrl Pts',(-54.5878262127692,-74.2634625619525,
68.5950860467173));
#206556=CARTESIAN_POINT('Ctrl Pts',(-54.6065435845373,-74.3458180137023,
68.0034318408713));
#206557=CARTESIAN_POINT('Ctrl Pts',(-54.6347501469436,-74.5547303361902,
67.1368578406274));
#206558=CARTESIAN_POINT('Ctrl Pts',(-54.6441345970218,-74.6379430599501,
66.8531607831728));
#206559=CARTESIAN_POINT('Ctrl Pts',(-54.6711606893686,-74.9153107845357,
66.0539869969008));
#206560=CARTESIAN_POINT('Ctrl Pts',(-54.6889164174018,-75.1426642602809,
65.5514169729881));
#206561=CARTESIAN_POINT('Ctrl Pts',(-54.725247238577,-75.7086005862016,
64.5528422799759));
#206562=CARTESIAN_POINT('Ctrl Pts',(-54.7438770726153,-76.0536243028582,
64.0634688125614));
#206563=CARTESIAN_POINT('Ctrl Pts',(-54.7788210658079,-76.7728794956045,
63.231027367026));
#206564=CARTESIAN_POINT('Ctrl Pts',(-54.7949554163308,-77.1326060662042,
62.8785008434476));
#206565=CARTESIAN_POINT('Ctrl Pts',(-54.830365641688,-77.9899850958522,
62.1674548966518));
#206566=CARTESIAN_POINT('Ctrl Pts',(-54.84930305249,-78.4984758404145,61.8257982800024));
#206567=CARTESIAN_POINT('Ctrl Pts',(-54.8847262838848,-79.4888465396703,
61.2964396989534));
#206568=CARTESIAN_POINT('Ctrl Pts',(-54.9010447988734,-79.9598814487711,
61.0936998418295));
#206569=CARTESIAN_POINT('Ctrl Pts',(-54.9360087087864,-81.0022565798859,
60.7459210379695));
#206570=CARTESIAN_POINT('Ctrl Pts',(-54.9542468382506,-81.5757330457078,
60.6145186004252));
#206571=CARTESIAN_POINT('Ctrl Pts',(-54.9819564822361,-82.4524902379245,
60.5012653520307));
#206572=CARTESIAN_POINT('Ctrl Pts',(-54.9913056516659,-82.7488018448857,
60.4776738507298));
#206573=CARTESIAN_POINT('Ctrl Pts',(-55.0176841874367,-83.5815196074021,
60.4523192208539));
#206574=CARTESIAN_POINT('Ctrl Pts',(-55.0348210866761,-84.1177017372103,
60.48342958032));
#206575=CARTESIAN_POINT('Ctrl Pts',(-55.0705671886528,-85.2440162653569,
60.6494582951026));
#206576=CARTESIAN_POINT('Ctrl Pts',(-55.089200938564,-85.8298129690779,
60.7963474225708));
#206577=CARTESIAN_POINT('Ctrl Pts',(-55.1231960096561,-86.8443013749974,
61.1609466417267));
#206578=CARTESIAN_POINT('Ctrl Pts',(-55.1383443905106,-87.278530347074,
61.3566628218977));
#206579=CARTESIAN_POINT('Ctrl Pts',(-55.1777226776238,-88.3692955365197,
61.9552272237522));
#206580=CARTESIAN_POINT('Ctrl Pts',(-55.2013284446643,-88.9935284884356,
62.4089859390303));
#206581=CARTESIAN_POINT('Ctrl Pts',(-55.2455894770798,-90.0144103447644,
63.3700487284535));
#206582=CARTESIAN_POINT('Ctrl Pts',(-55.2658400124447,-90.4289847484269,
63.8512660279433));
#206583=CARTESIAN_POINT('Ctrl Pts',(-55.3061069537296,-91.1617894580098,
64.9071414971543));
#206584=CARTESIAN_POINT('Ctrl Pts',(-55.3263288657872,-91.4747531335122,
65.4810392879816));
#206585=CARTESIAN_POINT('Ctrl Pts',(-55.3469857987243,-91.7236444643189,
66.0834535849133));
#206586=CARTESIAN_POINT('Origin',(-54.462516693425,-83.3223805071439,69.5544896765311));
#206587=CARTESIAN_POINT('',(-51.719048945098,-91.723644464317,66.0834535849086));
#206588=CARTESIAN_POINT('',(-51.9229031371334,-91.723644464317,66.0834535849087));
#206589=CARTESIAN_POINT('',(-54.462516693425,-91.723644464317,66.0834535849087));
#206590=CARTESIAN_POINT('Ctrl Pts',(-51.719048945098,-91.723644464317,66.0834535849086));
#206591=CARTESIAN_POINT('Ctrl Pts',(-51.7280460948346,-91.8334313256315,
66.3491806982507));
#206592=CARTESIAN_POINT('Ctrl Pts',(-51.7370778457283,-91.9306157095051,
66.6201278091617));
#206593=CARTESIAN_POINT('Ctrl Pts',(-51.7649159822995,-92.188226276821,
67.462244733628));
#206594=CARTESIAN_POINT('Ctrl Pts',(-51.7839197817191,-92.3057665340331,
68.0446929603594));
#206595=CARTESIAN_POINT('Ctrl Pts',(-51.8173273069588,-92.413046642744,
69.0991564993682));
#206596=CARTESIAN_POINT('Ctrl Pts',(-51.8318573841923,-92.4244346559946,
69.566843120823));
#206597=CARTESIAN_POINT('Ctrl Pts',(-51.864463419202,-92.3699133844991,
70.6004128247021));
#206598=CARTESIAN_POINT('Ctrl Pts',(-51.8825878956557,-92.2869251622951,
71.1634435721421));
#206599=CARTESIAN_POINT('Ctrl Pts',(-51.9187219781746,-92.0178233248715,
72.2631931788643));
#206600=CARTESIAN_POINT('Ctrl Pts',(-51.9363519248122,-91.832936819118,
72.7976724134826));
#206601=CARTESIAN_POINT('Ctrl Pts',(-51.9724938200408,-91.3590176540957,
73.8417798068455));
#206602=CARTESIAN_POINT('Ctrl Pts',(-51.9910560470183,-91.0679569868936,
74.3476539661278));
#206603=CARTESIAN_POINT('Ctrl Pts',(-52.0390763812932,-90.1999704828028,
75.5683310544183));
#206604=CARTESIAN_POINT('Ctrl Pts',(-52.0675003869634,-89.5597247088562,
76.230047794052));
#206605=CARTESIAN_POINT('Ctrl Pts',(-52.1125565717711,-88.4385887425772,
77.0842789749737));
#206606=CARTESIAN_POINT('Ctrl Pts',(-52.1285174301459,-88.0219464583443,
77.3511164603119));
#206607=CARTESIAN_POINT('Ctrl Pts',(-52.1536914625528,-87.3265022713049,
77.7204228076833));
#206608=CARTESIAN_POINT('Ctrl Pts',(-52.1629664133898,-87.0607943022757,
77.8454316115363));
#206609=CARTESIAN_POINT('Ctrl Pts',(-52.2097874835752,-85.6932541589566,
78.4096942627259));
#206610=CARTESIAN_POINT('Ctrl Pts',(-52.2480366809078,-84.5190110283137,
78.6431507396296));
#206611=CARTESIAN_POINT('Ctrl Pts',(-52.3040609088526,-82.7530810212965,
78.6452356797767));
#206612=CARTESIAN_POINT('Ctrl Pts',(-52.3224844475056,-82.1743185992721,
78.5904019278873));
#206613=CARTESIAN_POINT('Ctrl Pts',(-52.3594985379059,-81.0469595321664,
78.3734708628753));
#206614=CARTESIAN_POINT('Ctrl Pts',(-52.377865835396,-80.5004550770134,
78.2140925191472));
#206615=CARTESIAN_POINT('Ctrl Pts',(-52.4140204960253,-79.4433398869284,
77.7950159961957));
#206616=CARTESIAN_POINT('Ctrl Pts',(-52.4320383530452,-78.9351414315279,
77.5360534123711));
#206617=CARTESIAN_POINT('Ctrl Pts',(-52.4673467810817,-78.0085664234786,
76.9485093849778));
#206618=CARTESIAN_POINT('Ctrl Pts',(-52.4845077086776,-77.588112981137,
76.6274189899154));
#206619=CARTESIAN_POINT('Ctrl Pts',(-52.5178166694003,-76.8176849777865,
75.9249704882126));
#206620=CARTESIAN_POINT('Ctrl Pts',(-52.5340251926803,-76.4675761418157,
75.546630457846));
#206621=CARTESIAN_POINT('Ctrl Pts',(-52.5660246163178,-75.8522482829902,
74.7567348376003));
#206622=CARTESIAN_POINT('Ctrl Pts',(-52.5817363415229,-75.5844589623201,
74.3493612567707));
#206623=CARTESIAN_POINT('Ctrl Pts',(-52.6167570837017,-75.0627908399065,
73.3972988686499));
#206624=CARTESIAN_POINT('Ctrl Pts',(-52.6356418548615,-74.827614268292,
72.8449236210996));
#206625=CARTESIAN_POINT('Ctrl Pts',(-52.6640308229148,-74.5603214710058,
71.9922158021785));
#206626=CARTESIAN_POINT('Ctrl Pts',(-52.6734291289318,-74.4858967729631,
71.706869928634));
#206627=CARTESIAN_POINT('Ctrl Pts',(-52.7002855574127,-74.3142335361895,
70.8874847239771));
#206628=CARTESIAN_POINT('Ctrl Pts',(-52.7178595812873,-74.2507502221464,
70.3476595574776));
#206629=CARTESIAN_POINT('Ctrl Pts',(-52.752096062351,-74.2210464530811,
69.2719619690269));
#206630=CARTESIAN_POINT('Ctrl Pts',(-52.7688275234276,-74.2533190989187,
68.7382583579621));
#206631=CARTESIAN_POINT('Ctrl Pts',(-52.8016868286785,-74.4059514719878,
67.7172952524294));
#206632=CARTESIAN_POINT('Ctrl Pts',(-52.8177219971952,-74.5201382176993,
67.2310193615866));
#206633=CARTESIAN_POINT('Ctrl Pts',(-52.867566236269,-74.9988198589066,
65.7513459596427));
#206634=CARTESIAN_POINT('Ctrl Pts',(-52.90022275574,-75.4967926656062,64.8104686040742));
#206635=CARTESIAN_POINT('Ctrl Pts',(-52.9434349944675,-76.3254294934196,
63.7442985008549));
#206636=CARTESIAN_POINT('Ctrl Pts',(-52.9528453118307,-76.5168628756349,
63.5212006958766));
#206637=CARTESIAN_POINT('Ctrl Pts',(-52.9767428589438,-77.034707258445,
62.9737704318796));
#206638=CARTESIAN_POINT('Ctrl Pts',(-52.9910699917563,-77.3755367382101,
62.6642244244901));
#206639=CARTESIAN_POINT('Ctrl Pts',(-53.0242260319202,-78.2065432609747,
62.0172722664003));
#206640=CARTESIAN_POINT('Ctrl Pts',(-53.0431193134892,-78.7093350915824,
61.6994762410419));
#206641=CARTESIAN_POINT('Ctrl Pts',(-53.0807685885445,-79.7650676593376,
61.168733962228));
#206642=CARTESIAN_POINT('Ctrl Pts',(-53.0990847605614,-80.3150535149487,
60.9561548028325));
#206643=CARTESIAN_POINT('Ctrl Pts',(-53.1268493395572,-81.1679120998688,
60.7184347319786));
#206644=CARTESIAN_POINT('Ctrl Pts',(-53.1362014375202,-81.45784823377,60.6527416001073));
#206645=CARTESIAN_POINT('Ctrl Pts',(-53.1623121165999,-82.2698361804076,
60.5101806660068));
#206646=CARTESIAN_POINT('Ctrl Pts',(-53.1791828605216,-82.7961449935915,
60.4643601668526));
#206647=CARTESIAN_POINT('Ctrl Pts',(-53.2124636760748,-83.8540302211001,
60.4644846454046));
#206648=CARTESIAN_POINT('Ctrl Pts',(-53.2288874125688,-84.3835885296855,
60.5110010669611));
#206649=CARTESIAN_POINT('Ctrl Pts',(-53.2610378261074,-85.3907108882269,
60.6891878464769));
#206650=CARTESIAN_POINT('Ctrl Pts',(-53.276671043153,-85.8675957484608,
60.81415561908));
#206651=CARTESIAN_POINT('Ctrl Pts',(-53.3108764445405,-86.8846094766451,
61.1710049267115));
#206652=CARTESIAN_POINT('Ctrl Pts',(-53.3290479274024,-87.4171800085415,
61.4178495324768));
#206653=CARTESIAN_POINT('Ctrl Pts',(-53.3566688180232,-88.178992072836,
61.8648066055644));
#206654=CARTESIAN_POINT('Ctrl Pts',(-53.3660137267013,-88.4281347463818,
62.0279251561229));
#206655=CARTESIAN_POINT('Ctrl Pts',(-53.3911629094711,-89.0716763700902,
62.4959452841395));
#206656=CARTESIAN_POINT('Ctrl Pts',(-53.407066244405,-89.4497625944017,
62.8215380421825));
#206657=CARTESIAN_POINT('Ctrl Pts',(-53.4377452891996,-90.1332324938202,
63.5156011965559));
#206658=CARTESIAN_POINT('Ctrl Pts',(-53.4524840198263,-90.4400476533254,
63.8804524211517));
#206659=CARTESIAN_POINT('Ctrl Pts',(-53.4842724605499,-91.0298464419758,
64.7053810477322));
#206660=CARTESIAN_POINT('Ctrl Pts',(-53.5013290324563,-91.303323594756,
65.1700373453449));
#206661=CARTESIAN_POINT('Ctrl Pts',(-53.5234014509498,-91.6010007635352,
65.7970814828092));
#206662=CARTESIAN_POINT('Ctrl Pts',(-53.5283529317896,-91.6641978752785,
65.9395696054042));
#206663=CARTESIAN_POINT('Ctrl Pts',(-53.5332787937083,-91.723644464317,
66.0834535849087));
#206664=CARTESIAN_POINT('Ctrl Pts',(-53.7366673713217,-91.723644464317,
66.0834535849086));
#206665=CARTESIAN_POINT('Ctrl Pts',(-53.7081486511214,-91.3819206498898,
65.2563483950824));
#206666=CARTESIAN_POINT('Ctrl Pts',(-53.6799428389359,-90.9192504983588,
64.4826307592131));
#206667=CARTESIAN_POINT('Ctrl Pts',(-53.6205979136531,-89.7534812546762,
63.061961521807));
#206668=CARTESIAN_POINT('Ctrl Pts',(-53.5911706934458,-89.0485028626822,
62.4324452838763));
#206669=CARTESIAN_POINT('Ctrl Pts',(-53.5444755169724,-87.8271557109556,
61.6423679278073));
#206670=CARTESIAN_POINT('Ctrl Pts',(-53.5277536797414,-87.3716511843474,
61.3998546839219));
#206671=CARTESIAN_POINT('Ctrl Pts',(-53.4943639663923,-86.4161470981597,
60.9910383146938));
#206672=CARTESIAN_POINT('Ctrl Pts',(-53.477868827646,-85.9172934505708,
60.8269172316276));
#206673=CARTESIAN_POINT('Ctrl Pts',(-53.4516685615217,-85.1176832971479,
60.6385142777415));
#206674=CARTESIAN_POINT('Ctrl Pts',(-53.4421396712361,-84.8251140688993,
60.5845666347126));
#206675=CARTESIAN_POINT('Ctrl Pts',(-53.4136787459053,-83.9496869128899,
60.4671831011763));
#206676=CARTESIAN_POINT('Ctrl Pts',(-53.3947130266225,-83.3627652415183,
60.4456456603646));
#206677=CARTESIAN_POINT('Ctrl Pts',(-53.3575363906055,-82.1948539359201,
60.5157322882943));
#206678=CARTESIAN_POINT('Ctrl Pts',(-53.3390801383436,-81.6165748291615,
60.606826546077));
#206679=CARTESIAN_POINT('Ctrl Pts',(-53.3051724791001,-80.5946300775601,
60.8705451302912));
#206680=CARTESIAN_POINT('Ctrl Pts',(-53.2899012688467,-80.1480680465343,
61.023648320535));
#206681=CARTESIAN_POINT('Ctrl Pts',(-53.258092727956,-79.2349494413321,
61.4183846660114));
#206682=CARTESIAN_POINT('Ctrl Pts',(-53.2416775377997,-78.7733335208115,
61.6671913019313));
#206683=CARTESIAN_POINT('Ctrl Pts',(-53.2048870899337,-77.8060578531907,
62.3018490196695));
#206684=CARTESIAN_POINT('Ctrl Pts',(-53.1844570247185,-77.3141925598406,
62.7037762270346));
#206685=CARTESIAN_POINT('Ctrl Pts',(-53.1464175027061,-76.4771458758857,
63.54779452327));
#206686=CARTESIAN_POINT('Ctrl Pts',(-53.1290649933464,-76.123105667652,
63.9770289722223));
#206687=CARTESIAN_POINT('Ctrl Pts',(-53.1021126849508,-75.6438721313054,
64.680339003139));
#206688=CARTESIAN_POINT('Ctrl Pts',(-53.0927016830157,-75.4893308377453,
64.9327836264796));
#206689=CARTESIAN_POINT('Ctrl Pts',(-53.0642539903233,-75.062400958165,
65.7133038623293));
#206690=CARTESIAN_POINT('Ctrl Pts',(-53.0451961493636,-74.829161823644,
66.2609771893408));
#206691=CARTESIAN_POINT('Ctrl Pts',(-53.0099273872458,-74.4931319576961,
67.3294870084385));
#206692=CARTESIAN_POINT('Ctrl Pts',(-52.993448087483,-74.3791499280365,
67.844258133295));
#206693=CARTESIAN_POINT('Ctrl Pts',(-52.9606545795369,-74.2441998094337,
68.8675436550239));
#206694=CARTESIAN_POINT('Ctrl Pts',(-52.9444199327525,-74.2200408829854,
69.3737424775123));
#206695=CARTESIAN_POINT('Ctrl Pts',(-52.9115850000357,-74.2570604093489,
70.4090587406393));
#206696=CARTESIAN_POINT('Ctrl Pts',(-52.8951339010643,-74.3223038731665,
70.9361344387688));
#206697=CARTESIAN_POINT('Ctrl Pts',(-52.8691675386007,-74.4947513726767,
71.7429312181892));
#206698=CARTESIAN_POINT('Ctrl Pts',(-52.8598398246234,-74.5703985491578,
72.0281757097949));
#206699=CARTESIAN_POINT('Ctrl Pts',(-52.831441180149,-74.8411860763033,
72.8796970721193));
#206700=CARTESIAN_POINT('Ctrl Pts',(-52.8123827895505,-75.0785053588338,
73.4308543314911));
#206701=CARTESIAN_POINT('Ctrl Pts',(-52.7779731269084,-75.6110275476858,
74.3934818088159));
#206702=CARTESIAN_POINT('Ctrl Pts',(-52.7623446454619,-75.8896711784268,
74.8114506577758));
#206703=CARTESIAN_POINT('Ctrl Pts',(-52.7308414567282,-76.5093068977027,
75.5924397235683));
#206704=CARTESIAN_POINT('Ctrl Pts',(-52.7150256792488,-76.8484732181349,
75.9547500962502));
#206705=CARTESIAN_POINT('Ctrl Pts',(-52.6828410795849,-77.603471320067,
76.6395301983887));
#206706=CARTESIAN_POINT('Ctrl Pts',(-52.6666477548464,-78.0211694719652,
76.9572517435316));
#206707=CARTESIAN_POINT('Ctrl Pts',(-52.6324118986522,-78.9444518435359,
77.541125514525));
#206708=CARTESIAN_POINT('Ctrl Pts',(-52.6143779457094,-79.4524560329032,
77.7992628054456));
#206709=CARTESIAN_POINT('Ctrl Pts',(-52.5783259604422,-80.5092209315993,
78.2169250335483));
#206710=CARTESIAN_POINT('Ctrl Pts',(-52.5607000542427,-81.0556045471753,
78.3756791360494));
#206711=CARTESIAN_POINT('Ctrl Pts',(-52.5248209603296,-82.1825893786859,
78.5914287432175));
#206712=CARTESIAN_POINT('Ctrl Pts',(-52.5065068731459,-82.7610782936583,
78.6457117134075));
#206713=CARTESIAN_POINT('Ctrl Pts',(-52.4503909217026,-84.526672052444,
78.64213871166));
#206714=CARTESIAN_POINT('Ctrl Pts',(-52.4140519239493,-85.7007150635981,
78.407692612271));
#206715=CARTESIAN_POINT('Ctrl Pts',(-52.3669348165057,-87.0678498890913,
77.8422494937059));
#206716=CARTESIAN_POINT('Ctrl Pts',(-52.3575824285834,-87.3335287584867,
77.716976802084));
#206717=CARTESIAN_POINT('Ctrl Pts',(-52.3314086005314,-88.0664208126591,
77.3269663614386));
#206718=CARTESIAN_POINT('Ctrl Pts',(-52.3147453575165,-88.5169069175132,
77.0334075397887));
#206719=CARTESIAN_POINT('Ctrl Pts',(-52.278844705326,-89.4109679345417,
76.3308417521056));
#206720=CARTESIAN_POINT('Ctrl Pts',(-52.259599526264,-89.8451558968429,
75.9139890291635));
#206721=CARTESIAN_POINT('Ctrl Pts',(-52.2200211865281,-90.6535981838277,
74.9672514545419));
#206722=CARTESIAN_POINT('Ctrl Pts',(-52.200021894855,-91.0188254223797,
74.4339856300373));
#206723=CARTESIAN_POINT('Ctrl Pts',(-52.1605548288282,-91.6091501467412,
73.3384892655007));
#206724=CARTESIAN_POINT('Ctrl Pts',(-52.141237348591,-91.8407471212749,
72.7835176472257));
#206725=CARTESIAN_POINT('Ctrl Pts',(-52.1044422891552,-92.178169658784,
71.6787799226605));
#206726=CARTESIAN_POINT('Ctrl Pts',(-52.0871102535623,-92.291365931404,
71.1340196262976));
#206727=CARTESIAN_POINT('Ctrl Pts',(-52.0424985454643,-92.4502601798141,
69.7378150761446));
#206728=CARTESIAN_POINT('Ctrl Pts',(-52.0149900853586,-92.4274449726464,
68.8839662172004));
#206729=CARTESIAN_POINT('Ctrl Pts',(-51.9700176984552,-92.1917695500525,
67.4837102574374));
#206730=CARTESIAN_POINT('Ctrl Pts',(-51.9520345802026,-92.0445164227658,
66.9317944930678));
#206731=CARTESIAN_POINT('Ctrl Pts',(-51.9301340171887,-91.807517641383,
66.2919126336795));
#206732=CARTESIAN_POINT('Ctrl Pts',(-51.9265206085477,-91.7665388982637,
66.187274879867));
#206733=CARTESIAN_POINT('Ctrl Pts',(-51.9229031371334,-91.723644464317,
66.0834535849086));
#206734=CARTESIAN_POINT('Origin',(-54.462516693425,-83.3223805071439,69.5544896765311));
#206735=CARTESIAN_POINT('',(-49.9050113929448,-91.723644464317,66.0834535849087));
#206736=CARTESIAN_POINT('',(-50.1089321285242,-91.723644464317,66.0834535849087));
#206737=CARTESIAN_POINT('',(-54.462516693425,-91.723644464317,66.0834535849087));
#206738=CARTESIAN_POINT('Ctrl Pts',(-49.9050113929448,-91.723644464317,
66.0834535849087));
#206739=CARTESIAN_POINT('Ctrl Pts',(-49.9147117058398,-91.8403594377234,
66.3659494372877));
#206740=CARTESIAN_POINT('Ctrl Pts',(-49.9244626372976,-91.9428230910478,
66.6543254260075));
#206741=CARTESIAN_POINT('Ctrl Pts',(-49.9517309550091,-92.1890499511924,
67.4768052963225));
#206742=CARTESIAN_POINT('Ctrl Pts',(-49.9688935132306,-92.2989198871257,
68.0194516718644));
#206743=CARTESIAN_POINT('Ctrl Pts',(-50.0043898234736,-92.4215248738981,
69.1433469378638));
#206744=CARTESIAN_POINT('Ctrl Pts',(-50.0227509272814,-92.4292556160134,
69.7226515170119));
#206745=CARTESIAN_POINT('Ctrl Pts',(-50.0700821175691,-92.3078097536682,
71.2009650734095));
#206746=CARTESIAN_POINT('Ctrl Pts',(-50.0980432890603,-92.0993310317001,
72.0870703510565));
#206747=CARTESIAN_POINT('Ctrl Pts',(-50.1425875368639,-91.5798671404784,
73.3869633985969));
#206748=CARTESIAN_POINT('Ctrl Pts',(-50.1584973666223,-91.3591583619826,
73.8304852136159));
#206749=CARTESIAN_POINT('Ctrl Pts',(-50.1835782418007,-90.9516542433398,
74.505221860558));
#206750=CARTESIAN_POINT('Ctrl Pts',(-50.1928159371108,-90.7877440328881,
74.7490941130108));
#206751=CARTESIAN_POINT('Ctrl Pts',(-50.2396278932642,-89.9002769757862,
75.9405196464941));
#206752=CARTESIAN_POINT('Ctrl Pts',(-50.2779141269498,-89.0071221000094,
76.7471110380068));
#206753=CARTESIAN_POINT('Ctrl Pts',(-50.3530205098722,-86.9676506000635,
77.9653378464173));
#206754=CARTESIAN_POINT('Ctrl Pts',(-50.3911527776497,-85.8426406719233,
78.3680389196349));
#206755=CARTESIAN_POINT('Ctrl Pts',(-50.4454549028411,-84.1491389977272,
78.6223152913914));
#206756=CARTESIAN_POINT('Ctrl Pts',(-50.4622048143095,-83.620317206025,
78.6550511697303));
#206757=CARTESIAN_POINT('Ctrl Pts',(-50.4946443774774,-82.6115628902654,
78.6294391630879));
#206758=CARTESIAN_POINT('Ctrl Pts',(-50.5102295271332,-82.133187995805,
78.5792217354898));
#206759=CARTESIAN_POINT('Ctrl Pts',(-50.5416388860715,-81.1692545932663,
78.4000294669564));
#206760=CARTESIAN_POINT('Ctrl Pts',(-50.5573857379669,-80.6858640745953,
78.2681750298379));
#206761=CARTESIAN_POINT('Ctrl Pts',(-50.582839067233,-79.936093350969,77.9955177805239));
#206762=CARTESIAN_POINT('Ctrl Pts',(-50.5923829353959,-79.6615733493138,
77.8801359072546));
#206763=CARTESIAN_POINT('Ctrl Pts',(-50.6208596996984,-78.865131215324,
77.4983677315371));
#206764=CARTESIAN_POINT('Ctrl Pts',(-50.6398117578377,-78.3627405419623,
77.1947944437293));
#206765=CARTESIAN_POINT('Ctrl Pts',(-50.674092270101,-77.4980312629215,
76.5508360117242));
#206766=CARTESIAN_POINT('Ctrl Pts',(-50.6896804164518,-77.1275757909721,
76.2250442796543));
#206767=CARTESIAN_POINT('Ctrl Pts',(-50.7225253822295,-76.4162681619046,
75.4888854656735));
#206768=CARTESIAN_POINT('Ctrl Pts',(-50.7397636875988,-76.0813858709865,
75.075307743088));
#206769=CARTESIAN_POINT('Ctrl Pts',(-50.7737436312742,-75.4894710256001,
74.1970733708151));
#206770=CARTESIAN_POINT('Ctrl Pts',(-50.7903345038232,-75.2331056399603,
73.7344048003945));
#206771=CARTESIAN_POINT('Ctrl Pts',(-50.816619305745,-74.8975005736952,
72.980710162863));
#206772=CARTESIAN_POINT('Ctrl Pts',(-50.8261301328098,-74.7900308770867,
72.7035525028149));
#206773=CARTESIAN_POINT('Ctrl Pts',(-50.8546215199752,-74.510732181035,
71.8632576213085));
#206774=CARTESIAN_POINT('Ctrl Pts',(-50.8736088777131,-74.3797901664283,
71.2881709298883));
#206775=CARTESIAN_POINT('Ctrl Pts',(-50.9110524784387,-74.2302936511775,
70.1159668952692));
#206776=CARTESIAN_POINT('Ctrl Pts',(-50.9297652579409,-74.2130331102534,
69.5215277769831));
#206777=CARTESIAN_POINT('Ctrl Pts',(-50.9680212726247,-74.2950623682846,
68.3309801614858));
#206778=CARTESIAN_POINT('Ctrl Pts',(-50.9873686041531,-74.3954959605317,
67.7378450388702));
#206779=CARTESIAN_POINT('Ctrl Pts',(-51.0224252766225,-74.6877939353173,
66.6679078683688));
#206780=CARTESIAN_POINT('Ctrl Pts',(-51.0384077358017,-74.8629495866275,
66.189007899432));
#206781=CARTESIAN_POINT('Ctrl Pts',(-51.0710032714289,-75.2939730226834,
65.2604331227147));
#206782=CARTESIAN_POINT('Ctrl Pts',(-51.0875646029802,-75.5499389045143,
64.8128238155847));
#206783=CARTESIAN_POINT('Ctrl Pts',(-51.1213167918691,-76.1521548514087,
63.940725506023));
#206784=CARTESIAN_POINT('Ctrl Pts',(-51.1382849145464,-76.501627236609,
63.5209325142995));
#206785=CARTESIAN_POINT('Ctrl Pts',(-51.1648071070228,-77.095135998754,
62.9259189949457));
#206786=CARTESIAN_POINT('Ctrl Pts',(-51.1741696656935,-77.313734766831,
62.7271404034891));
#206787=CARTESIAN_POINT('Ctrl Pts',(-51.2026019892191,-78.0023405478588,
62.1597006176973));
#206788=CARTESIAN_POINT('Ctrl Pts',(-51.2216756010864,-78.4993519598212,
61.8263499545555));
#206789=CARTESIAN_POINT('Ctrl Pts',(-51.2575462095671,-79.5071897115629,
61.2857231149347));
#206790=CARTESIAN_POINT('Ctrl Pts',(-51.2746156182036,-80.0112589861578,
61.0712914152227));
#206791=CARTESIAN_POINT('Ctrl Pts',(-51.3073510376501,-80.9940111643925,
60.7542525107014));
#206792=CARTESIAN_POINT('Ctrl Pts',(-51.3228975014517,-81.4677118574821,
60.6423810585827));
#206793=CARTESIAN_POINT('Ctrl Pts',(-51.3546038077785,-82.4603928963994,
60.4905549578654));
#206794=CARTESIAN_POINT('Ctrl Pts',(-51.3706491520746,-82.9784744867673,
60.4561563234838));
#206795=CARTESIAN_POINT('Ctrl Pts',(-51.4071574905776,-84.1411626825417,
60.4784519058709));
#206796=CARTESIAN_POINT('Ctrl Pts',(-51.4276977631762,-84.7825260302579,
60.5593340711432));
#206797=CARTESIAN_POINT('Ctrl Pts',(-51.465141603421,-85.9348060503362,
60.8312208899268));
#206798=CARTESIAN_POINT('Ctrl Pts',(-51.4818147229151,-86.4476390286903,
61.0015400989278));
#206799=CARTESIAN_POINT('Ctrl Pts',(-51.5074430548604,-87.1981167133596,
61.3273548868817));
#206800=CARTESIAN_POINT('Ctrl Pts',(-51.5162169552698,-87.4486437936567,
61.4501064345573));
#206801=CARTESIAN_POINT('Ctrl Pts',(-51.5439484223193,-88.2171101271034,
61.8715170606771));
#206802=CARTESIAN_POINT('Ctrl Pts',(-51.5629968860554,-88.711485320593,
62.2098310629754));
#206803=CARTESIAN_POINT('Ctrl Pts',(-51.5957845290705,-89.5144903712622,
62.884361891401));
#206804=CARTESIAN_POINT('Ctrl Pts',(-51.6097993152967,-89.8378284318547,
63.1998246909724));
#206805=CARTESIAN_POINT('Ctrl Pts',(-51.6458717535102,-90.5967266573389,
64.0593190861755));
#206806=CARTESIAN_POINT('Ctrl Pts',(-51.6681372105029,-90.9956956352514,
64.6317619870711));
#206807=CARTESIAN_POINT('Ctrl Pts',(-51.6997074378457,-91.4725125845283,
65.5170628329408));
#206808=CARTESIAN_POINT('Ctrl Pts',(-51.7093578146623,-91.6053893697283,
65.7972300373293));
#206809=CARTESIAN_POINT('Ctrl Pts',(-51.7190489450981,-91.723644464317,
66.0834535849086));
#206810=CARTESIAN_POINT('Ctrl Pts',(-51.9229031371334,-91.723644464317,
66.0834535849086));
#206811=CARTESIAN_POINT('Ctrl Pts',(-51.9106399629138,-91.5782329720614,
65.7315009412026));
#206812=CARTESIAN_POINT('Ctrl Pts',(-51.8983152146373,-91.4108065720598,
65.388931473677));
#206813=CARTESIAN_POINT('Ctrl Pts',(-51.8701233880306,-90.9746246996887,
64.6226343007356));
#206814=CARTESIAN_POINT('Ctrl Pts',(-51.8543741618664,-90.6913995856782,
64.2086873870961));
#206815=CARTESIAN_POINT('Ctrl Pts',(-51.8079342398151,-89.7727445766005,
63.0787512514185));
#206816=CARTESIAN_POINT('Ctrl Pts',(-51.7769543255324,-89.0568057887049,
62.4369932458205));
#206817=CARTESIAN_POINT('Ctrl Pts',(-51.7089989440773,-87.2593857639417,
61.276109628659));
#206818=CARTESIAN_POINT('Ctrl Pts',(-51.6707264611623,-86.148627410159,
60.8341728469488));
#206819=CARTESIAN_POINT('Ctrl Pts',(-51.6238049046546,-84.6963343560413,
60.5640814951426));
#206820=CARTESIAN_POINT('Ctrl Pts',(-51.6145142495458,-84.405832334073,
60.5244664165164));
#206821=CARTESIAN_POINT('Ctrl Pts',(-51.5884431318578,-83.5916651291978,
60.4532999788211));
#206822=CARTESIAN_POINT('Ctrl Pts',(-51.5715430527392,-83.0664361370525,
60.4529155628379));
#206823=CARTESIAN_POINT('Ctrl Pts',(-51.535308385102,-81.947820903818,60.5490408300095));
#206824=CARTESIAN_POINT('Ctrl Pts',(-51.5164050182772,-81.3580404309915,
60.6590471765668));
#206825=CARTESIAN_POINT('Ctrl Pts',(-51.4880282358771,-80.500116496568,
60.9086137543441));
#206826=CARTESIAN_POINT('Ctrl Pts',(-51.4786269281836,-80.2210511450564,
61.0047470400078));
#206827=CARTESIAN_POINT('Ctrl Pts',(-51.4523421667,-79.4599662404302,61.3091033972305));
#206828=CARTESIAN_POINT('Ctrl Pts',(-51.4353421259464,-78.9905602503028,
61.54574621155));
#206829=CARTESIAN_POINT('Ctrl Pts',(-51.4032381396794,-78.1343302965438,
62.0748110955611));
#206830=CARTESIAN_POINT('Ctrl Pts',(-51.3881229843155,-77.7452453340655,
62.360254081977));
#206831=CARTESIAN_POINT('Ctrl Pts',(-51.354982436646,-76.955189235919,63.0426378803104));
#206832=CARTESIAN_POINT('Ctrl Pts',(-51.3369374176284,-76.5647631745038,
63.4487599330444));
#206833=CARTESIAN_POINT('Ctrl Pts',(-51.2998470461721,-75.8440821528249,
64.3528310350224));
#206834=CARTESIAN_POINT('Ctrl Pts',(-51.2812367383216,-75.520226204611,
64.8525122607279));
#206835=CARTESIAN_POINT('Ctrl Pts',(-51.2531349279433,-75.1116241412943,
65.6429327668723));
#206836=CARTESIAN_POINT('Ctrl Pts',(-51.2437586862846,-74.9887139169713,
65.9121282087519));
#206837=CARTESIAN_POINT('Ctrl Pts',(-51.2165748688895,-74.6728940874802,
66.7039373935078));
#206838=CARTESIAN_POINT('Ctrl Pts',(-51.1986581480155,-74.5145816307207,
67.238900554646));
#206839=CARTESIAN_POINT('Ctrl Pts',(-51.1608150331806,-74.2811988780267,
68.4148645041512));
#206840=CARTESIAN_POINT('Ctrl Pts',(-51.1408235386528,-74.2232899091996,
69.0562266421446));
#206841=CARTESIAN_POINT('Ctrl Pts',(-51.1035004545141,-74.2418834701496,
70.2311850277702));
#206842=CARTESIAN_POINT('Ctrl Pts',(-51.0864006493592,-74.2971604917727,
70.7622769462743));
#206843=CARTESIAN_POINT('Ctrl Pts',(-51.0531588352697,-74.497848223116,
71.7968903224989));
#206844=CARTESIAN_POINT('Ctrl Pts',(-51.0369912006251,-74.6408351811626,
72.2988488558184));
#206845=CARTESIAN_POINT('Ctrl Pts',(-51.0045451824436,-75.007113482696,
73.2619375189264));
#206846=CARTESIAN_POINT('Ctrl Pts',(-50.9883338827073,-75.2279046094035,
73.7220174218051));
#206847=CARTESIAN_POINT('Ctrl Pts',(-50.9535162065867,-75.7831574417221,
74.6665453786056));
#206848=CARTESIAN_POINT('Ctrl Pts',(-50.9353159240416,-76.1284414515151,
75.1419974076811));
#206849=CARTESIAN_POINT('Ctrl Pts',(-50.9076553343251,-76.7142304625479,
75.8034975351984));
#206850=CARTESIAN_POINT('Ctrl Pts',(-50.8983092076004,-76.922168045955,
76.0163024970541));
#206851=CARTESIAN_POINT('Ctrl Pts',(-50.8724112326359,-77.5224592529502,
76.5731916946453));
#206852=CARTESIAN_POINT('Ctrl Pts',(-50.8557516463148,-77.9345705998867,
76.8942970631852));
#206853=CARTESIAN_POINT('Ctrl Pts',(-50.8237908919568,-78.7877050486375,
77.4482720631052));
#206854=CARTESIAN_POINT('Ctrl Pts',(-50.8084473301634,-79.2248670555909,
77.6837866951273));
#206855=CARTESIAN_POINT('Ctrl Pts',(-50.7771862969671,-80.137596815985,
78.0830881309289));
#206856=CARTESIAN_POINT('Ctrl Pts',(-50.7613140591261,-80.6119298540795,
78.2454785681636));
#206857=CARTESIAN_POINT('Ctrl Pts',(-50.7268304996241,-81.6650034234414,
78.5113515181957));
#206858=CARTESIAN_POINT('Ctrl Pts',(-50.7086164197141,-82.2453277591109,
78.5995013127753));
#206859=CARTESIAN_POINT('Ctrl Pts',(-50.6715587960687,-83.4286575002796,
78.6636813055427));
#206860=CARTESIAN_POINT('Ctrl Pts',(-50.6526148129697,-84.0289673562377,
78.636856509736));
#206861=CARTESIAN_POINT('Ctrl Pts',(-50.5958211608329,-85.7965787181752,
78.3814666021691));
#206862=CARTESIAN_POINT('Ctrl Pts',(-50.5594309811275,-86.9264079236248,
77.9834964909913));
#206863=CARTESIAN_POINT('Ctrl Pts',(-50.4835875375019,-88.9745054927381,
76.7728785011232));
#206864=CARTESIAN_POINT('Ctrl Pts',(-50.4469037372857,-89.8717786780052,
75.9698648153537));
#206865=CARTESIAN_POINT('Ctrl Pts',(-50.3993945748335,-90.7645684248745,
74.7822158909312));
#206866=CARTESIAN_POINT('Ctrl Pts',(-50.3900079168931,-90.9292958464928,
74.5394794443228));
#206867=CARTESIAN_POINT('Ctrl Pts',(-50.3646250050068,-91.346276569298,
73.8560988857613));
#206868=CARTESIAN_POINT('Ctrl Pts',(-50.3487970710957,-91.5738238983745,
73.4016233069964));
#206869=CARTESIAN_POINT('Ctrl Pts',(-50.3040285835809,-92.0990337173014,
72.0886371055357));
#206870=CARTESIAN_POINT('Ctrl Pts',(-50.2747816579962,-92.3079433485688,
71.2010642612718));
#206871=CARTESIAN_POINT('Ctrl Pts',(-50.2278832161795,-92.4292882696803,
69.7211517899185));
#206872=CARTESIAN_POINT('Ctrl Pts',(-50.2096316899784,-92.4214578548965,
69.1417799494627));
#206873=CARTESIAN_POINT('Ctrl Pts',(-50.1733173469438,-92.2985382661797,
68.01686814027));
#206874=CARTESIAN_POINT('Ctrl Pts',(-50.1554343546318,-92.1882849888544,
67.4732789761947));
#206875=CARTESIAN_POINT('Ctrl Pts',(-50.1282000266549,-91.9417963729096,
66.6514363404576));
#206876=CARTESIAN_POINT('Ctrl Pts',(-50.1185905671141,-91.8397738343069,
66.3645320481434));
#206877=CARTESIAN_POINT('Ctrl Pts',(-50.1089321285242,-91.723644464317,
66.0834535849087));
#206878=CARTESIAN_POINT('Origin',(-61.5936228798467,-83.3229197588524,69.5524554490053));
#206879=CARTESIAN_POINT('',(-62.602329162019,-91.7241837160256,66.0814193573896));
#206880=CARTESIAN_POINT('',(-62.8075051404766,-91.7241532646522,66.0813456540805));
#206881=CARTESIAN_POINT('',(-61.5936228798467,-91.7241837160232,66.0814193573838));
#206882=CARTESIAN_POINT('',(-62.6023317437084,-91.724214653637,66.0814942394464));
#206883=CARTESIAN_POINT('Ctrl Pts',(-62.602329162019,-91.724183716028,66.0814193573955));
#206884=CARTESIAN_POINT('Ctrl Pts',(-62.6023301287422,-91.7241953008589,
66.0814473972141));
#206885=CARTESIAN_POINT('Ctrl Pts',(-62.6023307769843,-91.7242030690519,
66.0814661995147));
#206886=CARTESIAN_POINT('Ctrl Pts',(-62.6023317437084,-91.724214653637,
66.0814942394464));
#206887=CARTESIAN_POINT('',(-62.7290132089978,-92.4053664431831,69.9232336695063));
#206888=CARTESIAN_POINT('Ctrl Pts',(-62.7269877844547,-92.4054200988458,
69.9232858703778));
#206889=CARTESIAN_POINT('Ctrl Pts',(-62.7059767167849,-92.4321833496604,
69.2677915511049));
#206890=CARTESIAN_POINT('Ctrl Pts',(-62.6852394928937,-92.3879069276803,
68.6113136984254));
#206891=CARTESIAN_POINT('Ctrl Pts',(-62.6544240531954,-92.2165542002343,
67.6449849877673));
#206892=CARTESIAN_POINT('Ctrl Pts',(-62.6442290356213,-92.1425921867259,
67.3279207418242));
#206893=CARTESIAN_POINT('Ctrl Pts',(-62.6234162513844,-91.959643018198,
66.6984486864254));
#206894=CARTESIAN_POINT('Ctrl Pts',(-62.6128525065425,-91.8502885457368,
66.3866500398474));
#206895=CARTESIAN_POINT('Ctrl Pts',(-62.6023317437084,-91.724214653637,
66.0814942394464));
#206896=CARTESIAN_POINT('',(-62.9304638037219,-92.4054950025943,69.9232129291766));
#206897=CARTESIAN_POINT('',(-62.9299583493521,-92.4054226835952,69.9232225584337));
#206898=CARTESIAN_POINT('Ctrl Pts',(-62.9325038108326,-92.4054252108019,
69.9231606454937));
#206899=CARTESIAN_POINT('Ctrl Pts',(-62.9116762546274,-92.4324227266438,
69.2617048926575));
#206900=CARTESIAN_POINT('Ctrl Pts',(-62.8907033964332,-92.3870813596432,
68.5992795630952));
#206901=CARTESIAN_POINT('Ctrl Pts',(-62.8591164531908,-92.2133065594351,
67.630413397562));
#206902=CARTESIAN_POINT('Ctrl Pts',(-62.8487672428674,-92.1395668305264,
67.3163960992237));
#206903=CARTESIAN_POINT('Ctrl Pts',(-62.8281485913344,-91.9576684801071,
66.6928186370739));
#206904=CARTESIAN_POINT('Ctrl Pts',(-62.8178556351414,-91.8491373548634,
66.3838560001025));
#206905=CARTESIAN_POINT('Ctrl Pts',(-62.8075076622656,-91.7241837160232,
66.0814193573838));
#206906=CARTESIAN_POINT('Origin',(-61.5936228798467,-83.3229197588524,69.5524554490053));
#206907=CARTESIAN_POINT('',(-60.9932785231031,-91.7241837160232,66.0814193573838));
#206908=CARTESIAN_POINT('Ctrl Pts',(-62.8075051404766,-91.7241532646522,
66.0813456540805));
#206909=CARTESIAN_POINT('Ctrl Pts',(-62.782639448844,-91.4238893610732,
65.3546077182715));
#206910=CARTESIAN_POINT('Ctrl Pts',(-62.7573419230597,-91.030597562824,
64.6699048574091));
#206911=CARTESIAN_POINT('Ctrl Pts',(-62.707148163105,-90.0815230164625,
63.4239178672618));
#206912=CARTESIAN_POINT('Ctrl Pts',(-62.6828210378518,-89.5310041730699,
62.8668453774156));
#206913=CARTESIAN_POINT('Ctrl Pts',(-62.6414672514383,-88.5157511700844,
62.0743644731427));
#206914=CARTESIAN_POINT('Ctrl Pts',(-62.6249856508974,-88.0898489339138,
61.7959273286443));
#206915=CARTESIAN_POINT('Ctrl Pts',(-62.5930729332684,-87.2118569051275,
61.3216881943479));
#206916=CARTESIAN_POINT('Ctrl Pts',(-62.5776490581675,-86.7626672683054,
61.1240805190056));
#206917=CARTESIAN_POINT('Ctrl Pts',(-62.5525262949722,-86.0184966553697,
60.8661561273298));
#206918=CARTESIAN_POINT('Ctrl Pts',(-62.5429812228712,-85.7326311968053,
60.7825512578548));
#206919=CARTESIAN_POINT('Ctrl Pts',(-62.514502824905,-84.8736473974892,
60.5765095750246));
#206920=CARTESIAN_POINT('Ctrl Pts',(-62.4955585715648,-84.2922326355718,
60.4952589399396));
#206921=CARTESIAN_POINT('Ctrl Pts',(-62.4614485891902,-83.2202967080181,
60.4499200231851));
#206922=CARTESIAN_POINT('Ctrl Pts',(-62.4460230671324,-82.7326752762972,
60.4684975069705));
#206923=CARTESIAN_POINT('Ctrl Pts',(-62.4159521898034,-81.8022927836982,
60.5792006119913));
#206924=CARTESIAN_POINT('Ctrl Pts',(-62.4013844885234,-81.3602465161134,
60.6654132792302));
#206925=CARTESIAN_POINT('Ctrl Pts',(-62.3687077150992,-80.3823426440256,
60.9326845723041));
#206926=CARTESIAN_POINT('Ctrl Pts',(-62.3509474293283,-79.8533019520944,
61.1316955046727));
#206927=CARTESIAN_POINT('Ctrl Pts',(-62.3111515418468,-78.7293331677781,
61.6785259783383));
#206928=CARTESIAN_POINT('Ctrl Pts',(-62.2889855702203,-78.1484885668729,
62.0474542048791));
#206929=CARTESIAN_POINT('Ctrl Pts',(-62.2490753870823,-77.182021724831,
62.8272944155795));
#206930=CARTESIAN_POINT('Ctrl Pts',(-62.2316233663111,-76.7822923162096,
63.2153729809014));
#206931=CARTESIAN_POINT('Ctrl Pts',(-62.1957585642899,-76.048300806116,
64.0719012677919));
#206932=CARTESIAN_POINT('Ctrl Pts',(-62.177365850264,-75.7179090234939,
64.5404343917883));
#206933=CARTESIAN_POINT('Ctrl Pts',(-62.1407644355438,-75.1524904511458,
65.5282806228294));
#206934=CARTESIAN_POINT('Ctrl Pts',(-62.1229501544509,-74.9177564980146,
66.044873170331));
#206935=CARTESIAN_POINT('Ctrl Pts',(-62.0821006216508,-74.4954880525488,
67.2651918735177));
#206936=CARTESIAN_POINT('Ctrl Pts',(-62.0588399413442,-74.3412146325176,
67.9763609271869));
#206937=CARTESIAN_POINT('Ctrl Pts',(-62.0175905436349,-74.219958136856,
69.2610146368297));
#206938=CARTESIAN_POINT('Ctrl Pts',(-61.9999561766462,-74.2194478550678,
69.8274997616061));
#206939=CARTESIAN_POINT('Ctrl Pts',(-61.9727822537456,-74.2987586045137,
70.6842487011262));
#206940=CARTESIAN_POINT('Ctrl Pts',(-61.9634197903071,-74.3402621771479,
70.9766399771102));
#206941=CARTESIAN_POINT('Ctrl Pts',(-61.9350310385132,-74.5081192292594,
71.8508693468088));
#206942=CARTESIAN_POINT('Ctrl Pts',(-61.9159586366291,-74.677435589082,
72.4228274415055));
#206943=CARTESIAN_POINT('Ctrl Pts',(-61.8816411707454,-75.0884653984842,
73.4344627389694));
#206944=CARTESIAN_POINT('Ctrl Pts',(-61.8661243319853,-75.3129300365894,
73.8786874224392));
#206945=CARTESIAN_POINT('Ctrl Pts',(-61.8333740462486,-75.8534949558486,
74.7607237962095));
#206946=CARTESIAN_POINT('Ctrl Pts',(-61.8161579512294,-76.174532531962,
75.1932816556839));
#206947=CARTESIAN_POINT('Ctrl Pts',(-61.7822899692345,-76.885707966164,
75.9925579573077));
#206948=CARTESIAN_POINT('Ctrl Pts',(-61.7658024137524,-77.2737523608574,
76.3583494761944));
#206949=CARTESIAN_POINT('Ctrl Pts',(-61.7312727699392,-78.1366834708223,
77.0393646593839));
#206950=CARTESIAN_POINT('Ctrl Pts',(-61.713251789691,-78.6136932122976,
77.3482254816014));
#206951=CARTESIAN_POINT('Ctrl Pts',(-61.6772194918282,-79.6195922361186,
77.8733303829382));
#206952=CARTESIAN_POINT('Ctrl Pts',(-61.6595957716167,-80.1463361428618,
78.0883159448589));
#206953=CARTESIAN_POINT('Ctrl Pts',(-61.6237499877836,-81.2430951837849,
78.4202610611445));
#206954=CARTESIAN_POINT('Ctrl Pts',(-61.6054788586489,-81.8112227988724,
78.5345713663026));
#206955=CARTESIAN_POINT('Ctrl Pts',(-61.5495117122661,-83.5640688092825,
78.7161396148171));
#206956=CARTESIAN_POINT('Ctrl Pts',(-61.5132885942868,-84.7543668476728,
78.6068584711006));
#206957=CARTESIAN_POINT('Ctrl Pts',(-61.4439831094195,-86.8469514488567,
77.9907762249617));
#206958=CARTESIAN_POINT('Ctrl Pts',(-61.4133547643517,-87.7508638221166,
77.5535417050547));
#206959=CARTESIAN_POINT('Ctrl Pts',(-61.3725015184426,-88.8045667084337,
76.8096187940016));
#206960=CARTESIAN_POINT('Ctrl Pts',(-61.3631898701075,-89.0352192104166,
76.6294962908981));
#206961=CARTESIAN_POINT('Ctrl Pts',(-61.325135092192,-89.9415011458404,
75.8485398749232));
#206962=CARTESIAN_POINT('Ctrl Pts',(-61.2973272281126,-90.534398211703,
75.1596723383531));
#206963=CARTESIAN_POINT('Ctrl Pts',(-61.2495837013446,-91.3360001075092,
73.8861586684715));
#206964=CARTESIAN_POINT('Ctrl Pts',(-61.2303030811977,-91.6048968722122,
73.3470971633472));
#206965=CARTESIAN_POINT('Ctrl Pts',(-61.1925280821862,-92.031693432208,
72.2255569035656));
#206966=CARTESIAN_POINT('Ctrl Pts',(-61.1738414881785,-92.1888891937034,
71.6459682266556));
#206967=CARTESIAN_POINT('Ctrl Pts',(-61.1385650468259,-92.3722129896584,
70.5522622043069));
#206968=CARTESIAN_POINT('Ctrl Pts',(-61.1221597451864,-92.4140419477611,
70.0431837816635));
#206969=CARTESIAN_POINT('Ctrl Pts',(-61.096633182848,-92.4123489599951,
69.2400668706237));
#206970=CARTESIAN_POINT('Ctrl Pts',(-61.0874154894787,-92.3975428500331,
68.9470408089246));
#206971=CARTESIAN_POINT('Ctrl Pts',(-61.0501135215415,-92.2806775642666,
67.7688067151902));
#206972=CARTESIAN_POINT('Ctrl Pts',(-61.0216496146652,-92.0630968100072,
66.9017215051989));
#206973=CARTESIAN_POINT('Ctrl Pts',(-60.993278523103,-91.7241837160232,
66.0814193573839));
#206974=CARTESIAN_POINT('',(-60.7885639123434,-91.7241837160232,66.0814193573838));
#206975=CARTESIAN_POINT('',(-61.5936228798467,-91.7241837160232,66.0814193573838));
#206976=CARTESIAN_POINT('Ctrl Pts',(-60.7885639123434,-91.7241837160232,
66.0814193573838));
#206977=CARTESIAN_POINT('Ctrl Pts',(-60.8168982940386,-92.0672888336512,
66.9118678408229));
#206978=CARTESIAN_POINT('Ctrl Pts',(-60.8449183666358,-92.2859925617974,
67.7901443518347));
#206979=CARTESIAN_POINT('Ctrl Pts',(-60.8831526417602,-92.3996991184818,
68.9800704653405));
#206980=CARTESIAN_POINT('Ctrl Pts',(-60.8925524312737,-92.4134513972595,
69.2735559243787));
#206981=CARTESIAN_POINT('Ctrl Pts',(-60.9174368238779,-92.412178260678,
70.0588365261411));
#206982=CARTESIAN_POINT('Ctrl Pts',(-60.932787483143,-92.3714961568602,
70.5496070916347));
#206983=CARTESIAN_POINT('Ctrl Pts',(-60.9772216077173,-92.1426559184543,
71.9342410667884));
#206984=CARTESIAN_POINT('Ctrl Pts',(-61.0066354455244,-91.859482771096,
72.8063366536296));
#206985=CARTESIAN_POINT('Ctrl Pts',(-61.0537067591269,-91.192463652668,
74.1387394063432));
#206986=CARTESIAN_POINT('Ctrl Pts',(-61.0719689223178,-90.8848502493925,
74.6299470984856));
#206987=CARTESIAN_POINT('Ctrl Pts',(-61.1084338963099,-90.1929855909006,
75.5309673059974));
#206988=CARTESIAN_POINT('Ctrl Pts',(-61.126453524327,-89.8133021587206,
75.9411452521602));
#206989=CARTESIAN_POINT('Ctrl Pts',(-61.1633331215782,-88.949042409027,
76.7177232860578));
#206990=CARTESIAN_POINT('Ctrl Pts',(-61.1823779849551,-88.4605252890634,
77.0757078145086));
#206991=CARTESIAN_POINT('Ctrl Pts',(-61.2177278849416,-87.5125851856134,
77.6346813099218));
#206992=CARTESIAN_POINT('Ctrl Pts',(-61.2338320906311,-87.065121092545,
77.8513468946674));
#206993=CARTESIAN_POINT('Ctrl Pts',(-61.2656591486748,-86.1374434006063,
78.210175460382));
#206994=CARTESIAN_POINT('Ctrl Pts',(-61.2813449294374,-85.6586735055382,
78.3514280757492));
#206995=CARTESIAN_POINT('Ctrl Pts',(-61.3282500250971,-84.2192145915512,
78.650280335433));
#206996=CARTESIAN_POINT('Ctrl Pts',(-61.3597500356822,-83.2421341316582,
78.6939673325073));
#206997=CARTESIAN_POINT('Ctrl Pts',(-61.4282604264901,-81.0994589239397,
78.4457233733748));
#206998=CARTESIAN_POINT('Ctrl Pts',(-61.4665642768093,-79.9601101687614,
78.0803809269989));
#206999=CARTESIAN_POINT('Ctrl Pts',(-61.522559094674,-78.4165826313906,
77.2265761144129));
#207000=CARTESIAN_POINT('Ctrl Pts',(-61.5409287851939,-77.9380660966484,
76.8987208995993));
#207001=CARTESIAN_POINT('Ctrl Pts',(-61.5778530834986,-77.0582196363352,
76.1634578159226));
#207002=CARTESIAN_POINT('Ctrl Pts',(-61.596197134465,-76.6575364845791,
75.7592663609613));
#207003=CARTESIAN_POINT('Ctrl Pts',(-61.6322253585681,-75.9369036013822,
74.8814793368301));
#207004=CARTESIAN_POINT('Ctrl Pts',(-61.6501362005052,-75.6185290195753,
74.4098303908081));
#207005=CARTESIAN_POINT('Ctrl Pts',(-61.685821083523,-75.0845934510683,
73.4327905100171));
#207006=CARTESIAN_POINT('Ctrl Pts',(-61.7034793284167,-74.8665827823663,
72.9314187521735));
#207007=CARTESIAN_POINT('Ctrl Pts',(-61.73766044682,-74.5279868859487,71.9103238811904));
#207008=CARTESIAN_POINT('Ctrl Pts',(-61.7542661143291,-74.4054643287565,
71.3934826317876));
#207009=CARTESIAN_POINT('Ctrl Pts',(-61.7870276962639,-74.2562332221558,
70.3739160308934));
#207010=CARTESIAN_POINT('Ctrl Pts',(-61.8030966748672,-74.224769053084,
69.8737800427072));
#207011=CARTESIAN_POINT('Ctrl Pts',(-61.8522336467114,-74.2549710778356,
68.339027595969));
#207012=CARTESIAN_POINT('Ctrl Pts',(-61.8841769905295,-74.4518406136614,
67.3154811640129));
#207013=CARTESIAN_POINT('Ctrl Pts',(-61.9266147416522,-74.920079758707,
66.0728677985675));
#207014=CARTESIAN_POINT('Ctrl Pts',(-61.9359959635896,-75.0366477392345,
65.8037293725427));
#207015=CARTESIAN_POINT('Ctrl Pts',(-61.961424997767,-75.3904247045107,
65.084413189159));
#207016=CARTESIAN_POINT('Ctrl Pts',(-61.9772286572875,-75.6527247350318,
64.6477646308985));
#207017=CARTESIAN_POINT('Ctrl Pts',(-62.0115532880872,-76.2906467555519,
63.7632151083716));
#207018=CARTESIAN_POINT('Ctrl Pts',(-62.030089516706,-76.6757007497917,
63.3248849222721));
#207019=CARTESIAN_POINT('Ctrl Pts',(-62.0672816227846,-77.5277871877005,
62.5246413934834));
#207020=CARTESIAN_POINT('Ctrl Pts',(-62.0855140631312,-77.9934688737491,
62.1652578218559));
#207021=CARTESIAN_POINT('Ctrl Pts',(-62.1132208604885,-78.7421310016436,
61.6953605940876));
#207022=CARTESIAN_POINT('Ctrl Pts',(-62.1225699390672,-79.0013151489718,
61.5498747991622));
#207023=CARTESIAN_POINT('Ctrl Pts',(-62.1490053150776,-79.7484642844835,
61.1773832461642));
#207024=CARTESIAN_POINT('Ctrl Pts',(-62.1661982830379,-80.2501233601518,
60.9806122286629));
#207025=CARTESIAN_POINT('Ctrl Pts',(-62.2023613358389,-81.3556147788107,
60.656599334447));
#207026=CARTESIAN_POINT('Ctrl Pts',(-62.2213588160481,-81.9609934442741,
60.5440312316192));
#207027=CARTESIAN_POINT('Ctrl Pts',(-62.255885581863,-83.0515275727582,
60.4537659964282));
#207028=CARTESIAN_POINT('Ctrl Pts',(-62.2711863732942,-83.5323530737995,
60.452129250671));
#207029=CARTESIAN_POINT('Ctrl Pts',(-62.3077598618603,-84.6857142422267,
60.5396914991162));
#207030=CARTESIAN_POINT('Ctrl Pts',(-62.3285833453382,-85.3525521243088,
60.6660772370334));
#207031=CARTESIAN_POINT('Ctrl Pts',(-62.3643327853757,-86.4378214880229,
61.0004153008872));
#207032=CARTESIAN_POINT('Ctrl Pts',(-62.3789269779372,-86.8656055716723,
61.1685795365253));
#207033=CARTESIAN_POINT('Ctrl Pts',(-62.4281880966457,-88.2631528070393,
61.8441065846855));
#207034=CARTESIAN_POINT('Ctrl Pts',(-62.4616915558082,-89.1535935708666,
62.4935761900372));
#207035=CARTESIAN_POINT('Ctrl Pts',(-62.505365522961,-90.0996337652386,
63.4875327634942));
#207036=CARTESIAN_POINT('Ctrl Pts',(-62.5142515770287,-90.2825476536875,
63.6983354789032));
#207037=CARTESIAN_POINT('Ctrl Pts',(-62.5495766311797,-90.9763664269183,
64.5765062365734));
#207038=CARTESIAN_POINT('Ctrl Pts',(-62.5755554219838,-91.4033377225375,
65.3048466540976));
#207039=CARTESIAN_POINT('Ctrl Pts',(-62.602329162019,-91.724183716028,66.0814193573955));
#207040=CARTESIAN_POINT('Origin',(-61.5936228798467,-83.3229197588524,69.5524554490053));
#207041=CARTESIAN_POINT('',(-58.9742739887231,-91.7241837277703,66.0814193858164));
#207042=CARTESIAN_POINT('',(-59.1795703763519,-91.724183709737,66.0814193421689));
#207043=CARTESIAN_POINT('',(-61.5936228798467,-91.7241837160232,66.0814193573838));
#207044=CARTESIAN_POINT('Ctrl Pts',(-58.9742739877562,-91.7241837277819,
66.0814193858445));
#207045=CARTESIAN_POINT('Ctrl Pts',(-58.9908808498526,-91.9257346557453,
66.5692514101137));
#207046=CARTESIAN_POINT('Ctrl Pts',(-59.0076733421077,-92.0844500731938,
67.0738026638248));
#207047=CARTESIAN_POINT('Ctrl Pts',(-59.0627053178923,-92.4564321249842,
68.7556131068187));
#207048=CARTESIAN_POINT('Ctrl Pts',(-59.0995452584485,-92.4820027230901,
69.9613478729627));
#207049=CARTESIAN_POINT('Ctrl Pts',(-59.1763294497039,-92.0644174996969,
72.3194970018555));
#207050=CARTESIAN_POINT('Ctrl Pts',(-59.2134839228635,-91.6230232950485,
73.4484250669953));
#207051=CARTESIAN_POINT('Ctrl Pts',(-59.2798185920197,-90.5099699736407,
75.1843447045194));
#207052=CARTESIAN_POINT('Ctrl Pts',(-59.306794647372,-89.9440543097349,
75.8399395522327));
#207053=CARTESIAN_POINT('Ctrl Pts',(-59.3564437320649,-88.7716315751605,
76.8614591888738));
#207054=CARTESIAN_POINT('Ctrl Pts',(-59.3789666017369,-88.19851752829,77.2556070377854));
#207055=CARTESIAN_POINT('Ctrl Pts',(-59.4103427162114,-87.3288255032696,
77.717439476316));
#207056=CARTESIAN_POINT('Ctrl Pts',(-59.4195600296134,-87.0650332141483,
77.8416552162396));
#207057=CARTESIAN_POINT('Ctrl Pts',(-59.4475024480258,-86.2518958119344,
78.1778092999195));
#207058=CARTESIAN_POINT('Ctrl Pts',(-59.4663513373701,-85.6875172834469,
78.3492898145992));
#207059=CARTESIAN_POINT('Ctrl Pts',(-59.4949052382847,-84.8210363152403,
78.5230831823793));
#207060=CARTESIAN_POINT('Ctrl Pts',(-59.5044493027401,-84.5288673025814,
78.5670108106814));
#207061=CARTESIAN_POINT('Ctrl Pts',(-59.5293097555489,-83.7554968885733,
78.6450096573948));
#207062=CARTESIAN_POINT('Ctrl Pts',(-59.5445018264202,-83.2728265380557,
78.6551561549891));
#207063=CARTESIAN_POINT('Ctrl Pts',(-59.5914450836271,-81.804689052566,
78.5692008948062));
#207064=CARTESIAN_POINT('Ctrl Pts',(-59.6234634814916,-80.8337513441777,
78.3507943668341));
#207065=CARTESIAN_POINT('Ctrl Pts',(-59.6925162025095,-78.8173947877068,
77.5359692864206));
#207066=CARTESIAN_POINT('Ctrl Pts',(-59.7308228499329,-77.8152015027179,
76.8805721756744));
#207067=CARTESIAN_POINT('Ctrl Pts',(-59.7868686029272,-76.5512780269444,
75.644469479372));
#207068=CARTESIAN_POINT('Ctrl Pts',(-59.8053313153152,-76.175373566138,
75.1987234472925));
#207069=CARTESIAN_POINT('Ctrl Pts',(-59.8423698013046,-75.5208578315081,
74.2515572404954));
#207070=CARTESIAN_POINT('Ctrl Pts',(-59.8607019474952,-75.2418141424838,
73.753583441467));
#207071=CARTESIAN_POINT('Ctrl Pts',(-59.8968475291039,-74.7793631392255,
72.7091753358789));
#207072=CARTESIAN_POINT('Ctrl Pts',(-59.9148988032172,-74.5975143782169,
72.1648370032571));
#207073=CARTESIAN_POINT('Ctrl Pts',(-59.9513262035449,-74.3403231442999,
71.0563865840875));
#207074=CARTESIAN_POINT('Ctrl Pts',(-59.9695581868124,-74.2641988474479,
70.4950264196888));
#207075=CARTESIAN_POINT('Ctrl Pts',(-59.9998818133706,-74.224344760623,
69.5369023379722));
#207076=CARTESIAN_POINT('Ctrl Pts',(-60.0122259831535,-74.2335529429989,
69.1429180003753));
#207077=CARTESIAN_POINT('Ctrl Pts',(-60.0426641604663,-74.3184251587381,
68.1843228824391));
#207078=CARTESIAN_POINT('Ctrl Pts',(-60.060855089267,-74.4216222036621,
67.6238288611412));
#207079=CARTESIAN_POINT('Ctrl Pts',(-60.0978940207412,-74.7373164118713,
66.5085492889639));
#207080=CARTESIAN_POINT('Ctrl Pts',(-60.1163146125923,-74.9530998485078,
65.9574494391708));
#207081=CARTESIAN_POINT('Ctrl Pts',(-60.1442198768137,-75.3551635481451,
65.1670227820366));
#207082=CARTESIAN_POINT('Ctrl Pts',(-60.1535820856437,-75.5023665671669,
64.9096002063616));
#207083=CARTESIAN_POINT('Ctrl Pts',(-60.1806193446042,-75.9603345015432,
64.192498313495));
#207084=CARTESIAN_POINT('Ctrl Pts',(-60.1984003506664,-76.300928257504,
63.7534514050396));
#207085=CARTESIAN_POINT('Ctrl Pts',(-60.2365623844928,-77.1290347265396,
62.8667173025896));
#207086=CARTESIAN_POINT('Ctrl Pts',(-60.2570033883428,-77.6296757264703,
62.4355541959524));
#207087=CARTESIAN_POINT('Ctrl Pts',(-60.2949589766168,-78.6167558613648,
61.7568137992786));
#207088=CARTESIAN_POINT('Ctrl Pts',(-60.3122068434638,-79.0873098862241,
61.4914614798484));
#207089=CARTESIAN_POINT('Ctrl Pts',(-60.3480980487767,-80.1284570197993,
61.0208166362793));
#207090=CARTESIAN_POINT('Ctrl Pts',(-60.3667716031957,-80.7017004728976,
60.8276249116441));
#207091=CARTESIAN_POINT('Ctrl Pts',(-60.4009777322731,-81.7584940110668,
60.5851205443442));
#207092=CARTESIAN_POINT('Ctrl Pts',(-60.4163005490733,-82.2349326014184,
60.5149335199254));
#207093=CARTESIAN_POINT('Ctrl Pts',(-60.4544002950272,-83.4363346628987,
60.4343638274107));
#207094=CARTESIAN_POINT('Ctrl Pts',(-60.4766346105869,-84.1611907855992,
60.4722703326291));
#207095=CARTESIAN_POINT('Ctrl Pts',(-60.5140715722796,-85.3315789469087,
60.6749332528192));
#207096=CARTESIAN_POINT('Ctrl Pts',(-60.5288590170102,-85.7825443673847,
60.7891596011839));
#207097=CARTESIAN_POINT('Ctrl Pts',(-60.5624892309632,-86.788494743557,
61.1277659142991));
#207098=CARTESIAN_POINT('Ctrl Pts',(-60.5809396243979,-87.334063076315,
61.373437511639));
#207099=CARTESIAN_POINT('Ctrl Pts',(-60.6160219879483,-88.3040433443999,
61.9307745522433));
#207100=CARTESIAN_POINT('Ctrl Pts',(-60.63256472669,-88.7332559569293,62.2292140725272));
#207101=CARTESIAN_POINT('Ctrl Pts',(-60.6868217004815,-90.0451762610977,
63.320015613818));
#207102=CARTESIAN_POINT('Ctrl Pts',(-60.7231579565889,-90.7991641832008,
64.2479484416805));
#207103=CARTESIAN_POINT('Ctrl Pts',(-60.7701879850551,-91.4900992769741,
65.5510848102547));
#207104=CARTESIAN_POINT('Ctrl Pts',(-60.7794317860479,-91.6136014806138,
65.8137671278693));
#207105=CARTESIAN_POINT('Ctrl Pts',(-60.7885639123434,-91.7241837160232,
66.0814193573838));
#207106=CARTESIAN_POINT('Ctrl Pts',(-60.9932785231031,-91.7241837160232,
66.0814193573838));
#207107=CARTESIAN_POINT('Ctrl Pts',(-60.9836585589429,-91.609266325186,
65.8032743573871));
#207108=CARTESIAN_POINT('Ctrl Pts',(-60.9741358332696,-91.4803992918137,
65.5305050330448));
#207109=CARTESIAN_POINT('Ctrl Pts',(-60.9270802992573,-90.7781059031341,
64.2178840124118));
#207110=CARTESIAN_POINT('Ctrl Pts',(-60.8888532890121,-90.018802447874,
63.2912571558181));
#207111=CARTESIAN_POINT('Ctrl Pts',(-60.8322357517563,-88.6403280280915,
62.1555791049752));
#207112=CARTESIAN_POINT('Ctrl Pts',(-60.8132185571498,-88.1411463147246,
61.8211363998287));
#207113=CARTESIAN_POINT('Ctrl Pts',(-60.7750249259248,-87.0963265378314,
61.2618727704026));
#207114=CARTESIAN_POINT('Ctrl Pts',(-60.7561225370917,-86.5544443622508,
61.0360228755365));
#207115=CARTESIAN_POINT('Ctrl Pts',(-60.7218376982587,-85.5228478084517,
60.7188124525034));
#207116=CARTESIAN_POINT('Ctrl Pts',(-60.7062001797163,-85.0400554744152,
60.6124121799593));
#207117=CARTESIAN_POINT('Ctrl Pts',(-60.6738110596239,-84.0410208393284,
60.476189995232));
#207118=CARTESIAN_POINT('Ctrl Pts',(-60.6570942186559,-83.5260382871465,
60.4500930059206));
#207119=CARTESIAN_POINT('Ctrl Pts',(-60.6240319181291,-82.4963631963837,
60.485375516262));
#207120=CARTESIAN_POINT('Ctrl Pts',(-60.607805525829,-81.9835353091829,
60.5468356453021));
#207121=CARTESIAN_POINT('Ctrl Pts',(-60.5818679147074,-81.1874236998583,
60.7117845706479));
#207122=CARTESIAN_POINT('Ctrl Pts',(-60.572331013593,-80.8992978184601,
60.7863924901967));
#207123=CARTESIAN_POINT('Ctrl Pts',(-60.5438463993114,-80.0556438168937,
61.0496319669537));
#207124=CARTESIAN_POINT('Ctrl Pts',(-60.5248819043189,-79.5141369426373,
61.2780195740827));
#207125=CARTESIAN_POINT('Ctrl Pts',(-60.4896608844245,-78.5388903663837,
61.805500198871));
#207126=CARTESIAN_POINT('Ctrl Pts',(-60.4731466910582,-78.1016574196566,
62.0931880403867));
#207127=CARTESIAN_POINT('Ctrl Pts',(-60.4428068374976,-77.3590790196944,
62.6792229000049));
#207128=CARTESIAN_POINT('Ctrl Pts',(-60.4291140884938,-77.0453418691813,
62.9645320115567));
#207129=CARTESIAN_POINT('Ctrl Pts',(-60.3973440712632,-76.3625499688621,
63.6786809142309));
#207130=CARTESIAN_POINT('Ctrl Pts',(-60.3796211692993,-76.0113096533257,
64.1221391847533));
#207131=CARTESIAN_POINT('Ctrl Pts',(-60.3401220321253,-75.332753475204,
65.1651220201054));
#207132=CARTESIAN_POINT('Ctrl Pts',(-60.3182288784822,-75.0271241498172,
65.7747303146124));
#207133=CARTESIAN_POINT('Ctrl Pts',(-60.2784676608396,-74.5982230652185,
66.9400288655615));
#207134=CARTESIAN_POINT('Ctrl Pts',(-60.2609024862143,-74.4534436343785,
67.4842435611604));
#207135=CARTESIAN_POINT('Ctrl Pts',(-60.2222462640891,-74.2500905920886,
68.6880250243619));
#207136=CARTESIAN_POINT('Ctrl Pts',(-60.2010843280752,-74.2113042729708,
69.3477242652848));
#207137=CARTESIAN_POINT('Ctrl Pts',(-60.1621998069781,-74.2720875747106,
70.5650207586457));
#207138=CARTESIAN_POINT('Ctrl Pts',(-60.1447617133219,-74.3516232954627,
71.1204776505044));
#207139=CARTESIAN_POINT('Ctrl Pts',(-60.1091224794885,-74.6141256441802,
72.2190288625099));
#207140=CARTESIAN_POINT('Ctrl Pts',(-60.0909495045359,-74.7982626855029,
72.7593104905246));
#207141=CARTESIAN_POINT('Ctrl Pts',(-60.0546575572412,-75.2646446818146,
73.7970213248205));
#207142=CARTESIAN_POINT('Ctrl Pts',(-60.0369334088695,-75.5456277540114,
74.2922729755054));
#207143=CARTESIAN_POINT('Ctrl Pts',(-60.0008984975686,-76.2031526972008,
75.2335343312809));
#207144=CARTESIAN_POINT('Ctrl Pts',(-59.9825249930449,-76.5800517774161,
75.67613568403));
#207145=CARTESIAN_POINT('Ctrl Pts',(-59.926268923334,-77.8486967939239,
76.9057230471662));
#207146=CARTESIAN_POINT('Ctrl Pts',(-59.88990758121,-78.8544070034193,77.5568326873641));
#207147=CARTESIAN_POINT('Ctrl Pts',(-59.8225565777777,-80.8228582751085,
78.3415586035183));
#207148=CARTESIAN_POINT('Ctrl Pts',(-59.7938700528801,-81.7369363317453,
78.5515283314669));
#207149=CARTESIAN_POINT('Ctrl Pts',(-59.7478086174076,-83.1932161265221,
78.656903910119));
#207150=CARTESIAN_POINT('Ctrl Pts',(-59.7309667738328,-83.7218631284607,
78.6490835953509));
#207151=CARTESIAN_POINT('Ctrl Pts',(-59.7050208595486,-84.5403896371845,
78.5654554400883));
#207152=CARTESIAN_POINT('Ctrl Pts',(-59.6958264696521,-84.8323098346971,
78.5211869299153));
#207153=CARTESIAN_POINT('Ctrl Pts',(-59.6682566882164,-85.6983688636324,
78.346364362918));
#207154=CARTESIAN_POINT('Ctrl Pts',(-59.6498248806209,-86.262504943039,
78.1741966346491));
#207155=CARTESIAN_POINT('Ctrl Pts',(-59.6218885903569,-87.075242244736,
77.8370407378287));
#207156=CARTESIAN_POINT('Ctrl Pts',(-59.61260781306,-87.3389308468233,77.7124758292482));
#207157=CARTESIAN_POINT('Ctrl Pts',(-59.581961560223,-88.1937331512077,
77.2571860473787));
#207158=CARTESIAN_POINT('Ctrl Pts',(-59.5610948666435,-88.7538620560443,
76.8731497224859));
#207159=CARTESIAN_POINT('Ctrl Pts',(-59.512533068949,-89.9186687394956,
75.8666562474787));
#207160=CARTESIAN_POINT('Ctrl Pts',(-59.4850147781052,-90.4876529920233,
75.2128126897288));
#207161=CARTESIAN_POINT('Ctrl Pts',(-59.4204113195225,-91.6076307263067,
73.4809461880866));
#207162=CARTESIAN_POINT('Ctrl Pts',(-59.3821093262288,-92.0533420830907,
72.3540966318594));
#207163=CARTESIAN_POINT('Ctrl Pts',(-59.3068946430571,-92.4800760647086,
69.9991812669454));
#207164=CARTESIAN_POINT('Ctrl Pts',(-59.2686837525913,-92.4595902367898,
68.7946120083655));
#207165=CARTESIAN_POINT('Ctrl Pts',(-59.2139666988862,-92.0924482424603,
67.0993407838807));
#207166=CARTESIAN_POINT('Ctrl Pts',(-59.1969005346458,-91.9308425416561,
66.5816144831256));
#207167=CARTESIAN_POINT('Ctrl Pts',(-59.1795703768785,-91.7241837097306,
66.0814193421533));
#207168=CARTESIAN_POINT('Origin',(-61.5936228798467,-83.3229197588524,69.5524554490053));
#207169=CARTESIAN_POINT('',(-57.1603612091034,-91.7241837160232,66.0814193573838));
#207170=CARTESIAN_POINT('',(-57.3654750299524,-91.7241837160232,66.0814193573838));
#207171=CARTESIAN_POINT('',(-61.5936228798467,-91.7241837160232,66.0814193573838));
#207172=CARTESIAN_POINT('Ctrl Pts',(-57.1603612091034,-91.7241837160232,
66.0814193573838));
#207173=CARTESIAN_POINT('Ctrl Pts',(-57.1643075550946,-91.7714348510752,
66.1957855717848));
#207174=CARTESIAN_POINT('Ctrl Pts',(-57.1682592739096,-91.8163636829924,
66.3111480666542));
#207175=CARTESIAN_POINT('Ctrl Pts',(-57.201192711216,-92.1711758057006,
67.2803207234912));
#207176=CARTESIAN_POINT('Ctrl Pts',(-57.2292447649847,-92.3538340628692,
68.1752032550547));
#207177=CARTESIAN_POINT('Ctrl Pts',(-57.2738634620999,-92.4263624913974,
69.5754015843189));
#207178=CARTESIAN_POINT('Ctrl Pts',(-57.2897494762442,-92.4116774206205,
70.0698297406882));
#207179=CARTESIAN_POINT('Ctrl Pts',(-57.3148029097305,-92.3243440725679,
70.8524170008992));
#207180=CARTESIAN_POINT('Ctrl Pts',(-57.3240386954911,-92.2776603112734,
71.1424750414258));
#207181=CARTESIAN_POINT('Ctrl Pts',(-57.3708522755525,-91.9708346583543,
72.5961177973874));
#207182=CARTESIAN_POINT('Ctrl Pts',(-57.4091414904654,-91.4976074282449,
73.7027303808055));
#207183=CARTESIAN_POINT('Ctrl Pts',(-57.4842609382672,-90.1556475234844,
75.6635087704191));
#207184=CARTESIAN_POINT('Ctrl Pts',(-57.5224045134595,-89.3024498332601,
76.5005747389649));
#207185=CARTESIAN_POINT('Ctrl Pts',(-57.5764701266048,-87.8772559016594,
77.4365450251894));
#207186=CARTESIAN_POINT('Ctrl Pts',(-57.5929747042321,-87.4179231028032,
77.6846008445442));
#207187=CARTESIAN_POINT('Ctrl Pts',(-57.6258046815346,-86.4808254539663,
78.0910343755753));
#207188=CARTESIAN_POINT('Ctrl Pts',(-57.6420496562794,-86.0061165722681,
78.2518895028104));
#207189=CARTESIAN_POINT('Ctrl Pts',(-57.6738803754007,-85.0410300778121,
78.4923480219708));
#207190=CARTESIAN_POINT('Ctrl Pts',(-57.689444972188,-84.552521939159,78.5725256397523));
#207191=CARTESIAN_POINT('Ctrl Pts',(-57.7147177339823,-83.7631994761432,
78.6367335376223));
#207192=CARTESIAN_POINT('Ctrl Pts',(-57.7242681745868,-83.4654719202352,
78.6462792625143));
#207193=CARTESIAN_POINT('Ctrl Pts',(-57.7527572734999,-82.582197358887,
78.6312057289093));
#207194=CARTESIAN_POINT('Ctrl Pts',(-57.7717005025127,-81.9989056263173,
78.564634914755));
#207195=CARTESIAN_POINT('Ctrl Pts',(-57.8063909285601,-80.9316833242889,
78.3369232520953));
#207196=CARTESIAN_POINT('Ctrl Pts',(-57.8223966429801,-80.4469472315054,
78.1903756694889));
#207197=CARTESIAN_POINT('Ctrl Pts',(-57.8551886855639,-79.4974135420679,
77.8144641304721));
#207198=CARTESIAN_POINT('Ctrl Pts',(-57.8719273494801,-79.0349383175548,
77.5841735694151));
#207199=CARTESIAN_POINT('Ctrl Pts',(-57.9053131805234,-78.1458942510517,
77.0426909799553));
#207200=CARTESIAN_POINT('Ctrl Pts',(-57.9218204048192,-77.7218183928645,
76.7310966467465));
#207201=CARTESIAN_POINT('Ctrl Pts',(-57.9480233051002,-77.1037071145463,
76.1886444468371));
#207202=CARTESIAN_POINT('Ctrl Pts',(-57.9575365520924,-76.8901308045856,
75.9818282628259));
#207203=CARTESIAN_POINT('Ctrl Pts',(-57.9860324136145,-76.2849042509406,
75.335355439972));
#207204=CARTESIAN_POINT('Ctrl Pts',(-58.0050161401071,-75.9253960484828,
74.8677404488049));
#207205=CARTESIAN_POINT('Ctrl Pts',(-58.0424643676744,-75.2991679759306,
73.8653373491247));
#207206=CARTESIAN_POINT('Ctrl Pts',(-58.0611869392659,-75.0347731329829,
73.332424320369));
#207207=CARTESIAN_POINT('Ctrl Pts',(-58.0994464373814,-74.6113738282244,
72.2166936412776));
#207208=CARTESIAN_POINT('Ctrl Pts',(-58.1187827973433,-74.4545756367208,
71.6361270713852));
#207209=CARTESIAN_POINT('Ctrl Pts',(-58.1539312084072,-74.2720434637819,
70.5390498261329));
#207210=CARTESIAN_POINT('Ctrl Pts',(-58.1700167669714,-74.2308340851803,
70.0275421600996));
#207211=CARTESIAN_POINT('Ctrl Pts',(-58.2025959350043,-74.2350161326039,
69.0045550257246));
#207212=CARTESIAN_POINT('Ctrl Pts',(-58.2190306716271,-74.2801456199829,
68.4949023500349));
#207213=CARTESIAN_POINT('Ctrl Pts',(-58.2526122598165,-74.4612172411427,
67.4559438035145));
#207214=CARTESIAN_POINT('Ctrl Pts',(-58.2695416633615,-74.6024966871704,
66.9296025601453));
#207215=CARTESIAN_POINT('Ctrl Pts',(-58.296026273235,-74.8917708654786,
66.1418450920097));
#207216=CARTESIAN_POINT('Ctrl Pts',(-58.3053899012604,-75.0070129209366,
65.8697626281372));
#207217=CARTESIAN_POINT('Ctrl Pts',(-58.3338234479444,-75.3946205761399,
65.0660544878458));
#207218=CARTESIAN_POINT('Ctrl Pts',(-58.3528949851174,-75.7062949711908,
64.5551796005247));
#207219=CARTESIAN_POINT('Ctrl Pts',(-58.3882935170328,-76.385959503553,
63.6541018030826));
#207220=CARTESIAN_POINT('Ctrl Pts',(-58.4048943856861,-76.7427391072376,
63.258552577647));
#207221=CARTESIAN_POINT('Ctrl Pts',(-58.4346675241699,-77.4307444764585,
62.6186240690943));
#207222=CARTESIAN_POINT('Ctrl Pts',(-58.4476894679638,-77.7478164010396,
62.3612130182685));
#207223=CARTESIAN_POINT('Ctrl Pts',(-58.4785830619273,-78.5430493842177,
61.7999155307737));
#207224=CARTESIAN_POINT('Ctrl Pts',(-58.4960997564441,-79.0344094502668,
61.517673738298));
#207225=CARTESIAN_POINT('Ctrl Pts',(-58.5227363605971,-79.8073762245133,
61.1649009892014));
#207226=CARTESIAN_POINT('Ctrl Pts',(-58.5316852592252,-80.0713441764505,
61.0590832791401));
#207227=CARTESIAN_POINT('Ctrl Pts',(-58.5499140211205,-80.6151976913719,
60.870143207617));
#207228=CARTESIAN_POINT('Ctrl Pts',(-58.5591861949119,-80.8950037782894,
60.7877804476541));
#207229=CARTESIAN_POINT('Ctrl Pts',(-58.586539844,-81.7320777528774,60.5845505790919));
#207230=CARTESIAN_POINT('Ctrl Pts',(-58.6042602292198,-82.2972917414937,
60.5024726813504));
#207231=CARTESIAN_POINT('Ctrl Pts',(-58.6402273616741,-83.4466785572209,
60.4446832682405));
#207232=CARTESIAN_POINT('Ctrl Pts',(-58.658555460935,-84.028352856961,60.4712010325149));
#207233=CARTESIAN_POINT('Ctrl Pts',(-58.7072359978959,-85.5457853012357,
60.6871252311085));
#207234=CARTESIAN_POINT('Ctrl Pts',(-58.7364641284295,-86.4611958779166,
60.9683745048571));
#207235=CARTESIAN_POINT('Ctrl Pts',(-58.7832132337006,-87.7898683092187,
61.6181193945942));
#207236=CARTESIAN_POINT('Ctrl Pts',(-58.8000677246322,-88.2424648842144,
61.8905109661702));
#207237=CARTESIAN_POINT('Ctrl Pts',(-58.8318378019263,-89.0585758868051,
62.4839532076096));
#207238=CARTESIAN_POINT('Ctrl Pts',(-58.8467750324505,-89.4251153555413,
62.7978504449456));
#207239=CARTESIAN_POINT('Ctrl Pts',(-58.8797498752602,-90.1657642790579,
63.5418471455463));
#207240=CARTESIAN_POINT('Ctrl Pts',(-58.8978198322272,-90.5278717659411,
63.9810474409389));
#207241=CARTESIAN_POINT('Ctrl Pts',(-58.9338810151096,-91.1638608214093,
64.919040118221));
#207242=CARTESIAN_POINT('Ctrl Pts',(-58.9514883722586,-91.436767839919,
65.4155040937725));
#207243=CARTESIAN_POINT('Ctrl Pts',(-58.9709199352701,-91.6830246161798,
65.9830269473587));
#207244=CARTESIAN_POINT('Ctrl Pts',(-58.9725963370137,-91.7038227431489,
66.0321378446976));
#207245=CARTESIAN_POINT('Ctrl Pts',(-58.9742739877562,-91.7241837277819,
66.0814193858445));
#207246=CARTESIAN_POINT('Ctrl Pts',(-59.1795703768785,-91.7241837097306,
66.0814193421533));
#207247=CARTESIAN_POINT('Ctrl Pts',(-59.1783553620991,-91.7096948898098,
66.0463507353326));
#207248=CARTESIAN_POINT('Ctrl Pts',(-59.1771393902312,-91.6949846120067,
66.0113682909168));
#207249=CARTESIAN_POINT('Ctrl Pts',(-59.1580018344277,-91.4601655241754,
65.4625917852046));
#207250=CARTESIAN_POINT('Ctrl Pts',(-59.1399701168292,-91.1933449814746,
64.9700791141866));
#207251=CARTESIAN_POINT('Ctrl Pts',(-59.1045759997665,-90.5733648370307,
64.0414382185356));
#207252=CARTESIAN_POINT('Ctrl Pts',(-59.0870138155532,-90.2217326564725,
63.6071511480886));
#207253=CARTESIAN_POINT('Ctrl Pts',(-59.0544365075591,-89.5121086859036,
62.8790740543585));
#207254=CARTESIAN_POINT('Ctrl Pts',(-59.039582980177,-89.1672431070907,
62.5750662830142));
#207255=CARTESIAN_POINT('Ctrl Pts',(-59.0012843085679,-88.2159243714361,
61.8566666686836));
#207256=CARTESIAN_POINT('Ctrl Pts',(-58.978371995284,-87.5796644716814,
61.4872967016084));
#207257=CARTESIAN_POINT('Ctrl Pts',(-58.9401170374322,-86.4836038562859,
61.0171976259968));
#207258=CARTESIAN_POINT('Ctrl Pts',(-58.9252306844584,-86.0480941308018,
60.8683337116299));
#207259=CARTESIAN_POINT('Ctrl Pts',(-58.8910256424108,-85.0202121023796,
60.6019676932172));
#207260=CARTESIAN_POINT('Ctrl Pts',(-58.8720962206822,-84.4236506082263,
60.5092024127063));
#207261=CARTESIAN_POINT('Ctrl Pts',(-58.8212772660278,-82.8338578869889,
60.4217304057643));
#207262=CARTESIAN_POINT('Ctrl Pts',(-58.7892143585532,-81.8431288331944,
60.5291775535275));
#207263=CARTESIAN_POINT('Ctrl Pts',(-58.7201202500558,-79.7466171406805,
61.1117228620778));
#207264=CARTESIAN_POINT('Ctrl Pts',(-58.6818139625381,-78.6770244949825,
61.6498248259125));
#207265=CARTESIAN_POINT('Ctrl Pts',(-58.6257691208861,-77.2819454248588,
62.7352552474275));
#207266=CARTESIAN_POINT('Ctrl Pts',(-58.6073090915348,-76.8582525937609,
63.1356291190726));
#207267=CARTESIAN_POINT('Ctrl Pts',(-58.5702707919224,-76.1011351515366,
64.0027244590353));
#207268=CARTESIAN_POINT('Ctrl Pts',(-58.5519348061948,-75.7676859893879,
64.4659884950895));
#207269=CARTESIAN_POINT('Ctrl Pts',(-58.5157889379326,-75.190422212679,
65.4513000243091));
#207270=CARTESIAN_POINT('Ctrl Pts',(-58.497741483714,-74.9483624597392,
65.9714250761848));
#207271=CARTESIAN_POINT('Ctrl Pts',(-58.4613134672743,-74.567679016852,
67.0435448969656));
#207272=CARTESIAN_POINT('Ctrl Pts',(-58.4430756291629,-74.4286308850337,
67.5927330918716));
#207273=CARTESIAN_POINT('Ctrl Pts',(-58.4010649321468,-74.2239027487931,
68.9050171394925));
#207274=CARTESIAN_POINT('Ctrl Pts',(-58.3771770643042,-74.2016623822086,
69.6705738966716));
#207275=CARTESIAN_POINT('Ctrl Pts',(-58.3434224302482,-74.3035131501736,
70.7208207861201));
#207276=CARTESIAN_POINT('Ctrl Pts',(-58.3340499251273,-74.345746037725,
71.0102364882732));
#207277=CARTESIAN_POINT('Ctrl Pts',(-58.3049108446301,-74.5213858130833,
71.9083465114184));
#207278=CARTESIAN_POINT('Ctrl Pts',(-58.2855881226413,-74.7034237654515,
72.5056765036959));
#207279=CARTESIAN_POINT('Ctrl Pts',(-58.2498238969358,-75.1426564471019,
73.5489337250016));
#207280=CARTESIAN_POINT('Ctrl Pts',(-58.2335687564081,-75.3792911537745,
74.0007476823246));
#207281=CARTESIAN_POINT('Ctrl Pts',(-58.1982641757421,-75.9740987793751,
74.9360718971259));
#207282=CARTESIAN_POINT('Ctrl Pts',(-58.1796408263271,-76.3449207690453,
75.4087366445883));
#207283=CARTESIAN_POINT('Ctrl Pts',(-58.151516698401,-76.9647666172548,
76.0556234234973));
#207284=CARTESIAN_POINT('Ctrl Pts',(-58.142166017743,-77.1803356554583,
76.2596131085063));
#207285=CARTESIAN_POINT('Ctrl Pts',(-58.1148962857639,-77.8331707004816,
76.8194639086075));
#207286=CARTESIAN_POINT('Ctrl Pts',(-58.0968869088407,-78.2940299198404,
77.1456785032234));
#207287=CARTESIAN_POINT('Ctrl Pts',(-58.066637450632,-79.1300272859004,
77.6277430013837));
#207288=CARTESIAN_POINT('Ctrl Pts',(-58.0541568621049,-79.4908505879974,
77.8050831100247));
#207289=CARTESIAN_POINT('Ctrl Pts',(-58.0244492458845,-80.3665371628115,
78.1656188149886));
#207290=CARTESIAN_POINT('Ctrl Pts',(-58.0071473291945,-80.8885205324986,
78.3274466919687));
#207291=CARTESIAN_POINT('Ctrl Pts',(-57.9712424764974,-81.9945996455441,
78.5640006805048));
#207292=CARTESIAN_POINT('Ctrl Pts',(-57.9530557583684,-82.5778544662228,
78.6308509025772));
#207293=CARTESIAN_POINT('Ctrl Pts',(-57.9254352831612,-83.4611402262249,
78.6463464595879));
#207294=CARTESIAN_POINT('Ctrl Pts',(-57.9160908551431,-83.7588790637174,
78.6369420233036));
#207295=CARTESIAN_POINT('Ctrl Pts',(-57.8911014063756,-84.54722380647,78.5731907277357));
#207296=CARTESIAN_POINT('Ctrl Pts',(-57.8753600356538,-85.0347775998973,
78.4934914589621));
#207297=CARTESIAN_POINT('Ctrl Pts',(-57.8438473079412,-86.0050026187064,
78.2525863985289));
#207298=CARTESIAN_POINT('Ctrl Pts',(-57.8281804590448,-86.4854956150931,
78.0896660951154));
#207299=CARTESIAN_POINT('Ctrl Pts',(-57.796090447364,-87.4237074244127,
77.6814070912102));
#207300=CARTESIAN_POINT('Ctrl Pts',(-57.7797091837313,-87.879057086696,
77.435216223302));
#207301=CARTESIAN_POINT('Ctrl Pts',(-57.7256290096773,-89.3009349475064,
76.5019029960134));
#207302=CARTESIAN_POINT('Ctrl Pts',(-57.6893062427029,-90.1544163486836,
75.6649122163779));
#207303=CARTESIAN_POINT('Ctrl Pts',(-57.6135547941334,-91.496853693898,
73.7042292352895));
#207304=CARTESIAN_POINT('Ctrl Pts',(-57.5768874335455,-91.9702984067784,
72.5976583239647));
#207305=CARTESIAN_POINT('Ctrl Pts',(-57.5293772120705,-92.2773810073057,
71.1440437792263));
#207306=CARTESIAN_POINT('Ctrl Pts',(-57.5199805450081,-92.3241136417869,
70.8540086098186));
#207307=CARTESIAN_POINT('Ctrl Pts',(-57.4950210105062,-92.411628831952,
70.0710582791185));
#207308=CARTESIAN_POINT('Ctrl Pts',(-57.4795946638747,-92.4263817599483,
69.5762355380885));
#207309=CARTESIAN_POINT('Ctrl Pts',(-57.4351904996613,-92.3538893553277,
68.1754221232929));
#207310=CARTESIAN_POINT('Ctrl Pts',(-57.4058892022752,-92.1711981468918,
67.2803188469568));
#207311=CARTESIAN_POINT('Ctrl Pts',(-57.3732874320217,-91.8163112081297,
66.3110133090398));
#207312=CARTESIAN_POINT('Ctrl Pts',(-57.3693826819263,-91.7714071541859,
66.1957185344876));
#207313=CARTESIAN_POINT('Ctrl Pts',(-57.3654750299524,-91.7241837160232,
66.0814193573838));
#207314=CARTESIAN_POINT('Origin',(-64.4265543961493,-83.3237128444373,69.5530424137804));
#207315=CARTESIAN_POINT('',(-64.4174334691588,-91.7227797420331,66.0829140514164));
#207316=CARTESIAN_POINT('',(-64.5675364832717,-91.7227797420325,66.082914051415));
#207317=CARTESIAN_POINT('',(-64.4265543961493,-91.7227797420325,66.082914051415));
#207318=CARTESIAN_POINT('',(-64.4174351716144,-91.722800105991,66.0829633405634));
#207319=CARTESIAN_POINT('Ctrl Pts',(-64.4174351716144,-91.722800105991,
66.0829633405634));
#207320=CARTESIAN_POINT('Ctrl Pts',(-64.4174346041292,-91.7227933180531,
66.0829469108273));
#207321=CARTESIAN_POINT('Ctrl Pts',(-64.417434036644,-91.7227865300673,
66.0829304811121));
#207322=CARTESIAN_POINT('Ctrl Pts',(-64.4174334691588,-91.7227797420337,
66.0829140514177));
#207323=CARTESIAN_POINT('',(-64.5666618780602,-92.3407155670729,70.6707464084894));
#207324=CARTESIAN_POINT('Ctrl Pts',(-64.5657843992066,-92.3423880036114,
70.6709037535128));
#207325=CARTESIAN_POINT('Ctrl Pts',(-64.5410292714247,-92.4385150622132,
69.895370434019));
#207326=CARTESIAN_POINT('Ctrl Pts',(-64.5157599537561,-92.4342089172065,
69.1106652271105));
#207327=CARTESIAN_POINT('Ctrl Pts',(-64.4664991786972,-92.2249846832541,
67.5621750022409));
#207328=CARTESIAN_POINT('Ctrl Pts',(-64.4423690633479,-92.0210452715925,
66.8048452107943));
#207329=CARTESIAN_POINT('Ctrl Pts',(-64.4174351716144,-91.722800105991,
66.0829633405634));
#207330=CARTESIAN_POINT('Origin',(-64.5675364832709,-83.3237128444373,69.5530424137804));
#207331=CARTESIAN_POINT('Origin',(-27.5423496375577,-74.9965420974961,72.9903965241317));
#207332=CARTESIAN_POINT('',(-30.7042591052869,-85.9391496438337,68.4693880411367));
#207333=CARTESIAN_POINT('',(-31.000413750398,-85.9391496391482,68.4693880297961));
#207334=CARTESIAN_POINT('',(-27.5423496375574,-85.9391496391482,68.4693880297962));
#207335=CARTESIAN_POINT('',(-32.4074704173708,-83.5021837654764,64.7498540653718));
#207336=CARTESIAN_POINT('Ctrl Pts',(-30.7042591049895,-85.9391496438364,
68.4693880411434));
#207337=CARTESIAN_POINT('Ctrl Pts',(-30.7071432045293,-85.9845654573861,
68.5793120605169));
#207338=CARTESIAN_POINT('Ctrl Pts',(-30.7100298765835,-86.0283279638993,
68.6899278133005));
#207339=CARTESIAN_POINT('Ctrl Pts',(-30.7314903820352,-86.3407926437295,
69.5159082856428));
#207340=CARTESIAN_POINT('Ctrl Pts',(-30.7502951478004,-86.5413372287112,
70.2551118645619));
#207341=CARTESIAN_POINT('Ctrl Pts',(-30.7880170308652,-86.8001841891141,
71.7796052353538));
#207342=CARTESIAN_POINT('Ctrl Pts',(-30.8067253105562,-86.85437986065,72.5618279359104));
#207343=CARTESIAN_POINT('Ctrl Pts',(-30.8440099841418,-86.8087314383416,
74.0910619682391));
#207344=CARTESIAN_POINT('Ctrl Pts',(-30.8623820857554,-86.7156689921332,
74.8346731455419));
#207345=CARTESIAN_POINT('Ctrl Pts',(-30.8896034539907,-86.4706684462532,
75.9346034566644));
#207346=CARTESIAN_POINT('Ctrl Pts',(-30.8987267060841,-86.3705077421378,
76.3005076268647));
#207347=CARTESIAN_POINT('Ctrl Pts',(-30.9264312686469,-86.0155656347624,
77.3889953031016));
#207348=CARTESIAN_POINT('Ctrl Pts',(-30.9452013262935,-85.7080997144869,
78.0922659739933));
#207349=CARTESIAN_POINT('Ctrl Pts',(-30.9827961460176,-84.9539398590874,
79.4434068326821));
#207350=CARTESIAN_POINT('Ctrl Pts',(-31.0014229555361,-84.5063398186325,
80.0865127085207));
#207351=CARTESIAN_POINT('Ctrl Pts',(-31.0385706158449,-83.5129783442073,
81.2493039530921));
#207352=CARTESIAN_POINT('Ctrl Pts',(-31.0568842446479,-82.9745504758854,
81.7705235161812));
#207353=CARTESIAN_POINT('Ctrl Pts',(-31.0840397115793,-82.0940878563685,
82.4745480719511));
#207354=CARTESIAN_POINT('Ctrl Pts',(-31.0931509110187,-81.7863701512867,
82.6972251189293));
#207355=CARTESIAN_POINT('Ctrl Pts',(-31.1208199817104,-80.8266619512405,
83.3237097366427));
#207356=CARTESIAN_POINT('Ctrl Pts',(-31.1395731345786,-80.1456699616022,
83.6793688182087));
#207357=CARTESIAN_POINT('Ctrl Pts',(-31.1771138492042,-78.7106922779752,
84.2596399069424));
#207358=CARTESIAN_POINT('Ctrl Pts',(-31.1957146935657,-77.9590595147694,
84.4801421190806));
#207359=CARTESIAN_POINT('Ctrl Pts',(-31.2328274046535,-76.4566786725149,
84.7635396778024));
#207360=CARTESIAN_POINT('Ctrl Pts',(-31.2511279433087,-75.7106803106599,
84.83222551326));
#207361=CARTESIAN_POINT('Ctrl Pts',(-31.2782920461113,-74.583085824835,
84.8290501767478));
#207362=CARTESIAN_POINT('Ctrl Pts',(-31.2874188282591,-74.2032428467766,
84.8096749532239));
#207363=CARTESIAN_POINT('Ctrl Pts',(-31.3151023748541,-73.0629186209356,
84.6962828941739));
#207364=CARTESIAN_POINT('Ctrl Pts',(-31.3338604399769,-72.3099991999214,
84.5467432309358));
#207365=CARTESIAN_POINT('Ctrl Pts',(-31.3714457980926,-70.8282886952565,
84.0997228727802));
#207366=CARTESIAN_POINT('Ctrl Pts',(-31.3900936106412,-70.1039676831453,
83.8003081359218));
#207367=CARTESIAN_POINT('Ctrl Pts',(-31.4272909824107,-68.7557241837118,
83.0795160541388));
#207368=CARTESIAN_POINT('Ctrl Pts',(-31.4456248131496,-68.1317858942723,
82.6657916817774));
#207369=CARTESIAN_POINT('Ctrl Pts',(-31.4728631723181,-67.2552269288479,
81.9568297101897));
#207370=CARTESIAN_POINT('Ctrl Pts',(-31.4820258659373,-66.9711566313225,
81.7034942829615));
#207371=CARTESIAN_POINT('Ctrl Pts',(-31.5097623070298,-66.1547977137663,
80.9016098999437));
#207372=CARTESIAN_POINT('Ctrl Pts',(-31.5285400473232,-65.6629099285718,
80.3148103292199));
#207373=CARTESIAN_POINT('Ctrl Pts',(-31.5691339998758,-64.7213617714676,
78.9413008663864));
#207374=CARTESIAN_POINT('Ctrl Pts',(-31.5907096984462,-64.2982909971383,
78.14209755223));
#207375=CARTESIAN_POINT('Ctrl Pts',(-31.6221007543298,-63.8317068315534,
76.9490340134588));
#207376=CARTESIAN_POINT('Ctrl Pts',(-31.6314437729075,-63.7105012176045,
76.5889570999271));
#207377=CARTESIAN_POINT('Ctrl Pts',(-31.6560197121624,-63.4364098802596,
75.6234286894173));
#207378=CARTESIAN_POINT('Ctrl Pts',(-31.671033899748,-63.3137297869777,
75.0106470624251));
#207379=CARTESIAN_POINT('Ctrl Pts',(-31.7047776140326,-63.1497607691003,
73.6343535167224));
#207380=CARTESIAN_POINT('Ctrl Pts',(-31.7235895909336,-63.1328760920988,
72.870715232101));
#207381=CARTESIAN_POINT('Ctrl Pts',(-31.7649870414119,-63.2584445617294,
71.1852285472259));
#207382=CARTESIAN_POINT('Ctrl Pts',(-31.7872985139579,-63.4359874023173,
70.2709946279799));
#207383=CARTESIAN_POINT('Ctrl Pts',(-31.8195010241203,-63.834104995451,
69.0249778555225));
#207384=CARTESIAN_POINT('Ctrl Pts',(-31.8288900534836,-63.9671030559063,
68.6688202399193));
#207385=CARTESIAN_POINT('Ctrl Pts',(-31.8646424176768,-64.5411922652769,
67.3315896995405));
#207386=CARTESIAN_POINT('Ctrl Pts',(-31.8905243214653,-65.0980260916543,
66.4058830810216));
#207387=CARTESIAN_POINT('Ctrl Pts',(-31.926533878651,-66.0122618544706,
65.2696696427136));
#207388=CARTESIAN_POINT('Ctrl Pts',(-31.9359982523297,-66.2667454965785,
64.9830518186356));
#207389=CARTESIAN_POINT('Ctrl Pts',(-31.9585712997858,-66.9120174586244,
64.3236960593822));
#207390=CARTESIAN_POINT('Ctrl Pts',(-31.971650016924,-67.3152732029544,
63.9643594386768));
#207391=CARTESIAN_POINT('Ctrl Pts',(-32.003365826438,-68.3383236131057,
63.1711085216078));
#207392=CARTESIAN_POINT('Ctrl Pts',(-32.022120836258,-68.9779125267418,
62.7665821034246));
#207393=CARTESIAN_POINT('Ctrl Pts',(-32.0616663025437,-70.4166592161241,
62.0386895278778));
#207394=CARTESIAN_POINT('Ctrl Pts',(-32.082393915655,-71.2214500334388,
61.7358906506367));
#207395=CARTESIAN_POINT('Ctrl Pts',(-32.1129240666703,-72.4200404170053,
61.4281167610066));
#207396=CARTESIAN_POINT('Ctrl Pts',(-32.1223373183744,-72.7925622453359,
61.3513610459618));
#207397=CARTESIAN_POINT('Ctrl Pts',(-32.1461140581556,-73.7462800711484,
61.2022903378908));
#207398=CARTESIAN_POINT('Ctrl Pts',(-32.1602847045135,-74.3303337149976,
61.1549087977211));
#207399=CARTESIAN_POINT('Ctrl Pts',(-32.1932425150503,-75.6787881761831,
61.1456775751533));
#207400=CARTESIAN_POINT('Ctrl Pts',(-32.2121296952263,-76.4408037420532,
61.2142799287779));
#207401=CARTESIAN_POINT('Ctrl Pts',(-32.2501673639803,-77.9602656117201,
61.5008568215757));
#207402=CARTESIAN_POINT('Ctrl Pts',(-32.2690290690518,-78.7133570885059,
61.7219242033699));
#207403=CARTESIAN_POINT('Ctrl Pts',(-32.3081937252706,-80.1928731399112,
62.3208321709841));
#207404=CARTESIAN_POINT('Ctrl Pts',(-32.3283181484142,-80.9132149042037,
62.7028091759389));
#207405=CARTESIAN_POINT('Ctrl Pts',(-32.3582225934137,-81.9343183651991,
63.3872432828824));
#207406=CARTESIAN_POINT('Ctrl Pts',(-32.368315847494,-82.2674785607088,
63.6369600267938));
#207407=CARTESIAN_POINT('Ctrl Pts',(-32.3886344788051,-82.9058716239084,
64.1702193176143));
#207408=CARTESIAN_POINT('Ctrl Pts',(-32.3988458781379,-83.2106814012253,
64.4533636048996));
#207409=CARTESIAN_POINT('Ctrl Pts',(-32.4090802221679,-83.4999635122087,
64.7519499557376));
#207410=CARTESIAN_POINT('',(-32.7070018384414,-83.5021837802876,64.7498540510208));
#207411=CARTESIAN_POINT('Origin',(-32.5572357904921,-87.0216635390508,61.3397527098387));
#207412=CARTESIAN_POINT('Ctrl Pts',(-32.7053886803439,-83.5000181996321,
64.7520064024586));
#207413=CARTESIAN_POINT('Ctrl Pts',(-32.6955235775403,-83.2159761503953,
64.4588247562857));
#207414=CARTESIAN_POINT('Ctrl Pts',(-32.6856518412961,-82.9169615816791,
64.180528821265));
#207415=CARTESIAN_POINT('Ctrl Pts',(-32.6657614829319,-82.29100434518,63.6556208137225));
#207416=CARTESIAN_POINT('Ctrl Pts',(-32.6557559698928,-81.9644490912632,
63.4094003432205));
#207417=CARTESIAN_POINT('Ctrl Pts',(-32.6262473116798,-80.9649493872972,
62.7339598779866));
#207418=CARTESIAN_POINT('Ctrl Pts',(-32.607154849764,-80.2606397788824,
62.355282177213));
#207419=CARTESIAN_POINT('Ctrl Pts',(-32.5688597261284,-78.7997606767584,
61.7507608422622));
#207420=CARTESIAN_POINT('Ctrl Pts',(-32.5496201108103,-78.0479541535455,
61.5238032313802));
#207421=CARTESIAN_POINT('Ctrl Pts',(-32.5122282763324,-76.5325989865272,
61.2260547705057));
#207422=CARTESIAN_POINT('Ctrl Pts',(-32.4940526186921,-75.773527879885,
61.1516674041786));
#207423=CARTESIAN_POINT('Ctrl Pts',(-32.4663243767396,-74.6331304636974,
61.1501222475673));
#207424=CARTESIAN_POINT('Ctrl Pts',(-32.457055363824,-74.2538716297711,
61.1678501491844));
#207425=CARTESIAN_POINT('Ctrl Pts',(-32.4296082716827,-73.1326137434058,
61.2744352894935));
#207426=CARTESIAN_POINT('Ctrl Pts',(-32.411791311583,-72.3974612467249,
61.4153044453678));
#207427=CARTESIAN_POINT('Ctrl Pts',(-32.374796683084,-70.9279543662837,
61.8440388478007));
#207428=CARTESIAN_POINT('Ctrl Pts',(-32.3555785938572,-70.1990824339427,
62.1377898829238));
#207429=CARTESIAN_POINT('Ctrl Pts',(-32.3274200720563,-69.1673891423799,
62.6779746001249));
#207430=CARTESIAN_POINT('Ctrl Pts',(-32.3182936882276,-68.8388796045901,
62.8706996944416));
#207431=CARTESIAN_POINT('Ctrl Pts',(-32.2876159549682,-67.7723110391946,
63.5676121662592));
#207432=CARTESIAN_POINT('Ctrl Pts',(-32.2657942501253,-67.082116790659,
64.1393949651531));
#207433=CARTESIAN_POINT('Ctrl Pts',(-32.2348495530599,-66.1980778729565,
65.0586200074079));
#207434=CARTESIAN_POINT('Ctrl Pts',(-32.2256816351913,-65.9468053524882,
65.3465547554137));
#207435=CARTESIAN_POINT('Ctrl Pts',(-32.1982389607735,-65.2397576912024,
66.2405999387672));
#207436=CARTESIAN_POINT('Ctrl Pts',(-32.1798483429023,-64.8277936767111,
66.8788386288624));
#207437=CARTESIAN_POINT('Ctrl Pts',(-32.1431185151747,-64.1366904307863,
68.2153197596488));
#207438=CARTESIAN_POINT('Ctrl Pts',(-32.1252230237423,-63.8572237084219,
68.909547941657));
#207439=CARTESIAN_POINT('Ctrl Pts',(-32.0875515299678,-63.4144500316063,
70.4032333095941));
#207440=CARTESIAN_POINT('Ctrl Pts',(-32.0676381394455,-63.2644413265768,
71.2026424779196));
#207441=CARTESIAN_POINT('Ctrl Pts',(-32.0294863562713,-63.1346017963956,
72.767003299345));
#207442=CARTESIAN_POINT('Ctrl Pts',(-32.011341711395,-63.1446488920153,
73.5272085810173));
#207443=CARTESIAN_POINT('Ctrl Pts',(-31.979994086474,-63.2848186274647,
74.8052249267449));
#207444=CARTESIAN_POINT('Ctrl Pts',(-31.9670359017254,-63.3772231735677,
75.3248116631135));
#207445=CARTESIAN_POINT('Ctrl Pts',(-31.9448400569064,-63.5957909022094,
76.2073889445845));
#207446=CARTESIAN_POINT('Ctrl Pts',(-31.9356130023789,-63.7055382814396,
76.5736075478546));
#207447=CARTESIAN_POINT('Ctrl Pts',(-31.9079011677942,-64.0869137846266,
77.6532568640312));
#207448=CARTESIAN_POINT('Ctrl Pts',(-31.889304744203,-64.4099659372064,
78.3463885023222));
#207449=CARTESIAN_POINT('Ctrl Pts',(-31.8522258789601,-65.1766905039656,
79.6468430874556));
#207450=CARTESIAN_POINT('Ctrl Pts',(-31.8341947001364,-65.6159391447516,
80.2527692827694));
#207451=CARTESIAN_POINT('Ctrl Pts',(-31.7954188454572,-66.6691730346643,
81.4493010415083));
#207452=CARTESIAN_POINT('Ctrl Pts',(-31.7744776665257,-67.2956839939467,
82.0233865657951));
#207453=CARTESIAN_POINT('Ctrl Pts',(-31.7350939690592,-68.593099193836,
82.9783528899875));
#207454=CARTESIAN_POINT('Ctrl Pts',(-31.7166927358616,-69.2504763472443,
83.3704778726981));
#207455=CARTESIAN_POINT('Ctrl Pts',(-31.6854023968601,-70.4027780984813,
83.9146022665282));
#207456=CARTESIAN_POINT('Ctrl Pts',(-31.6727694345795,-70.8781549672121,
84.1025441246547));
#207457=CARTESIAN_POINT('Ctrl Pts',(-31.6508516949256,-71.7274663599358,
84.3763095166132));
#207458=CARTESIAN_POINT('Ctrl Pts',(-31.6415772192522,-72.0962065035156,
84.4757752603689));
#207459=CARTESIAN_POINT('Ctrl Pts',(-31.6063238889962,-73.5105054038661,
84.7848089382225));
#207460=CARTESIAN_POINT('Ctrl Pts',(-31.5799383761504,-74.57788002886,84.8706817215814));
#207461=CARTESIAN_POINT('Ctrl Pts',(-31.5350170352657,-76.4108734893557,
84.7705654121244));
#207462=CARTESIAN_POINT('Ctrl Pts',(-31.5163791767883,-77.1735670391079,
84.6537270219544));
#207463=CARTESIAN_POINT('Ctrl Pts',(-31.4785596195015,-78.6606251574944,
84.2748805738338));
#207464=CARTESIAN_POINT('Ctrl Pts',(-31.4596683080806,-79.3817144600273,
84.0147041477492));
#207465=CARTESIAN_POINT('Ctrl Pts',(-31.4127643992252,-81.1193900753321,
83.1900685887214));
#207466=CARTESIAN_POINT('Ctrl Pts',(-31.3841098156622,-82.0875618085936,
82.5423602128335));
#207467=CARTESIAN_POINT('Ctrl Pts',(-31.3464639612025,-83.2281269792472,
81.5089614646173));
#207468=CARTESIAN_POINT('Ctrl Pts',(-31.3372185144437,-83.4976051329108,
81.2400550818893));
#207469=CARTESIAN_POINT('Ctrl Pts',(-31.3097513713876,-84.2546823859785,
80.4080249033765));
#207470=CARTESIAN_POINT('Ctrl Pts',(-31.2913800401256,-84.7026497717221,
79.8113813780443));
#207471=CARTESIAN_POINT('Ctrl Pts',(-31.2545593096663,-85.483193428776,
78.5376459511404));
#207472=CARTESIAN_POINT('Ctrl Pts',(-31.2364814300193,-85.8132163418888,
77.8629104229391));
#207473=CARTESIAN_POINT('Ctrl Pts',(-31.1990043821139,-86.3527121201128,
76.4297261704076));
#207474=CARTESIAN_POINT('Ctrl Pts',(-31.1796109525616,-86.5550121217493,
75.6724401148098));
#207475=CARTESIAN_POINT('Ctrl Pts',(-31.1512319426453,-86.7425971277642,
74.525085894939));
#207476=CARTESIAN_POINT('Ctrl Pts',(-31.1420081022768,-86.7858641947752,
74.1466688461417));
#207477=CARTESIAN_POINT('Ctrl Pts',(-31.1145807181722,-86.8597638973797,
73.0221985032259));
#207478=CARTESIAN_POINT('Ctrl Pts',(-31.0962362007859,-86.8381924195305,
72.274610871309));
#207479=CARTESIAN_POINT('Ctrl Pts',(-31.0595156209465,-86.6543553234396,
70.7914046819641));
#207480=CARTESIAN_POINT('Ctrl Pts',(-31.0415259441024,-86.4921070713351,
70.0591576044501));
#207481=CARTESIAN_POINT('Ctrl Pts',(-31.0156884375958,-86.1658214882129,
69.0502525285244));
#207482=CARTESIAN_POINT('Ctrl Pts',(-31.0080604245923,-86.0581626590963,
68.7574460529718));
#207483=CARTESIAN_POINT('Ctrl Pts',(-31.000413750398,-85.9391496391482,
68.4693880297961));
#207484=CARTESIAN_POINT('Origin',(-27.5423496375577,-74.9965420974961,72.9903965241317));
#207485=CARTESIAN_POINT('',(-28.8902889611216,-85.9391496391482,68.4693880297961));
#207486=CARTESIAN_POINT('',(-29.1863798856002,-85.9391496391482,68.4693880297961));
#207487=CARTESIAN_POINT('',(-27.5423496375574,-85.9391496391482,68.4693880297962));
#207488=CARTESIAN_POINT('Ctrl Pts',(-28.8902889611216,-85.9391496391482,
68.4693880297961));
#207489=CARTESIAN_POINT('Ctrl Pts',(-28.8995283211901,-86.0828659887593,
68.817237765775));
#207490=CARTESIAN_POINT('Ctrl Pts',(-28.9087847558972,-86.2099969740892,
69.1719428377128));
#207491=CARTESIAN_POINT('Ctrl Pts',(-28.9365166337169,-86.5427728456659,
70.2616199806556));
#207492=CARTESIAN_POINT('Ctrl Pts',(-28.9548136351524,-86.6945173551246,
71.0107379450507));
#207493=CARTESIAN_POINT('Ctrl Pts',(-28.9826977064045,-86.8122987634401,
72.1465922017969));
#207494=CARTESIAN_POINT('Ctrl Pts',(-28.9920030101979,-86.8332684586263,
72.5256173699335));
#207495=CARTESIAN_POINT('Ctrl Pts',(-29.0195714954137,-86.8413959006649,
73.652315710583));
#207496=CARTESIAN_POINT('Ctrl Pts',(-29.0374679912989,-86.7760169187804,
74.3984708422766));
#207497=CARTESIAN_POINT('Ctrl Pts',(-29.0745754429211,-86.4989551491749,
75.9038615842204));
#207498=CARTESIAN_POINT('Ctrl Pts',(-29.0938293857601,-86.2810628959108,
76.6582800598336));
#207499=CARTESIAN_POINT('Ctrl Pts',(-29.1312567660433,-85.7078102381637,
78.0921471338613));
#207500=CARTESIAN_POINT('Ctrl Pts',(-29.1494411374351,-85.3578996415665,
78.7697910615343));
#207501=CARTESIAN_POINT('Ctrl Pts',(-29.1834627613708,-84.5997096230225,
79.9449582163071));
#207502=CARTESIAN_POINT('Ctrl Pts',(-29.1990955263269,-84.2113052693821,
80.4519580931511));
#207503=CARTESIAN_POINT('Ctrl Pts',(-29.223663925763,-83.5292890863697,
81.2072584288094));
#207504=CARTESIAN_POINT('Ctrl Pts',(-29.2327815354917,-83.2611762405944,
81.4768807104254));
#207505=CARTESIAN_POINT('Ctrl Pts',(-29.2598230591689,-82.4330918413416,
82.2331011690959));
#207506=CARTESIAN_POINT('Ctrl Pts',(-29.2778991984299,-81.8398692406232,
82.6805318777052));
#207507=CARTESIAN_POINT('Ctrl Pts',(-29.3141450695314,-80.5721043557795,
83.4619063847497));
#207508=CARTESIAN_POINT('Ctrl Pts',(-29.3319583185975,-79.8997463284145,
83.7930814781586));
#207509=CARTESIAN_POINT('Ctrl Pts',(-29.3672593369409,-78.5355352643541,
84.311258612612));
#207510=CARTESIAN_POINT('Ctrl Pts',(-29.3846907415346,-77.8489968223934,
84.5034276010871));
#207511=CARTESIAN_POINT('Ctrl Pts',(-29.4197344489482,-76.4262357244761,
84.7665150256504));
#207512=CARTESIAN_POINT('Ctrl Pts',(-29.4372673189812,-75.6922061657539,
84.8325690467404));
#207513=CARTESIAN_POINT('Ctrl Pts',(-29.4732775397643,-74.2086489955821,
84.8275898494527));
#207514=CARTESIAN_POINT('Ctrl Pts',(-29.4916136494817,-73.4624104466234,
84.7541701221947));
#207515=CARTESIAN_POINT('Ctrl Pts',(-29.5187968234955,-72.3559276941455,
84.5381724100144));
#207516=CARTESIAN_POINT('Ctrl Pts',(-29.5279055210172,-71.9874554292504,
84.447681096201));
#207517=CARTESIAN_POINT('Ctrl Pts',(-29.5556043148239,-70.8887031839507,
84.1211728614577));
#207518=CARTESIAN_POINT('Ctrl Pts',(-29.5743943838771,-70.176419571956,
83.8317491779264));
#207519=CARTESIAN_POINT('Ctrl Pts',(-29.6166217713601,-68.6389933094776,
83.0253745443578));
#207520=CARTESIAN_POINT('Ctrl Pts',(-29.6397325088142,-67.8393284889846,
82.4716152789057));
#207521=CARTESIAN_POINT('Ctrl Pts',(-29.6727251199189,-66.83227203796,81.5734915450803));
#207522=CARTESIAN_POINT('Ctrl Pts',(-29.6820549697602,-66.5607898095081,
81.3068205885803));
#207523=CARTESIAN_POINT('Ctrl Pts',(-29.7135942094719,-65.6818272063981,
80.3560312107896));
#207524=CARTESIAN_POINT('Ctrl Pts',(-29.7354604200767,-65.1409273570892,
79.6148476331426));
#207525=CARTESIAN_POINT('Ctrl Pts',(-29.7671521443193,-64.5037619811568,
78.4882150363556));
#207526=CARTESIAN_POINT('Ctrl Pts',(-29.7764893851431,-64.3328021039724,
78.1487966704457));
#207527=CARTESIAN_POINT('Ctrl Pts',(-29.8140374973234,-63.7088234368817,
76.7458116307822));
#207528=CARTESIAN_POINT('Ctrl Pts',(-29.8417315397632,-63.3963174211873,
75.6267801525121));
#207529=CARTESIAN_POINT('Ctrl Pts',(-29.8890836023462,-63.1539811167698,
73.7163291010924));
#207530=CARTESIAN_POINT('Ctrl Pts',(-29.9076924443221,-63.131840415978,
72.9447162553307));
#207531=CARTESIAN_POINT('Ctrl Pts',(-29.9450550017397,-63.2372823510437,
71.4145964340451));
#207532=CARTESIAN_POINT('Ctrl Pts',(-29.9639085109905,-63.3633654104137,
70.6596194303905));
#207533=CARTESIAN_POINT('Ctrl Pts',(-30.0085207959319,-63.8343849018536,
68.9041877426353));
#207534=CARTESIAN_POINT('Ctrl Pts',(-30.0338703028542,-64.2421911750197,
67.9273150329408));
#207535=CARTESIAN_POINT('Ctrl Pts',(-30.0693099484831,-64.9667602581611,
66.6872345673202));
#207536=CARTESIAN_POINT('Ctrl Pts',(-30.0787578858061,-65.1755346487063,
66.3666370547101));
#207537=CARTESIAN_POINT('Ctrl Pts',(-30.1002166176163,-65.6890186467851,
65.6559118241576));
#207538=CARTESIAN_POINT('Ctrl Pts',(-30.1122017028276,-66.0034048638451,
65.2736521907534));
#207539=CARTESIAN_POINT('Ctrl Pts',(-30.1428913209674,-66.8597673107173,
64.3560645921094));
#207540=CARTESIAN_POINT('Ctrl Pts',(-30.1617406158681,-67.4311487764751,
63.8512717027624));
#207541=CARTESIAN_POINT('Ctrl Pts',(-30.1997217089976,-68.6816661592658,
62.94464768289));
#207542=CARTESIAN_POINT('Ctrl Pts',(-30.2186374492105,-69.3604796340118,
62.5486757851087));
#207543=CARTESIAN_POINT('Ctrl Pts',(-30.2562923496927,-70.7525956015514,
61.9121843293235));
#207544=CARTESIAN_POINT('Ctrl Pts',(-30.2748246328103,-71.4596214643,61.6666132054406));
#207545=CARTESIAN_POINT('Ctrl Pts',(-30.3023184544787,-72.5535867528755,
61.3991895158625));
#207546=CARTESIAN_POINT('Ctrl Pts',(-30.3115464992686,-72.9262373699216,
61.3268657950991));
#207547=CARTESIAN_POINT('Ctrl Pts',(-30.339443138637,-74.0548196951778,
61.163631644942));
#207548=CARTESIAN_POINT('Ctrl Pts',(-30.3583002721842,-74.8166679009763,
61.1275620744038));
#207549=CARTESIAN_POINT('Ctrl Pts',(-30.3962660247664,-76.3592346568466,
61.2032381620261));
#207550=CARTESIAN_POINT('Ctrl Pts',(-30.4151558405309,-77.1360426787338,
61.3192108467647));
#207551=CARTESIAN_POINT('Ctrl Pts',(-30.4527658357012,-78.6202333891019,
61.6940477278681));
#207552=CARTESIAN_POINT('Ctrl Pts',(-30.4712817497197,-79.3258368571948,
61.9452233127894));
#207553=CARTESIAN_POINT('Ctrl Pts',(-30.4987258026978,-80.346572414155,
62.4215242683615));
#207554=CARTESIAN_POINT('Ctrl Pts',(-30.5079261447506,-80.682203796793,
62.5982294610262));
#207555=CARTESIAN_POINT('Ctrl Pts',(-30.5357819144917,-81.6654910615277,
63.1778322987453));
#207556=CARTESIAN_POINT('Ctrl Pts',(-30.5546220355387,-82.2832805489083,
63.6274521458031));
#207557=CARTESIAN_POINT('Ctrl Pts',(-30.592489021526,-83.4391975601457,
64.6528521833681));
#207558=CARTESIAN_POINT('Ctrl Pts',(-30.6112994776759,-83.9718815960666,
65.229187676426));
#207559=CARTESIAN_POINT('Ctrl Pts',(-30.6487654182889,-84.8944066472866,
66.4504123203477));
#207560=CARTESIAN_POINT('Ctrl Pts',(-30.6672176269276,-85.2875297772593,
67.0883037849678));
#207561=CARTESIAN_POINT('Ctrl Pts',(-30.6916666439696,-85.7327469846333,
67.9922290522817));
#207562=CARTESIAN_POINT('Ctrl Pts',(-30.697956103958,-85.8398965092981,
68.2291566628825));
#207563=CARTESIAN_POINT('Ctrl Pts',(-30.7042591049895,-85.9391496438364,
68.4693880411434));
#207564=CARTESIAN_POINT('Ctrl Pts',(-31.000413750398,-85.9391496391482,
68.4693880297961));
#207565=CARTESIAN_POINT('Ctrl Pts',(-30.9894496914595,-85.7685047637428,
68.0563607366832));
#207566=CARTESIAN_POINT('Ctrl Pts',(-30.9784421937568,-85.5745171272631,
67.6530957880328));
#207567=CARTESIAN_POINT('Ctrl Pts',(-30.9489866478898,-84.9890409660733,
66.594169209003));
#207568=CARTESIAN_POINT('Ctrl Pts',(-30.9306856427922,-84.5564200349675,
65.9639821729572));
#207569=CARTESIAN_POINT('Ctrl Pts',(-30.9027964530365,-83.8223434458471,
65.0891727552971));
#207570=CARTESIAN_POINT('Ctrl Pts',(-30.8934900606079,-83.5646509049784,
64.8104443704195));
#207571=CARTESIAN_POINT('Ctrl Pts',(-30.8659179058485,-82.7609049498348,
64.0208156210601));
#207572=CARTESIAN_POINT('Ctrl Pts',(-30.8480189088652,-82.1793932751416,
63.5487143241095));
#207573=CARTESIAN_POINT('Ctrl Pts',(-30.8109072016306,-80.9052198210213,
62.7005335637446));
#207574=CARTESIAN_POINT('Ctrl Pts',(-30.7916515937246,-80.2117021199372,
62.332261004331));
#207575=CARTESIAN_POINT('Ctrl Pts',(-30.7542197255713,-78.7828348739039,
61.7465901526257));
#207576=CARTESIAN_POINT('Ctrl Pts',(-30.7360324761767,-78.0525681585849,
61.5265443642416));
#207577=CARTESIAN_POINT('Ctrl Pts',(-30.7082843972894,-76.933941270481,
61.3040471830111));
#207578=CARTESIAN_POINT('Ctrl Pts',(-30.6990064480223,-76.5582851223548,
61.2479421620343));
#207579=CARTESIAN_POINT('Ctrl Pts',(-30.6715352727106,-75.4373726781259,
61.1352798449406));
#207580=CARTESIAN_POINT('Ctrl Pts',(-30.6537045516274,-74.6887582132883,
61.1310797784556));
#207581=CARTESIAN_POINT('Ctrl Pts',(-30.616698716733,-73.1639679461412,
61.2670725895126));
#207582=CARTESIAN_POINT('Ctrl Pts',(-30.5974786207648,-72.3920292877713,
61.4140776340297));
#207583=CARTESIAN_POINT('Ctrl Pts',(-30.560137270925,-70.9114610705807,
61.8517288591366));
#207584=CARTESIAN_POINT('Ctrl Pts',(-30.5420056666565,-70.2050537507344,
62.1368510124088));
#207585=CARTESIAN_POINT('Ctrl Pts',(-30.5143121197003,-69.1938492896317,
62.66308946839));
#207586=CARTESIAN_POINT('Ctrl Pts',(-30.5050377464032,-68.865473614258,
62.8545929909763));
#207587=CARTESIAN_POINT('Ctrl Pts',(-30.4775977068192,-67.9209001963202,
63.4681772825442));
#207588=CARTESIAN_POINT('Ctrl Pts',(-30.4597881945804,-67.3347815885907,
63.9330903691818));
#207589=CARTESIAN_POINT('Ctrl Pts',(-30.422795492168,-66.2307352813139,
64.9931677445109));
#207590=CARTESIAN_POINT('Ctrl Pts',(-30.4035642681644,-65.7204745552141,
65.5910991910053));
#207591=CARTESIAN_POINT('Ctrl Pts',(-30.3661762005337,-64.839223198782,
66.8595510439525));
#207592=CARTESIAN_POINT('Ctrl Pts',(-30.3480147272345,-64.4665326441387,
67.5243833155983));
#207593=CARTESIAN_POINT('Ctrl Pts',(-30.3173044032287,-63.9580353402467,
68.6795630671376));
#207594=CARTESIAN_POINT('Ctrl Pts',(-30.3050081691236,-63.7852893419021,
69.1511613747627));
#207595=CARTESIAN_POINT('Ctrl Pts',(-30.2835062850145,-63.5345902378565,
69.9987605562438));
#207596=CARTESIAN_POINT('Ctrl Pts',(-30.2743102969878,-63.4440046693556,
70.3702618705647));
#207597=CARTESIAN_POINT('Ctrl Pts',(-30.2467410043588,-63.2273042486643,
71.4924223775198));
#207598=CARTESIAN_POINT('Ctrl Pts',(-30.2282552016501,-63.1553881146373,
72.251514331098));
#207599=CARTESIAN_POINT('Ctrl Pts',(-30.1913586400014,-63.1581686717972,
73.7590405717097));
#207600=CARTESIAN_POINT('Ctrl Pts',(-30.1733966847103,-63.2302014472502,
74.5040444931853));
#207601=CARTESIAN_POINT('Ctrl Pts',(-30.1353420038036,-63.5281125145034,
76.0453335219479));
#207602=CARTESIAN_POINT('Ctrl Pts',(-30.1150845932192,-63.7681252329433,
76.8348930486754));
#207603=CARTESIAN_POINT('Ctrl Pts',(-30.0857305276213,-64.236120142187,
77.9440350629426));
#207604=CARTESIAN_POINT('Ctrl Pts',(-30.0765347506166,-64.4010163055766,
78.2875702886592));
#207605=CARTESIAN_POINT('Ctrl Pts',(-30.0428586837917,-65.061971816687,
79.5097345229102));
#207606=CARTESIAN_POINT('Ctrl Pts',(-30.0179927316207,-65.6531656500806,
80.3319735496283));
#207607=CARTESIAN_POINT('Ctrl Pts',(-29.9841355838376,-66.6007529654551,
81.3471537236086));
#207608=CARTESIAN_POINT('Ctrl Pts',(-29.9749379466294,-66.8733574698408,
81.6123764882092));
#207609=CARTESIAN_POINT('Ctrl Pts',(-29.9427149566515,-67.8667577154263,
82.4898713783317));
#207610=CARTESIAN_POINT('Ctrl Pts',(-29.919341186383,-68.6476753332647,
83.0286095885551));
#207611=CARTESIAN_POINT('Ctrl Pts',(-29.8774996552032,-70.1627104857593,
83.8256098816011));
#207612=CARTESIAN_POINT('Ctrl Pts',(-29.8589967844682,-70.8741735942729,
84.11576661727));
#207613=CARTESIAN_POINT('Ctrl Pts',(-29.8308165594556,-71.9723342870696,
84.4437098691336));
#207614=CARTESIAN_POINT('Ctrl Pts',(-29.8214390084931,-72.341004740389,
84.5347605157055));
#207615=CARTESIAN_POINT('Ctrl Pts',(-29.793644439547,-73.44727190563,84.7521691218095));
#207616=CARTESIAN_POINT('Ctrl Pts',(-29.7755815110613,-74.1931497677014,
84.8265316423652));
#207617=CARTESIAN_POINT('Ctrl Pts',(-29.7391907940018,-75.6794620293426,
84.8334988644618));
#207618=CARTESIAN_POINT('Ctrl Pts',(-29.7208679422351,-76.4165826127964,
84.7678719069554));
#207619=CARTESIAN_POINT('Ctrl Pts',(-29.6850838483618,-77.8499336465015,
84.5036674362128));
#207620=CARTESIAN_POINT('Ctrl Pts',(-29.6677084140173,-78.5437558307006,
84.3091655361343));
#207621=CARTESIAN_POINT('Ctrl Pts',(-29.6316592996847,-79.9141711786744,
83.7865084938981));
#207622=CARTESIAN_POINT('Ctrl Pts',(-29.6130886579637,-80.5859096273871,
83.4545299006682));
#207623=CARTESIAN_POINT('Ctrl Pts',(-29.5766865576896,-81.8532708661213,
82.6711241673343));
#207624=CARTESIAN_POINT('Ctrl Pts',(-29.5586589112364,-82.446591262627,
82.2222968715369));
#207625=CARTESIAN_POINT('Ctrl Pts',(-29.5309788247761,-83.2742408827129,
81.4641411954743));
#207626=CARTESIAN_POINT('Ctrl Pts',(-29.5215695524635,-83.5419880701921,
81.1940541730913));
#207627=CARTESIAN_POINT('Ctrl Pts',(-29.497077497559,-84.2072318305858,
80.4550248991315));
#207628=CARTESIAN_POINT('Ctrl Pts',(-29.4822163965591,-84.5820327648268,
79.9672046446882));
#207629=CARTESIAN_POINT('Ctrl Pts',(-29.4485768052743,-85.3333166045812,
78.8138212269672));
#207630=CARTESIAN_POINT('Ctrl Pts',(-29.4297129690653,-85.6866920038498,
78.136449853645));
#207631=CARTESIAN_POINT('Ctrl Pts',(-29.3917545451188,-86.2661187543358,
76.7038891394555));
#207632=CARTESIAN_POINT('Ctrl Pts',(-29.3729028524161,-86.4869973251195,
75.9506039495689));
#207633=CARTESIAN_POINT('Ctrl Pts',(-29.3353572175053,-86.7702323688165,
74.4462388093395));
#207634=CARTESIAN_POINT('Ctrl Pts',(-29.3168550496728,-86.8386605925247,
73.699972782897));
#207635=CARTESIAN_POINT('Ctrl Pts',(-29.280503388481,-86.833846342415,72.2056509893591));
#207636=CARTESIAN_POINT('Ctrl Pts',(-29.2624303820932,-86.7608265292928,
71.4609495908793));
#207637=CARTESIAN_POINT('Ctrl Pts',(-29.2347456172494,-86.5454194912509,
70.3543832744611));
#207638=CARTESIAN_POINT('Ctrl Pts',(-29.2253655360832,-86.4546865015407,
69.9843922351259));
#207639=CARTESIAN_POINT('Ctrl Pts',(-29.2060769114763,-86.2303559646516,
69.229094147064));
#207640=CARTESIAN_POINT('Ctrl Pts',(-29.1962359460246,-86.0944395319839,
68.845250263768));
#207641=CARTESIAN_POINT('Ctrl Pts',(-29.1863798856002,-85.9391496391482,
68.4693880297961));
#207642=CARTESIAN_POINT('Origin',(-27.5423496375577,-74.9965420974961,72.9903965241317));
#207643=CARTESIAN_POINT('',(-27.0763524854127,-85.9391496391482,68.4693880297962));
#207644=CARTESIAN_POINT('',(-27.3723203523406,-85.9391496418573,68.4693880363532));
#207645=CARTESIAN_POINT('',(-27.5423496375574,-85.9391496391482,68.4693880297962));
#207646=CARTESIAN_POINT('Ctrl Pts',(-27.0763524854127,-85.9391496391482,
68.4693880297962));
#207647=CARTESIAN_POINT('Ctrl Pts',(-27.0854958243982,-86.0832420586906,
68.8181480019916));
#207648=CARTESIAN_POINT('Ctrl Pts',(-27.0946269738679,-86.2106594560495,
69.1737926277716));
#207649=CARTESIAN_POINT('Ctrl Pts',(-27.1228582600314,-86.5493155510614,
70.283709893587));
#207650=CARTESIAN_POINT('Ctrl Pts',(-27.1421585225472,-86.7029336633776,
71.053098990638));
#207651=CARTESIAN_POINT('Ctrl Pts',(-27.17041855609,-86.8167726463045,72.2110433942339));
#207652=CARTESIAN_POINT('Ctrl Pts',(-27.1795935858813,-86.8357252283469,
72.5916666797719));
#207653=CARTESIAN_POINT('Ctrl Pts',(-27.2077451655468,-86.8374804134635,
73.7554635391027));
#207654=CARTESIAN_POINT('Ctrl Pts',(-27.2268821242396,-86.7609998238509,
74.5365753507185));
#207655=CARTESIAN_POINT('Ctrl Pts',(-27.2642716278407,-86.4617074378826,
76.0384000127796));
#207656=CARTESIAN_POINT('Ctrl Pts',(-27.2821489972801,-86.2461607100747,
76.7568834329032));
#207657=CARTESIAN_POINT('Ctrl Pts',(-27.3152541188379,-85.7317463330596,
78.0219489283277));
#207658=CARTESIAN_POINT('Ctrl Pts',(-27.3303623796387,-85.4549018410693,
78.5746454022493));
#207659=CARTESIAN_POINT('Ctrl Pts',(-27.3636484640859,-84.7492010731034,
79.7452307442853));
#207660=CARTESIAN_POINT('Ctrl Pts',(-27.3815147552166,-84.3020647535182,
80.3490235437407));
#207661=CARTESIAN_POINT('Ctrl Pts',(-27.414094271405,-83.4029500332305,
81.3490243729791));
#207662=CARTESIAN_POINT('Ctrl Pts',(-27.42864906318,-82.9722483421988,81.7609414970286));
#207663=CARTESIAN_POINT('Ctrl Pts',(-27.4524654145557,-82.215525696821,
82.3826318433475));
#207664=CARTESIAN_POINT('Ctrl Pts',(-27.4617059544625,-81.9069456727931,
82.6119416897413));
#207665=CARTESIAN_POINT('Ctrl Pts',(-27.4975499411919,-80.6692153515452,
83.4414062209669));
#207666=CARTESIAN_POINT('Ctrl Pts',(-27.5245562214543,-79.6689475592958,
83.9252692475761));
#207667=CARTESIAN_POINT('Ctrl Pts',(-27.5604332604563,-78.2542686781622,
84.3795080463537));
#207668=CARTESIAN_POINT('Ctrl Pts',(-27.569546337496,-77.8869933492492,
84.4782133806877));
#207669=CARTESIAN_POINT('Ctrl Pts',(-27.5996011291581,-76.6680617310802,
84.743634102178));
#207670=CARTESIAN_POINT('Ctrl Pts',(-27.6208060446094,-75.8028037754163,
84.8344875628036));
#207671=CARTESIAN_POINT('Ctrl Pts',(-27.6601660945229,-74.1802254319195,
84.8261111357782));
#207672=CARTESIAN_POINT('Ctrl Pts',(-27.678163838067,-73.4271326307702,
84.7499659232919));
#207673=CARTESIAN_POINT('Ctrl Pts',(-27.7096512555339,-72.155460078534,
84.4969827358799));
#207674=CARTESIAN_POINT('Ctrl Pts',(-27.722910279037,-71.6323539700395,
84.3550570407994));
#207675=CARTESIAN_POINT('Ctrl Pts',(-27.7453913084619,-70.7591413854709,
84.0525441104013));
#207676=CARTESIAN_POINT('Ctrl Pts',(-27.7546006665861,-70.4037705024483,
83.9097886059322));
#207677=CARTESIAN_POINT('Ctrl Pts',(-27.782192090083,-69.3635283837108,
83.4321325338603));
#207678=CARTESIAN_POINT('Ctrl Pts',(-27.8006798026253,-68.7034257213282,
83.0480985277529));
#207679=CARTESIAN_POINT('Ctrl Pts',(-27.8375958582695,-67.4779572579048,
82.1669823762717));
#207680=CARTESIAN_POINT('Ctrl Pts',(-27.8555730354232,-66.9137755313285,
81.6741592142469));
#207681=CARTESIAN_POINT('Ctrl Pts',(-27.8943775210409,-65.8118876914272,
80.5105983339386));
#207682=CARTESIAN_POINT('Ctrl Pts',(-27.9154171071773,-65.2929316034503,
79.8278842459823));
#207683=CARTESIAN_POINT('Ctrl Pts',(-27.9547657332123,-64.4593718710948,
78.4427521309384));
#207684=CARTESIAN_POINT('Ctrl Pts',(-27.9730378279666,-64.1305677171517,
77.7538769334039));
#207685=CARTESIAN_POINT('Ctrl Pts',(-28.0009792322269,-63.7399154047799,
76.6800802198003));
#207686=CARTESIAN_POINT('Ctrl Pts',(-28.0103472509272,-63.6269930873546,
76.3158686007264));
#207687=CARTESIAN_POINT('Ctrl Pts',(-28.0380276306472,-63.3454586317787,
75.2241170171683));
#207688=CARTESIAN_POINT('Ctrl Pts',(-28.0559933115398,-63.2278430736962,
74.4853807791906));
#207689=CARTESIAN_POINT('Ctrl Pts',(-28.0906017774928,-63.1378619891058,
73.0679641596003));
#207690=CARTESIAN_POINT('Ctrl Pts',(-28.1072138532676,-63.1526649094277,
72.3930065568334));
#207691=CARTESIAN_POINT('Ctrl Pts',(-28.1430018502095,-63.3086502028039,
70.9442050877484));
#207692=CARTESIAN_POINT('Ctrl Pts',(-28.1618386467817,-63.4695746651608,
70.1756605434761));
#207693=CARTESIAN_POINT('Ctrl Pts',(-28.1951719525807,-63.8788966067122,
68.8780392101065));
#207694=CARTESIAN_POINT('Ctrl Pts',(-28.209451321217,-64.0926259071167,
68.3408662960563));
#207695=CARTESIAN_POINT('Ctrl Pts',(-28.2330434613466,-64.5115675363652,
67.477538743212));
#207696=CARTESIAN_POINT('Ctrl Pts',(-28.2423403980979,-64.6950042239373,
67.1419257611867));
#207697=CARTESIAN_POINT('Ctrl Pts',(-28.2782575692713,-65.4642324921899,
65.8834052913237));
#207698=CARTESIAN_POINT('Ctrl Pts',(-28.3052940638149,-66.1604550120399,
65.0344049615902));
#207699=CARTESIAN_POINT('Ctrl Pts',(-28.350874467331,-67.5289153598374,
63.7704257229028));
#207700=CARTESIAN_POINT('Ctrl Pts',(-28.3695263041074,-68.1443016492391,
63.3043181251833));
#207701=CARTESIAN_POINT('Ctrl Pts',(-28.4073533634817,-69.452036387946,
62.5012072138239));
#207702=CARTESIAN_POINT('Ctrl Pts',(-28.4262322373492,-70.1407193831999,
62.1651652551974));
#207703=CARTESIAN_POINT('Ctrl Pts',(-28.4729977225934,-71.9374544942296,
61.4946502189513));
#207704=CARTESIAN_POINT('Ctrl Pts',(-28.5015233185326,-73.0710745963116,
61.2514541564332));
#207705=CARTESIAN_POINT('Ctrl Pts',(-28.539037728165,-74.6015318743609,
61.1511013483145));
#207706=CARTESIAN_POINT('Ctrl Pts',(-28.5482828840261,-74.9821772154139,
61.1445222323692));
#207707=CARTESIAN_POINT('Ctrl Pts',(-28.5757505360324,-76.1066502335183,
61.1792932576915));
#207708=CARTESIAN_POINT('Ctrl Pts',(-28.5941223390068,-76.8469945147195,
61.2724481329931));
#207709=CARTESIAN_POINT('Ctrl Pts',(-28.6309417874922,-78.3050861885961,
61.597622529213));
#207710=CARTESIAN_POINT('Ctrl Pts',(-28.649017256776,-79.0193697578069,
61.829813117216));
#207711=CARTESIAN_POINT('Ctrl Pts',(-28.6864894041204,-80.424296898995,
62.439041713671));
#207712=CARTESIAN_POINT('Ctrl Pts',(-28.705881136776,-81.1091114536378,
62.8204354895673));
#207713=CARTESIAN_POINT('Ctrl Pts',(-28.7342580491699,-82.0639475914451,
63.4837217852691));
#207714=CARTESIAN_POINT('Ctrl Pts',(-28.7434809356145,-82.3659292479492,
63.7158496889855));
#207715=CARTESIAN_POINT('Ctrl Pts',(-28.7709065316449,-83.2252871348818,
64.4449357595009));
#207716=CARTESIAN_POINT('Ctrl Pts',(-28.7892499602592,-83.7474465205768,
64.9804773629521));
#207717=CARTESIAN_POINT('Ctrl Pts',(-28.8259669934294,-84.6852208613554,
66.1442567743271));
#207718=CARTESIAN_POINT('Ctrl Pts',(-28.8439536997745,-85.0984403092417,
66.7701248636407));
#207719=CARTESIAN_POINT('Ctrl Pts',(-28.8715192371081,-85.6297322719695,
67.76907056115));
#207720=CARTESIAN_POINT('Ctrl Pts',(-28.8808941381578,-85.7930150961074,
68.1156853205936));
#207721=CARTESIAN_POINT('Ctrl Pts',(-28.8902889611216,-85.9391496391482,
68.4693880297961));
#207722=CARTESIAN_POINT('Ctrl Pts',(-29.1863798856002,-85.9391496391482,
68.4693880297961));
#207723=CARTESIAN_POINT('Ctrl Pts',(-29.1772971019885,-85.7960433235432,
68.1230148145369));
#207724=CARTESIAN_POINT('Ctrl Pts',(-29.1681963644014,-85.6364843713224,
67.783420036426));
#207725=CARTESIAN_POINT('Ctrl Pts',(-29.1407582807521,-85.1107337065779,
66.7900910423739));
#207726=CARTESIAN_POINT('Ctrl Pts',(-29.1223061210748,-84.6985425981529,
66.1631089736439));
#207727=CARTESIAN_POINT('Ctrl Pts',(-29.086126866369,-83.7636903125962,
64.9983969503919));
#207728=CARTESIAN_POINT('Ctrl Pts',(-29.0681898763684,-83.2436912315594,
64.4628250181062));
#207729=CARTESIAN_POINT('Ctrl Pts',(-29.0406822288947,-82.3871745438409,
63.7327731941406));
#207730=CARTESIAN_POINT('Ctrl Pts',(-29.0313471682672,-82.085776424672,
63.4999911451696));
#207731=CARTESIAN_POINT('Ctrl Pts',(-28.9963513666028,-80.9090654919775,
62.6785523534647));
#207732=CARTESIAN_POINT('Ctrl Pts',(-28.9712333862021,-79.9676695700785,
62.1931766210143));
#207733=CARTESIAN_POINT('Ctrl Pts',(-28.936153491432,-78.6150149385664,
61.7106575674738));
#207734=CARTESIAN_POINT('Ctrl Pts',(-28.9268151025791,-78.2495315632111,
61.5998777430556));
#207735=CARTESIAN_POINT('Ctrl Pts',(-28.8986232865437,-77.1209857350694,
61.3165687150427));
#207736=CARTESIAN_POINT('Ctrl Pts',(-28.8799524364902,-76.3456378895604,
61.2017806270506));
#207737=CARTESIAN_POINT('Ctrl Pts',(-28.84277626314,-74.8190565486453,61.1284459314675));
#207738=CARTESIAN_POINT('Ctrl Pts',(-28.8245393308923,-74.0717378243645,
61.1632193222358));
#207739=CARTESIAN_POINT('Ctrl Pts',(-28.7973642074776,-72.9538852843799,
61.3218872134568));
#207740=CARTESIAN_POINT('Ctrl Pts',(-28.7881723804377,-72.5779165325592,
61.3939830133214));
#207741=CARTESIAN_POINT('Ctrl Pts',(-28.7605398889809,-71.467218577826,
61.6633444746261));
#207742=CARTESIAN_POINT('Ctrl Pts',(-28.7419026733009,-70.7473162378985,
61.9132892231419));
#207743=CARTESIAN_POINT('Ctrl Pts',(-28.7024162991224,-69.2638670363202,
62.5943845610187));
#207744=CARTESIAN_POINT('Ctrl Pts',(-28.6816183984185,-68.5139859753697,
63.0446887362641));
#207745=CARTESIAN_POINT('Ctrl Pts',(-28.6511205513814,-67.5178540827379,
63.8037720930618));
#207746=CARTESIAN_POINT('Ctrl Pts',(-28.6418249490305,-67.2266154303546,
64.0487477735725));
#207747=CARTESIAN_POINT('Ctrl Pts',(-28.6070570797181,-66.1770088413486,
65.0216909239259));
#207748=CARTESIAN_POINT('Ctrl Pts',(-28.5820663180276,-65.5048692407564,
65.8354971531125));
#207749=CARTESIAN_POINT('Ctrl Pts',(-28.5471143481036,-64.7472228277439,
67.0509431605125));
#207750=CARTESIAN_POINT('Ctrl Pts',(-28.5377911110625,-64.5612176840882,
67.3841804834701));
#207751=CARTESIAN_POINT('Ctrl Pts',(-28.5057992212909,-63.9736707187411,
68.5677290036345));
#207752=CARTESIAN_POINT('Ctrl Pts',(-28.4833135156324,-63.6574612378688,
69.4564278876824));
#207753=CARTESIAN_POINT('Ctrl Pts',(-28.4510316098729,-63.3654362439088,
70.7447832160995));
#207754=CARTESIAN_POINT('Ctrl Pts',(-28.4416982050555,-63.299187330961,
71.1202907801755));
#207755=CARTESIAN_POINT('Ctrl Pts',(-28.4111483995126,-63.1405535562565,
72.3690450414608));
#207756=CARTESIAN_POINT('Ctrl Pts',(-28.3901404343418,-63.1271069850738,
73.2493573598642));
#207757=CARTESIAN_POINT('Ctrl Pts',(-28.3593818012442,-63.247423227447,
74.5012803414066));
#207758=CARTESIAN_POINT('Ctrl Pts',(-28.3500533854523,-63.3019615544363,
74.8775504441455));
#207759=CARTESIAN_POINT('Ctrl Pts',(-28.3145658838677,-63.5795131831366,
76.3047652862547));
#207760=CARTESIAN_POINT('Ctrl Pts',(-28.2888790660904,-63.9270181929924,
77.3262045619693));
#207761=CARTESIAN_POINT('Ctrl Pts',(-28.253128170771,-64.5784613645797,
78.6286525642252));
#207762=CARTESIAN_POINT('Ctrl Pts',(-28.2437350477626,-64.7659425711944,
78.9620942217622));
#207763=CARTESIAN_POINT('Ctrl Pts',(-28.2210603974966,-65.261384644195,
79.751223920991));
#207764=CARTESIAN_POINT('Ctrl Pts',(-28.2078117545108,-65.5855813581234,
80.1956652425472));
#207765=CARTESIAN_POINT('Ctrl Pts',(-28.1753370399049,-66.4432887600706,
81.2143830534427));
#207766=CARTESIAN_POINT('Ctrl Pts',(-28.1559792817018,-67.0051748741336,
81.7613796200071));
#207767=CARTESIAN_POINT('Ctrl Pts',(-28.1238826824113,-68.0341112928614,
82.581507257976));
#207768=CARTESIAN_POINT('Ctrl Pts',(-28.1109884955671,-68.4733393884123,
82.8854799455036));
#207769=CARTESIAN_POINT('Ctrl Pts',(-28.0794727435621,-69.5815716782739,
83.5464889931359));
#207770=CARTESIAN_POINT('Ctrl Pts',(-28.0607239664772,-70.2672509867591,
83.8709658275296));
#207771=CARTESIAN_POINT('Ctrl Pts',(-28.0217455610983,-71.7645473977778,
84.4110543225423));
#207772=CARTESIAN_POINT('Ctrl Pts',(-28.0016036491204,-72.5776705248003,
84.6104775775714));
#207773=CARTESIAN_POINT('Ctrl Pts',(-27.9626090655067,-74.1466431912166,
84.8233178847389));
#207774=CARTESIAN_POINT('Ctrl Pts',(-27.944140686824,-74.8961773583242,
84.8533764503368));
#207775=CARTESIAN_POINT('Ctrl Pts',(-27.9073466166383,-76.4035714098902,
84.7708829331443));
#207776=CARTESIAN_POINT('Ctrl Pts',(-27.8887394009146,-77.1578438435078,
84.6560880138918));
#207777=CARTESIAN_POINT('Ctrl Pts',(-27.8604553618274,-78.2675743292867,
84.3758045125257));
#207778=CARTESIAN_POINT('Ctrl Pts',(-27.8509778381277,-78.6345156666761,
84.2639194082339));
#207779=CARTESIAN_POINT('Ctrl Pts',(-27.8282952642196,-79.5066990884764,
83.9509517373548));
#207780=CARTESIAN_POINT('Ctrl Pts',(-27.8151196182559,-80.0047829154031,
83.7325011740936));
#207781=CARTESIAN_POINT('Ctrl Pts',(-27.7833096066947,-81.1546297060221,
83.1307836630291));
#207782=CARTESIAN_POINT('Ctrl Pts',(-27.7645629968101,-81.7881823980881,
82.7178376662782));
#207783=CARTESIAN_POINT('Ctrl Pts',(-27.724612867408,-83.0623235968154,
81.7018345949151));
#207784=CARTESIAN_POINT('Ctrl Pts',(-27.7034548636324,-83.6839390151742,
81.082066834104));
#207785=CARTESIAN_POINT('Ctrl Pts',(-27.672478627145,-84.4697558964199,
80.1025887706415));
#207786=CARTESIAN_POINT('Ctrl Pts',(-27.6630586456205,-84.6934918862971,
79.7943823483294));
#207787=CARTESIAN_POINT('Ctrl Pts',(-27.6344430041026,-85.3309789543933,
78.8207398754691));
#207788=CARTESIAN_POINT('Ctrl Pts',(-27.6155741924473,-85.6939013615658,
78.1245952783084));
#207789=CARTESIAN_POINT('Ctrl Pts',(-27.5779950692029,-86.2637759448029,
76.7037178938473));
#207790=CARTESIAN_POINT('Ctrl Pts',(-27.559469337933,-86.4757554127163,
75.9848889626256));
#207791=CARTESIAN_POINT('Ctrl Pts',(-27.5230989687509,-86.7608444447559,
74.5191435707775));
#207792=CARTESIAN_POINT('Ctrl Pts',(-27.5050372303059,-86.8337435163221,
73.775596407627));
#207793=CARTESIAN_POINT('Ctrl Pts',(-27.4773527021625,-86.83752431961,72.6495276199141));
#207794=CARTESIAN_POINT('Ctrl Pts',(-27.4679637405674,-86.8204473139073,
72.2690664875133));
#207795=CARTESIAN_POINT('Ctrl Pts',(-27.4394453805095,-86.7123543098441,
71.1109723305979));
#207796=CARTESIAN_POINT('Ctrl Pts',(-27.420664768781,-86.5625736543532,
70.3409800383466));
#207797=CARTESIAN_POINT('Ctrl Pts',(-27.3918260336057,-86.2238438127127,
69.2107403412772));
#207798=CARTESIAN_POINT('Ctrl Pts',(-27.3820680337574,-86.0907277246481,
68.836266240543));
#207799=CARTESIAN_POINT('Ctrl Pts',(-27.3723203523406,-85.9391496445663,
68.4693880429103));
#207800=CARTESIAN_POINT('Origin',(-33.5526503323277,-74.999949493375,72.9851176492631));
#207801=CARTESIAN_POINT('',(-37.9576288901553,-85.9425570350205,68.4641091549305));
#207802=CARTESIAN_POINT('',(-38.2588681851947,-85.9425518661828,68.4640966443435));
#207803=CARTESIAN_POINT('',(-33.5526503323277,-85.9425570350204,68.4641091549303));
#207804=CARTESIAN_POINT('',(-37.9576293742551,-85.9425645971074,68.4641274581797));
#207805=CARTESIAN_POINT('Ctrl Pts',(-37.9576288901553,-85.9425570350206,
68.4641091549307));
#207806=CARTESIAN_POINT('Ctrl Pts',(-37.9576291329799,-85.9425608281721,
68.4641183358399));
#207807=CARTESIAN_POINT('Ctrl Pts',(-37.9576293758044,-85.9425646213122,
68.4641275167542));
#207808=CARTESIAN_POINT('Ctrl Pts',(-37.9576296186288,-85.9425684144409,
68.4641366976736));
#207809=CARTESIAN_POINT('',(-38.4180624217171,-79.3025708087853,84.0154429842386));
#207810=CARTESIAN_POINT('Ctrl Pts',(-37.9576293742551,-85.9425645971074,
68.4641274581797));
#207811=CARTESIAN_POINT('Ctrl Pts',(-37.9743923969875,-86.2044180485594,
69.0979181570568));
#207812=CARTESIAN_POINT('Ctrl Pts',(-37.9910143369726,-86.4107141752036,
69.7532621342486));
#207813=CARTESIAN_POINT('Ctrl Pts',(-38.0246878627216,-86.706819364395,
71.0890404319913));
#207814=CARTESIAN_POINT('Ctrl Pts',(-38.0416261577221,-86.7966319325827,
71.7668394250167));
#207815=CARTESIAN_POINT('Ctrl Pts',(-38.0694126443366,-86.8481623115025,
72.9028136493742));
#207816=CARTESIAN_POINT('Ctrl Pts',(-38.0804609652665,-86.8425840969132,
73.3578466519687));
#207817=CARTESIAN_POINT('Ctrl Pts',(-38.1107350188431,-86.7563114151496,
74.5909878161061));
#207818=CARTESIAN_POINT('Ctrl Pts',(-38.1301458593981,-86.624726229738,
75.3632308311965));
#207819=CARTESIAN_POINT('Ctrl Pts',(-38.1586472131736,-86.3172838441829,
76.4841413512661));
#207820=CARTESIAN_POINT('Ctrl Pts',(-38.1679026264474,-86.1988822198968,
76.8463520170879));
#207821=CARTESIAN_POINT('Ctrl Pts',(-38.1865718755565,-85.9263093144659,
77.5614275235112));
#207822=CARTESIAN_POINT('Ctrl Pts',(-38.1959758908047,-85.7719763124514,
77.9137470500015));
#207823=CARTESIAN_POINT('Ctrl Pts',(-38.2228550042187,-85.2855496534766,
78.8916927030285));
#207824=CARTESIAN_POINT('Ctrl Pts',(-38.2403936750185,-84.9141192185452,
79.495912358085));
#207825=CARTESIAN_POINT('Ctrl Pts',(-38.2709383730497,-84.1652783971981,
80.500014999148));
#207826=CARTESIAN_POINT('Ctrl Pts',(-38.2841616945643,-83.8098556447903,
80.9137044893147));
#207827=CARTESIAN_POINT('Ctrl Pts',(-38.3176332551114,-82.8513592357023,
81.8849868252109));
#207828=CARTESIAN_POINT('Ctrl Pts',(-38.3379297369795,-82.216444701061,
82.4071404513844));
#207829=CARTESIAN_POINT('Ctrl Pts',(-38.368073150965,-81.1831583171694,
83.0907477405221));
#207830=CARTESIAN_POINT('Ctrl Pts',(-38.3782385943083,-80.8215881332394,
83.3032741780965));
#207831=CARTESIAN_POINT('Ctrl Pts',(-38.3987282946612,-80.0768318302408,
83.6894003568694));
#207832=CARTESIAN_POINT('Ctrl Pts',(-38.4090386083604,-79.6941400064729,
83.8626621797839));
#207833=CARTESIAN_POINT('Ctrl Pts',(-38.4193726539769,-79.3030589811838,
84.0152321705287));
#207834=CARTESIAN_POINT('',(-38.7170569083159,-79.302583977372,84.0154504430313));
#207835=CARTESIAN_POINT('',(-38.4175364832709,-79.30270960864,84.0153684626757));
#207836=CARTESIAN_POINT('Ctrl Pts',(-38.2588685144218,-85.9425570350203,
68.4641091549302));
#207837=CARTESIAN_POINT('Ctrl Pts',(-38.2753921140801,-86.2019757173487,
69.0920037570412));
#207838=CARTESIAN_POINT('Ctrl Pts',(-38.2919909110401,-86.4068721094222,
69.7410687161471));
#207839=CARTESIAN_POINT('Ctrl Pts',(-38.3247086479941,-86.7021386154924,
71.062960663399));
#207840=CARTESIAN_POINT('Ctrl Pts',(-38.3408123281424,-86.7926840996756,
71.7331880602675));
#207841=CARTESIAN_POINT('Ctrl Pts',(-38.368176471662,-86.847564808067,72.8567104434098));
#207842=CARTESIAN_POINT('Ctrl Pts',(-38.3791668041158,-86.8438920145194,
73.3068378553918));
#207843=CARTESIAN_POINT('Ctrl Pts',(-38.404419780308,-86.7762256212567,
74.3443579761178));
#207844=CARTESIAN_POINT('Ctrl Pts',(-38.4185812414996,-86.6938852844249,
74.9293606887009));
#207845=CARTESIAN_POINT('Ctrl Pts',(-38.4507641769267,-86.4092982467322,
76.235443956933));
#207846=CARTESIAN_POINT('Ctrl Pts',(-38.4690337585595,-86.1816326587067,
76.9484258103896));
#207847=CARTESIAN_POINT('Ctrl Pts',(-38.5056409803773,-85.5900645712485,
78.3336123336522));
#207848=CARTESIAN_POINT('Ctrl Pts',(-38.5237690303284,-85.2252868599235,
79.0017114320046));
#207849=CARTESIAN_POINT('Ctrl Pts',(-38.5602504821626,-84.3803056288327,
80.2477433922791));
#207850=CARTESIAN_POINT('Ctrl Pts',(-38.5785684555978,-83.9041334058414,
80.8242712373526));
#207851=CARTESIAN_POINT('Ctrl Pts',(-38.616219007985,-82.8062023510351,
81.9235023377032));
#207852=CARTESIAN_POINT('Ctrl Pts',(-38.6355332715926,-82.1785627775367,
82.4349754727978));
#207853=CARTESIAN_POINT('Ctrl Pts',(-38.6653949765361,-81.1583426766389,
83.1056540435057));
#207854=CARTESIAN_POINT('Ctrl Pts',(-38.6755171178595,-80.8012577923637,
83.3144877599883));
#207855=CARTESIAN_POINT('Ctrl Pts',(-38.6956648674306,-80.066181046409,
83.6942191651638));
#207856=CARTESIAN_POINT('Ctrl Pts',(-38.7056764744094,-79.6886661336525,
83.8648002743088));
#207857=CARTESIAN_POINT('Ctrl Pts',(-38.7156810426872,-79.3029942695161,
84.0152574158675));
#207858=CARTESIAN_POINT('Origin',(-33.5526503323277,-74.999949493375,72.9851176492631));
#207859=CARTESIAN_POINT('',(-36.4450710296185,-85.9425570350204,68.4641091549303));
#207860=CARTESIAN_POINT('Ctrl Pts',(-38.2588681851947,-85.9425518661828,
68.4640966443435));
#207861=CARTESIAN_POINT('Ctrl Pts',(-38.2416125443476,-85.6716394289052,
67.8083847872759));
#207862=CARTESIAN_POINT('Ctrl Pts',(-38.2246992567495,-85.3423424744358,
67.178359752856));
#207863=CARTESIAN_POINT('Ctrl Pts',(-38.1907913902441,-84.5847639064926,
66.0001810544474));
#207864=CARTESIAN_POINT('Ctrl Pts',(-38.1738496662569,-84.1607033288119,
65.4526156031358));
#207865=CARTESIAN_POINT('Ctrl Pts',(-38.1458700494748,-83.3784173735093,
64.6069461298567));
#207866=CARTESIAN_POINT('Ctrl Pts',(-38.1348186763153,-83.0460512346096,
64.2872598648431));
#207867=CARTESIAN_POINT('Ctrl Pts',(-38.1012115696759,-81.9879336323315,
63.382191774255));
#207868=CARTESIAN_POINT('Ctrl Pts',(-38.0783453797895,-81.2109640053625,
62.8623023649894));
#207869=CARTESIAN_POINT('Ctrl Pts',(-38.0372470656261,-79.7022677703556,
62.0924956090233));
#207870=CARTESIAN_POINT('Ctrl Pts',(-38.0189916508675,-78.9915459718726,
61.8124646475773));
#207871=CARTESIAN_POINT('Ctrl Pts',(-37.9851891809974,-77.6600567554545,
61.4312455378352));
#207872=CARTESIAN_POINT('Ctrl Pts',(-37.9698558123282,-77.0486597540841,
61.3073215263093));
#207873=CARTESIAN_POINT('Ctrl Pts',(-37.9455221116277,-76.0534310284601,
61.1861967898652));
#207874=CARTESIAN_POINT('Ctrl Pts',(-37.9363633125234,-75.6745141071768,
61.1584816112066));
#207875=CARTESIAN_POINT('Ctrl Pts',(-37.9052919782341,-74.3934819972736,
61.1265564688018));
#207876=CARTESIAN_POINT('Ctrl Pts',(-37.8830606873922,-73.4924271033512,
61.2071451995449));
#207877=CARTESIAN_POINT('Ctrl Pts',(-37.842452469934,-71.8611039360052,
61.543465613656));
#207878=CARTESIAN_POINT('Ctrl Pts',(-37.8240751982879,-71.1295998622464,
61.7697642269712));
#207879=CARTESIAN_POINT('Ctrl Pts',(-37.796023696184,-70.0741530811529,
62.211937365696));
#207880=CARTESIAN_POINT('Ctrl Pts',(-37.7866509684566,-69.7305847509062,
62.3757501858922));
#207881=CARTESIAN_POINT('Ctrl Pts',(-37.7589211397404,-68.7375101769051,
62.9094039216394));
#207882=CARTESIAN_POINT('Ctrl Pts',(-37.7409140989774,-68.1144577391385,
63.3244676823421));
#207883=CARTESIAN_POINT('Ctrl Pts',(-37.7035748245326,-66.9278199909356,
64.2884395531698));
#207884=CARTESIAN_POINT('Ctrl Pts',(-37.6841954035802,-66.3712896182925,
64.8403214554513));
#207885=CARTESIAN_POINT('Ctrl Pts',(-37.6463117908446,-65.3853821197504,
66.0333703196312));
#207886=CARTESIAN_POINT('Ctrl Pts',(-37.6278172025649,-64.9559563641628,
66.6696679463548));
#207887=CARTESIAN_POINT('Ctrl Pts',(-37.5996252819912,-64.4098558886715,
67.6771441788257));
#207888=CARTESIAN_POINT('Ctrl Pts',(-37.5902278724741,-64.2449134677174,
68.0198518845031));
#207889=CARTESIAN_POINT('Ctrl Pts',(-37.5624044606299,-63.8053665947533,
69.0582574537565));
#207890=CARTESIAN_POINT('Ctrl Pts',(-37.5443334318455,-63.5798328803693,
69.7726645123915));
#207891=CARTESIAN_POINT('Ctrl Pts',(-37.5068934288594,-63.2593820722814,
71.2676036407564));
#207892=CARTESIAN_POINT('Ctrl Pts',(-37.4874816554964,-63.17164387106,72.0459921353528));
#207893=CARTESIAN_POINT('Ctrl Pts',(-37.4495292111963,-63.1510148244988,
73.5937510368514));
#207894=CARTESIAN_POINT('Ctrl Pts',(-37.4309908956369,-63.2152494585919,
74.3593589166442));
#207895=CARTESIAN_POINT('Ctrl Pts',(-37.4027658154795,-63.4212676048063,
75.4867988277926));
#207896=CARTESIAN_POINT('Ctrl Pts',(-37.3933733120741,-63.5074246657974,
75.8567296161491));
#207897=CARTESIAN_POINT('Ctrl Pts',(-37.3655429605183,-63.8156143655937,
76.9411140168159));
#207898=CARTESIAN_POINT('Ctrl Pts',(-37.3474663305294,-64.0876986611687,
77.6393676233608));
#207899=CARTESIAN_POINT('Ctrl Pts',(-37.3100234317308,-64.7751675108902,
79.0054966869767));
#207900=CARTESIAN_POINT('Ctrl Pts',(-37.2906186537663,-65.1948023495195,
79.6671992307357));
#207901=CARTESIAN_POINT('Ctrl Pts',(-37.2527293925608,-66.1485614315836,
80.8857195033305));
#207902=CARTESIAN_POINT('Ctrl Pts',(-37.2342357545949,-66.6779437734176,
81.4415239738006));
#207903=CARTESIAN_POINT('Ctrl Pts',(-37.2060940265001,-67.5441090173429,
82.1902448480956));
#207904=CARTESIAN_POINT('Ctrl Pts',(-37.1967331731798,-67.8426842846673,
82.4242636898797));
#207905=CARTESIAN_POINT('Ctrl Pts',(-37.1689807489343,-68.7619521988769,
83.0760387798127));
#207906=CARTESIAN_POINT('Ctrl Pts',(-37.1509553911568,-69.4115327090771,
83.449767619805));
#207907=CARTESIAN_POINT('Ctrl Pts',(-37.1136099924952,-70.8038262478118,
84.0839709447713));
#207908=CARTESIAN_POINT('Ctrl Pts',(-37.0942546423633,-71.5460236827676,
84.3368746469189));
#207909=CARTESIAN_POINT('Ctrl Pts',(-37.0565352279133,-73.051858134729,
84.6884955663936));
#207910=CARTESIAN_POINT('Ctrl Pts',(-37.0381506453932,-73.8110757932122,
84.789807429784));
#207911=CARTESIAN_POINT('Ctrl Pts',(-37.010166306195,-74.9534477350529,
84.8308601815569));
#207912=CARTESIAN_POINT('Ctrl Pts',(-37.0008486703605,-75.3325853469066,
84.8262802307058));
#207913=CARTESIAN_POINT('Ctrl Pts',(-36.9732219453808,-76.4571279179261,
84.7586369880659));
#207914=CARTESIAN_POINT('Ctrl Pts',(-36.9552807147453,-77.1974784827877,
84.6431618483784));
#207915=CARTESIAN_POINT('Ctrl Pts',(-36.918216632995,-78.67545719408,84.266756192141));
#207916=CARTESIAN_POINT('Ctrl Pts',(-36.8990633551225,-79.4081973934672,
84.0011092457016));
#207917=CARTESIAN_POINT('Ctrl Pts',(-36.861678037431,-80.7968427730354,
83.3367662934791));
#207918=CARTESIAN_POINT('Ctrl Pts',(-36.843434072982,-81.450762252324,82.9424075977943));
#207919=CARTESIAN_POINT('Ctrl Pts',(-36.8156208183404,-82.3667480570503,
82.2616680953195));
#207920=CARTESIAN_POINT('Ctrl Pts',(-36.8063331633932,-82.6601959543437,
82.0208651388703));
#207921=CARTESIAN_POINT('Ctrl Pts',(-36.7788204255325,-83.4957607368464,
81.2651954505709));
#207922=CARTESIAN_POINT('Ctrl Pts',(-36.7609605030719,-84.0012571101229,
80.71266317542));
#207923=CARTESIAN_POINT('Ctrl Pts',(-36.7239099388123,-84.9232542401603,
79.4906702030789));
#207924=CARTESIAN_POINT('Ctrl Pts',(-36.7046775421896,-85.3319454568592,
78.8198451706126));
#207925=CARTESIAN_POINT('Ctrl Pts',(-36.6673068359652,-86.0007663416384,
77.4281497084285));
#207926=CARTESIAN_POINT('Ctrl Pts',(-36.6491525986536,-86.2633684645749,
76.7125705098767));
#207927=CARTESIAN_POINT('Ctrl Pts',(-36.6214428496755,-86.5514603764109,
75.6094128012789));
#207928=CARTESIAN_POINT('Ctrl Pts',(-36.612172041046,-86.6296694441817,
75.2376588382518));
#207929=CARTESIAN_POINT('Ctrl Pts',(-36.5847295931906,-86.8083033491122,
74.1255289639083));
#207930=CARTESIAN_POINT('Ctrl Pts',(-36.5669174831325,-86.8567129957862,
73.3787156042629));
#207931=CARTESIAN_POINT('Ctrl Pts',(-36.5299300095861,-86.8111017792754,
71.848643033187));
#207932=CARTESIAN_POINT('Ctrl Pts',(-36.5107101518215,-86.709953528322,
71.0692126138227));
#207933=CARTESIAN_POINT('Ctrl Pts',(-36.4761290010132,-86.3863504026881,
69.6764751873896));
#207934=CARTESIAN_POINT('Ctrl Pts',(-36.4607107367829,-86.1890117344204,
69.0606258515277));
#207935=CARTESIAN_POINT('Ctrl Pts',(-36.4450710296185,-85.9425570350204,
68.4641091549303));
#207936=CARTESIAN_POINT('',(-36.143425535889,-85.9425570350204,68.4641091549303));
#207937=CARTESIAN_POINT('',(-33.5526503323277,-85.9425570350204,68.4641091549303));
#207938=CARTESIAN_POINT('Ctrl Pts',(-36.143425535889,-85.9425570350204,
68.4641091549303));
#207939=CARTESIAN_POINT('Ctrl Pts',(-36.148238507304,-86.0174834758539,
68.6454604259047));
#207940=CARTESIAN_POINT('Ctrl Pts',(-36.1530665592699,-86.0879280851577,
68.8287383180261));
#207941=CARTESIAN_POINT('Ctrl Pts',(-36.167266731233,-86.281155707984,69.371435524502));
#207942=CARTESIAN_POINT('Ctrl Pts',(-36.1766643368532,-86.3912228849641,
69.7350096114226));
#207943=CARTESIAN_POINT('Ctrl Pts',(-36.2030542231982,-86.6518386352883,
70.7735096421015));
#207944=CARTESIAN_POINT('Ctrl Pts',(-36.2197568716503,-86.7610399882958,
71.4572166260671));
#207945=CARTESIAN_POINT('Ctrl Pts',(-36.2552103712041,-86.8635398875244,
72.9007540960301));
#207946=CARTESIAN_POINT('Ctrl Pts',(-36.2739887581872,-86.8447212800773,
73.6583681292809));
#207947=CARTESIAN_POINT('Ctrl Pts',(-36.3103716158341,-86.6664108020393,
75.1302890120472));
#207948=CARTESIAN_POINT('Ctrl Pts',(-36.3279354581554,-86.5128221102881,
75.8420129729576));
#207949=CARTESIAN_POINT('Ctrl Pts',(-36.3641725418675,-86.0709158492975,
77.2480084534117));
#207950=CARTESIAN_POINT('Ctrl Pts',(-36.3827138424614,-85.7798828500403,
77.9380541339613));
#207951=CARTESIAN_POINT('Ctrl Pts',(-36.4191576989442,-85.072124697069,
79.2531561708606));
#207952=CARTESIAN_POINT('Ctrl Pts',(-36.4372829124874,-84.6571567029495,
79.8753547680538));
#207953=CARTESIAN_POINT('Ctrl Pts',(-36.4650541363608,-83.9463039397956,
80.7496371837122));
#207954=CARTESIAN_POINT('Ctrl Pts',(-36.4744653456105,-83.6921109467192,
81.0331826818526));
#207955=CARTESIAN_POINT('Ctrl Pts',(-36.5030580974817,-82.8746401466155,
81.8610580580722));
#207956=CARTESIAN_POINT('Ctrl Pts',(-36.5219004939314,-82.2706782802858,
82.3621948471306));
#207957=CARTESIAN_POINT('Ctrl Pts',(-36.5594359775069,-81.0014393595734,
83.2185000153491));
#207958=CARTESIAN_POINT('Ctrl Pts',(-36.5779561060125,-80.3429151466602,
83.5772242458362));
#207959=CARTESIAN_POINT('Ctrl Pts',(-36.6142671885997,-78.9707546081985,
84.1639642071798));
#207960=CARTESIAN_POINT('Ctrl Pts',(-36.6322663079185,-78.2604946666755,
84.3913768263397));
#207961=CARTESIAN_POINT('Ctrl Pts',(-36.6598749832277,-77.1618598961551,
84.6320549198793));
#207962=CARTESIAN_POINT('Ctrl Pts',(-36.6692493346064,-76.7864044560539,
84.6955225510577));
#207963=CARTESIAN_POINT('Ctrl Pts',(-36.6977320732928,-75.6317722112526,
84.8338736460224));
#207964=CARTESIAN_POINT('Ctrl Pts',(-36.7164809648073,-74.8476831316937,
84.8497303991984));
#207965=CARTESIAN_POINT('Ctrl Pts',(-36.7538592000449,-73.3205657064729,
84.7291228904894));
#207966=CARTESIAN_POINT('Ctrl Pts',(-36.7723383793587,-72.5806394466273,
84.5992872690723));
#207967=CARTESIAN_POINT('Ctrl Pts',(-36.8094626036945,-71.1035223093137,
84.1927196477861));
#207968=CARTESIAN_POINT('Ctrl Pts',(-36.8282950950502,-70.3715189689159,
83.9107809543057));
#207969=CARTESIAN_POINT('Ctrl Pts',(-36.856734308558,-69.3326466704178,
83.3873696220951));
#207970=CARTESIAN_POINT('Ctrl Pts',(-36.8660725857096,-69.0010560135803,
83.1997368064791));
#207971=CARTESIAN_POINT('Ctrl Pts',(-36.8943966804287,-68.0179528155365,
82.5790341463043));
#207972=CARTESIAN_POINT('Ctrl Pts',(-36.9130538277333,-67.3997932428991,
82.0971503431833));
#207973=CARTESIAN_POINT('Ctrl Pts',(-36.9502644985451,-66.2915970856974,
81.0414966619182));
#207974=CARTESIAN_POINT('Ctrl Pts',(-36.9686368114208,-65.7997256006237,
80.4748795771567));
#207975=CARTESIAN_POINT('Ctrl Pts',(-37.0047206435837,-64.9305165687805,
79.2576607293675));
#207976=CARTESIAN_POINT('Ctrl Pts',(-37.0226503340936,-64.5548889939857,
78.6099719727269));
#207977=CARTESIAN_POINT('Ctrl Pts',(-37.0501221059068,-64.0838323661145,
77.5854841283829));
#207978=CARTESIAN_POINT('Ctrl Pts',(-37.0594257097561,-63.9416231268765,
77.2322817378447));
#207979=CARTESIAN_POINT('Ctrl Pts',(-37.0944558615515,-63.4683337741028,
75.8708371110155));
#207980=CARTESIAN_POINT('Ctrl Pts',(-37.1196682747815,-63.2562408457119,
74.8265431874806));
#207981=CARTESIAN_POINT('Ctrl Pts',(-37.1548355702015,-63.1608567503633,
73.3872393056425));
#207982=CARTESIAN_POINT('Ctrl Pts',(-37.1641520237652,-63.1540469129996,
73.005445881158));
#207983=CARTESIAN_POINT('Ctrl Pts',(-37.1960864508945,-63.194341250831,
71.6849857454238));
#207984=CARTESIAN_POINT('Ctrl Pts',(-37.2185220904404,-63.3346533868927,
70.7527189972505));
#207985=CARTESIAN_POINT('Ctrl Pts',(-37.2507210153804,-63.6847111884255,
69.4792801883886));
#207986=CARTESIAN_POINT('Ctrl Pts',(-37.2600339386413,-63.8034555614583,
69.1167795582661));
#207987=CARTESIAN_POINT('Ctrl Pts',(-37.2905721356825,-64.2537199352495,
67.93790366409));
#207988=CARTESIAN_POINT('Ctrl Pts',(-37.3115906708213,-64.6587791099737,
67.1527919767579));
#207989=CARTESIAN_POINT('Ctrl Pts',(-37.3423292207609,-65.357995683196,
66.1034389200866));
#207990=CARTESIAN_POINT('Ctrl Pts',(-37.3516320206513,-65.5839750211042,
65.797336342476));
#207991=CARTESIAN_POINT('Ctrl Pts',(-37.3856258642121,-66.467624739571,
64.7137289705806));
#207992=CARTESIAN_POINT('Ctrl Pts',(-37.4098726886797,-67.2100234473301,
64.0110721617912));
#207993=CARTESIAN_POINT('Ctrl Pts',(-37.4440566413501,-68.3410826462592,
63.1879365471086));
#207994=CARTESIAN_POINT('Ctrl Pts',(-37.4533880966028,-68.6596995598004,
62.9787947945492));
#207995=CARTESIAN_POINT('Ctrl Pts',(-37.4830414748069,-69.7116943037478,
62.3587099843057));
#207996=CARTESIAN_POINT('Ctrl Pts',(-37.5031438140031,-70.4789133305202,
62.010309049287));
#207997=CARTESIAN_POINT('Ctrl Pts',(-37.5329543904772,-71.636968187707,
61.6266533792021));
#207998=CARTESIAN_POINT('Ctrl Pts',(-37.5422743339172,-72.0029436119635,
61.5246504221834));
#207999=CARTESIAN_POINT('Ctrl Pts',(-37.5694744519505,-73.087747807898,
61.2778252619525));
#208000=CARTESIAN_POINT('Ctrl Pts',(-37.5870320088167,-73.8158612059384,
61.1819339459102));
#208001=CARTESIAN_POINT('Ctrl Pts',(-37.6239248535313,-75.3301887145771,
61.1241062397469));
#208002=CARTESIAN_POINT('Ctrl Pts',(-37.6432534817882,-76.1132600710327,
61.1718543800873));
#208003=CARTESIAN_POINT('Ctrl Pts',(-37.6766178299039,-77.4672112260184,
61.3903106970509));
#208004=CARTESIAN_POINT('Ctrl Pts',(-37.6908179431224,-78.0407413815151,
61.5273467136123));
#208005=CARTESIAN_POINT('Ctrl Pts',(-37.7243121371928,-79.3470851552171,
61.9445169355828));
#208006=CARTESIAN_POINT('Ctrl Pts',(-37.7436781430201,-80.0670499423904,
62.2558609425313));
#208007=CARTESIAN_POINT('Ctrl Pts',(-37.7784709687326,-81.3158038597836,
62.9497977401581));
#208008=CARTESIAN_POINT('Ctrl Pts',(-37.7940996341551,-81.8539485181105,
63.3093562021165));
#208009=CARTESIAN_POINT('Ctrl Pts',(-37.8221659870852,-82.7499128002765,
64.020411671817));
#208010=CARTESIAN_POINT('Ctrl Pts',(-37.8344691414043,-83.1198651551587,
64.3540776172099));
#208011=CARTESIAN_POINT('Ctrl Pts',(-37.86522554667,-83.9940875726504,65.2486559849823));
#208012=CARTESIAN_POINT('Ctrl Pts',(-37.8833718986528,-84.4678644238347,
65.8362753272456));
#208013=CARTESIAN_POINT('Ctrl Pts',(-37.9203741409185,-85.2989408740914,
67.0959335227594));
#208014=CARTESIAN_POINT('Ctrl Pts',(-37.9391486654917,-85.6538782424784,
67.7653936501169));
#208015=CARTESIAN_POINT('Ctrl Pts',(-37.9576288901553,-85.9425570350206,
68.4641091549307));
#208016=CARTESIAN_POINT('Origin',(-33.5526503323277,-74.999949493375,72.9851176492631));
#208017=CARTESIAN_POINT('',(-34.329622639475,-85.9425570350204,68.4641091549303));
#208018=CARTESIAN_POINT('',(-34.6308727573024,-85.9425570350204,68.4641091549303));
#208019=CARTESIAN_POINT('',(-33.5526503323277,-85.9425570350204,68.4641091549303));
#208020=CARTESIAN_POINT('Ctrl Pts',(-34.329622639475,-85.9425570350204,
68.4641091549303));
#208021=CARTESIAN_POINT('Ctrl Pts',(-34.3331454855336,-85.9971435846138,
68.5962299394856));
#208022=CARTESIAN_POINT('Ctrl Pts',(-34.3366615064198,-86.0493527669876,
68.7293767663076));
#208023=CARTESIAN_POINT('Ctrl Pts',(-34.3589661420323,-86.3663168730277,
69.582934301803));
#208024=CARTESIAN_POINT('Ctrl Pts',(-34.3775289583419,-86.5628967428812,
70.3266565489548));
#208025=CARTESIAN_POINT('Ctrl Pts',(-34.4117140406206,-86.785736124185,
71.6965614893729));
#208026=CARTESIAN_POINT('Ctrl Pts',(-34.4271139387984,-86.8370621353701,
72.3158541704069));
#208027=CARTESIAN_POINT('Ctrl Pts',(-34.4515943340047,-86.8411879378932,
73.3166789929037));
#208028=CARTESIAN_POINT('Ctrl Pts',(-34.460840960197,-86.824425079426,73.6969031311766));
#208029=CARTESIAN_POINT('Ctrl Pts',(-34.4882992586455,-86.7209055734037,
74.816013838025));
#208030=CARTESIAN_POINT('Ctrl Pts',(-34.5066650536923,-86.5828342577236,
75.5482721060436));
#208031=CARTESIAN_POINT('Ctrl Pts',(-34.5435021566419,-86.1693837093553,
76.983421397808));
#208032=CARTESIAN_POINT('Ctrl Pts',(-34.5616096469221,-85.8937474926455,
77.6827616992859));
#208033=CARTESIAN_POINT('Ctrl Pts',(-34.5991461705954,-85.1995290142402,
79.0481026945294));
#208034=CARTESIAN_POINT('Ctrl Pts',(-34.6185603487462,-84.7771069687462,
79.7080934417855));
#208035=CARTESIAN_POINT('Ctrl Pts',(-34.6469680849255,-84.0569094913357,
80.6203317292538));
#208036=CARTESIAN_POINT('Ctrl Pts',(-34.6562049432673,-83.806817852358,
80.9074966497412));
#208037=CARTESIAN_POINT('Ctrl Pts',(-34.6836624447065,-83.0271662173277,
81.7200941635885));
#208038=CARTESIAN_POINT('Ctrl Pts',(-34.7020276571441,-82.4613395161597,
82.2081144724638));
#208039=CARTESIAN_POINT('Ctrl Pts',(-34.7388066803891,-81.242820807903,
83.0731006593034));
#208040=CARTESIAN_POINT('Ctrl Pts',(-34.7568400152815,-80.5925035909137,
83.4476308918892));
#208041=CARTESIAN_POINT('Ctrl Pts',(-34.7942258548029,-79.1995047284768,
84.0826697742791));
#208042=CARTESIAN_POINT('Ctrl Pts',(-34.8135838749069,-78.4574257329447,
84.3357909980717));
#208043=CARTESIAN_POINT('Ctrl Pts',(-34.841917391454,-77.3250717421524,
84.6005797464628));
#208044=CARTESIAN_POINT('Ctrl Pts',(-34.8511227011814,-76.9503498702266,
84.6693417411533));
#208045=CARTESIAN_POINT('Ctrl Pts',(-34.8793707315971,-75.7972408508684,
84.8239127022759));
#208046=CARTESIAN_POINT('Ctrl Pts',(-34.8985781208994,-75.0131129118346,
84.8507215233565));
#208047=CARTESIAN_POINT('Ctrl Pts',(-34.9361050064331,-73.4841460455405,
84.7513541681887));
#208048=CARTESIAN_POINT('Ctrl Pts',(-34.9540641051862,-72.7424940300257,
84.6318286806867));
#208049=CARTESIAN_POINT('Ctrl Pts',(-34.9896687620346,-71.3260212041991,
84.2630799997661));
#208050=CARTESIAN_POINT('Ctrl Pts',(-35.0072527034101,-70.6526056524081,
84.0210036619251));
#208051=CARTESIAN_POINT('Ctrl Pts',(-35.0430839339609,-69.3159397063232,
83.3990514534641));
#208052=CARTESIAN_POINT('Ctrl Pts',(-35.0612722237815,-68.6592371791954,
83.0127474950601));
#208053=CARTESIAN_POINT('Ctrl Pts',(-35.0959719163052,-67.5063999244693,
82.1757879512153));
#208054=CARTESIAN_POINT('Ctrl Pts',(-35.1122898947841,-67.0025037569717,
81.7408343349271));
#208055=CARTESIAN_POINT('Ctrl Pts',(-35.1468602730768,-66.0020639810478,
80.7184797408343));
#208056=CARTESIAN_POINT('Ctrl Pts',(-35.1652217936896,-65.5207497281352,
80.1203545918229));
#208057=CARTESIAN_POINT('Ctrl Pts',(-35.1931558519464,-64.8918673622647,
79.1618177588344));
#208058=CARTESIAN_POINT('Ctrl Pts',(-35.2024619063936,-64.6986035695765,
78.8338115681298));
#208059=CARTESIAN_POINT('Ctrl Pts',(-35.2263409482913,-64.2417323022475,
77.9652779921287));
#208060=CARTESIAN_POINT('Ctrl Pts',(-35.2407033747601,-64.0028852075868,
77.4129627151134));
#208061=CARTESIAN_POINT('Ctrl Pts',(-35.2737592115932,-63.5563632386513,
76.1181001861888));
#208062=CARTESIAN_POINT('Ctrl Pts',(-35.2925525979034,-63.3771186653348,
75.3686101024677));
#208063=CARTESIAN_POINT('Ctrl Pts',(-35.3301955770658,-63.1647543079954,
73.8330157568421));
#208064=CARTESIAN_POINT('Ctrl Pts',(-35.3487882818884,-63.1345993688963,
73.050276214966));
#208065=CARTESIAN_POINT('Ctrl Pts',(-35.3859053287861,-63.2269862620111,
71.5228495536105));
#208066=CARTESIAN_POINT('Ctrl Pts',(-35.4042500264341,-63.3430018964623,
70.7813772379834));
#208067=CARTESIAN_POINT('Ctrl Pts',(-35.4403055803372,-63.7132183521813,
69.331527780735));
#208068=CARTESIAN_POINT('Ctrl Pts',(-35.4582331517031,-63.9663547939685,
68.6263557777856));
#208069=CARTESIAN_POINT('Ctrl Pts',(-35.4857043494334,-64.445988734284,
67.605651120122));
#208070=CARTESIAN_POINT('Ctrl Pts',(-35.4950012797736,-64.624177266005,
67.269516336227));
#208071=CARTESIAN_POINT('Ctrl Pts',(-35.5311899500532,-65.3837890589454,
65.9895734885102));
#208072=CARTESIAN_POINT('Ctrl Pts',(-35.5575682690911,-66.0803483339916,
65.1207108285158));
#208073=CARTESIAN_POINT('Ctrl Pts',(-35.5939937242823,-67.1662192011089,
64.0992137072605));
#208074=CARTESIAN_POINT('Ctrl Pts',(-35.6033388806798,-67.4574982581706,
63.8506745030953));
#208075=CARTESIAN_POINT('Ctrl Pts',(-35.6279078702261,-68.2611781331839,
63.2296149644293));
#208076=CARTESIAN_POINT('Ctrl Pts',(-35.643092677736,-68.7922891015213,
62.8833442566644));
#208077=CARTESIAN_POINT('Ctrl Pts',(-35.6775470584763,-70.0365630454112,
62.2074533387053));
#208078=CARTESIAN_POINT('Ctrl Pts',(-35.6967970925699,-70.759980699616,
61.9028829891663));
#208079=CARTESIAN_POINT('Ctrl Pts',(-35.7249389510534,-71.8715815101032,
61.5597880547802));
#208080=CARTESIAN_POINT('Ctrl Pts',(-35.7341115011194,-72.2402065668481,
61.4651931106097));
#208081=CARTESIAN_POINT('Ctrl Pts',(-35.7618677759948,-73.3604526520311,
61.2345862663303));
#208082=CARTESIAN_POINT('Ctrl Pts',(-35.7806552631901,-74.1212918052034,
61.1533432880975));
#208083=CARTESIAN_POINT('Ctrl Pts',(-35.8215037729031,-75.794586805878,
61.1370451384279));
#208084=CARTESIAN_POINT('Ctrl Pts',(-35.8433144636235,-76.7025343150823,
61.2331185731713));
#208085=CARTESIAN_POINT('Ctrl Pts',(-35.8749641583077,-77.9610258826306,
61.5153134448595));
#208086=CARTESIAN_POINT('Ctrl Pts',(-35.8843204616723,-78.3273548386835,
61.6161794722982));
#208087=CARTESIAN_POINT('Ctrl Pts',(-35.9082821378525,-79.2562739356596,
61.9207031895175));
#208088=CARTESIAN_POINT('Ctrl Pts',(-35.9226926456173,-79.8094247629693,
62.1496890346621));
#208089=CARTESIAN_POINT('Ctrl Pts',(-35.9558505891654,-81.0238912889785,
62.7638346708611));
#208090=CARTESIAN_POINT('Ctrl Pts',(-35.9746959834488,-81.6699859002282,
63.1732319549594));
#208091=CARTESIAN_POINT('Ctrl Pts',(-36.0183948795527,-83.0752451939547,
64.2670087383948));
#208092=CARTESIAN_POINT('Ctrl Pts',(-36.0428739043318,-83.7943899375482,
64.9930187511748));
#208093=CARTESIAN_POINT('Ctrl Pts',(-36.0773872760601,-84.6432282252551,
66.105229667036));
#208094=CARTESIAN_POINT('Ctrl Pts',(-36.0868193645644,-84.8598640899545,
66.4194669793043));
#208095=CARTESIAN_POINT('Ctrl Pts',(-36.1119948092705,-85.4014006277824,
67.2923975823855));
#208096=CARTESIAN_POINT('Ctrl Pts',(-36.1276008548743,-85.6962046419724,
67.8678400796899));
#208097=CARTESIAN_POINT('Ctrl Pts',(-36.143425535889,-85.9425570350204,
68.4641091549303));
#208098=CARTESIAN_POINT('Ctrl Pts',(-36.4450710296185,-85.9425570350204,
68.4641091549303));
#208099=CARTESIAN_POINT('Ctrl Pts',(-36.4423012432504,-85.8989099986937,
68.3584662680661));
#208100=CARTESIAN_POINT('Ctrl Pts',(-36.4395263830693,-85.8537224637666,
68.2534296903723));
#208101=CARTESIAN_POINT('Ctrl Pts',(-36.4214766063348,-85.5503858269364,
67.5755721521631));
#208102=CARTESIAN_POINT('Ctrl Pts',(-36.4060778793579,-85.2485270709375,
67.0234440471119));
#208103=CARTESIAN_POINT('Ctrl Pts',(-36.3817313446517,-84.6962406003481,
66.1802449180317));
#208104=CARTESIAN_POINT('Ctrl Pts',(-36.3726172947798,-84.4730327659579,
65.8728010050208));
#208105=CARTESIAN_POINT('Ctrl Pts',(-36.345519548382,-83.7702764260099,
64.9967402335534));
#208106=CARTESIAN_POINT('Ctrl Pts',(-36.3273777496255,-83.2515338997932,
64.4619638613415));
#208107=CARTESIAN_POINT('Ctrl Pts',(-36.2901603729948,-82.0909634028798,
63.4714504751788));
#208108=CARTESIAN_POINT('Ctrl Pts',(-36.271485138386,-81.446953432645,63.0237682451142));
#208109=CARTESIAN_POINT('Ctrl Pts',(-36.2334585080771,-80.0790776588067,
62.2614727233239));
#208110=CARTESIAN_POINT('Ctrl Pts',(-36.2141711485334,-79.3584738918224,
61.9489330039573));
#208111=CARTESIAN_POINT('Ctrl Pts',(-36.185995790235,-78.2508598472694,
61.5940770740617));
#208112=CARTESIAN_POINT('Ctrl Pts',(-36.1768518249844,-77.8840634175721,
61.4957264208434));
#208113=CARTESIAN_POINT('Ctrl Pts',(-36.1464433664546,-76.6574615990018,
61.2292836392938));
#208114=CARTESIAN_POINT('Ctrl Pts',(-36.1248802104232,-75.7837662242147,
61.138911762691));
#208115=CARTESIAN_POINT('Ctrl Pts',(-36.0849816876455,-74.1456047686891,
61.1516163766496));
#208116=CARTESIAN_POINT('Ctrl Pts',(-36.0666663650914,-73.3854313170334,
61.2311823622453));
#208117=CARTESIAN_POINT('Ctrl Pts',(-36.0386798573186,-72.2650520565091,
61.4592542871392));
#208118=CARTESIAN_POINT('Ctrl Pts',(-36.0293101717141,-71.8957823513543,
61.5531740009475));
#208119=CARTESIAN_POINT('Ctrl Pts',(-36.0016109162129,-70.817837671739,
61.8834274650834));
#208120=CARTESIAN_POINT('Ctrl Pts',(-35.9836295193508,-70.1262781175103,
62.1691612478175));
#208121=CARTESIAN_POINT('Ctrl Pts',(-35.9491086987731,-68.8750423125115,
62.830665325642));
#208122=CARTESIAN_POINT('Ctrl Pts',(-35.932609906165,-68.3113836752578,
63.1927497777215));
#208123=CARTESIAN_POINT('Ctrl Pts',(-35.9067635571126,-67.4778069486584,
63.833933339976));
#208124=CARTESIAN_POINT('Ctrl Pts',(-35.8974498608685,-67.1857983076346,
64.0819808722953));
#208125=CARTESIAN_POINT('Ctrl Pts',(-35.8609307481193,-66.0900369904637,
65.1082854467731));
#208126=CARTESIAN_POINT('Ctrl Pts',(-35.8332993448451,-65.3861858277439,
65.9846490465808));
#208127=CARTESIAN_POINT('Ctrl Pts',(-35.796660027315,-64.6218662135142,
67.2737141729382));
#208128=CARTESIAN_POINT('Ctrl Pts',(-35.7874270697126,-64.4438167182841,
67.6099149701739));
#208129=CARTESIAN_POINT('Ctrl Pts',(-35.7599128469347,-63.9647069729288,
68.6305736201635));
#208130=CARTESIAN_POINT('Ctrl Pts',(-35.7414774339647,-63.7119206907607,
69.3355937987189));
#208131=CARTESIAN_POINT('Ctrl Pts',(-35.7045641317483,-63.3422378550477,
70.7853929430686));
#208132=CARTESIAN_POINT('Ctrl Pts',(-35.6864703925755,-63.2264664906049,
71.5269927350631));
#208133=CARTESIAN_POINT('Ctrl Pts',(-35.64896276832,-63.1346231584062,73.0545522259459));
#208134=CARTESIAN_POINT('Ctrl Pts',(-35.6295395978061,-63.1650606577362,
73.8372882417922));
#208135=CARTESIAN_POINT('Ctrl Pts',(-35.591570688659,-63.3780004791115,
75.3729507917361));
#208136=CARTESIAN_POINT('Ctrl Pts',(-35.5729545372401,-63.5575613725005,
76.1225058437425));
#208137=CARTESIAN_POINT('Ctrl Pts',(-35.5392581543781,-64.0039247016326,
77.4152470367238));
#208138=CARTESIAN_POINT('Ctrl Pts',(-35.5244078500187,-64.2419660370971,
77.9655197990577));
#208139=CARTESIAN_POINT('Ctrl Pts',(-35.5004693491248,-64.6976848422838,
78.8321932270412));
#208140=CARTESIAN_POINT('Ctrl Pts',(-35.4912269110028,-64.8908981914762,
79.1602315944225));
#208141=CARTESIAN_POINT('Ctrl Pts',(-35.4632432077074,-65.5196493313512,
80.1188959326026));
#208142=CARTESIAN_POINT('Ctrl Pts',(-35.4443344478751,-66.0008935294722,
80.7171201449417));
#208143=CARTESIAN_POINT('Ctrl Pts',(-35.4090628193468,-67.0029332504941,
81.7414152575258));
#208144=CARTESIAN_POINT('Ctrl Pts',(-35.3929634040686,-67.5087898420713,
82.1779161630646));
#208145=CARTESIAN_POINT('Ctrl Pts',(-35.3581139196932,-68.6639077562523,
83.0156867835771));
#208146=CARTESIAN_POINT('Ctrl Pts',(-35.3393112272503,-69.320642967518,
83.401604946994));
#208147=CARTESIAN_POINT('Ctrl Pts',(-35.3033648638821,-70.6522332529131,
84.0204876789463));
#208148=CARTESIAN_POINT('Ctrl Pts',(-35.2863178546542,-71.3201557861807,
84.2608062216495));
#208149=CARTESIAN_POINT('Ctrl Pts',(-35.2506607664019,-72.7309324357505,
84.6295964062637));
#208150=CARTESIAN_POINT('Ctrl Pts',(-35.2321277475721,-73.4726974434984,
84.7498884682277));
#208151=CARTESIAN_POINT('Ctrl Pts',(-35.1977519682759,-74.8843898012942,
84.8429857086929));
#208152=CARTESIAN_POINT('Ctrl Pts',(-35.1817199062326,-75.5504459355787,
84.8307642657437));
#208153=CARTESIAN_POINT('Ctrl Pts',(-35.1472033483399,-76.9550789089867,
84.6862178346176));
#208154=CARTESIAN_POINT('Ctrl Pts',(-35.1288267557659,-77.6893151583641,
84.5395799832117));
#208155=CARTESIAN_POINT('Ctrl Pts',(-35.1015387546173,-78.7693740033933,
84.2152777009895));
#208156=CARTESIAN_POINT('Ctrl Pts',(-35.0923560388029,-79.1284330759511,
84.0883009357928));
#208157=CARTESIAN_POINT('Ctrl Pts',(-35.0646247563223,-80.1862319254944,
83.6558044667905));
#208158=CARTESIAN_POINT('Ctrl Pts',(-35.0458864998912,-80.8622097135662,
83.2999116846659));
#208159=CARTESIAN_POINT('Ctrl Pts',(-35.0089330498868,-82.1327502131304,
82.4655028259929));
#208160=CARTESIAN_POINT('Ctrl Pts',(-34.9908243354338,-82.7248219386633,
81.9896111615221));
#208161=CARTESIAN_POINT('Ctrl Pts',(-34.9541983172375,-83.8024995639809,
80.9383692959569));
#208162=CARTESIAN_POINT('Ctrl Pts',(-34.9358635852369,-84.2870193242917,
80.3668141566195));
#208163=CARTESIAN_POINT('Ctrl Pts',(-34.9086817659159,-84.9313639763156,
79.441992414841));
#208164=CARTESIAN_POINT('Ctrl Pts',(-34.8995626760387,-85.1332290555259,
79.1203332685521));
#208165=CARTESIAN_POINT('Ctrl Pts',(-34.8718816299111,-85.6947918522471,
78.1219625845443));
#208166=CARTESIAN_POINT('Ctrl Pts',(-34.8531275457829,-86.0046212701144,
77.4195302834456));
#208167=CARTESIAN_POINT('Ctrl Pts',(-34.8155821464385,-86.4891036128981,
75.9499447390178));
#208168=CARTESIAN_POINT('Ctrl Pts',(-34.7969745907575,-86.6596990821518,
75.1853692935595));
#208169=CARTESIAN_POINT('Ctrl Pts',(-34.7598582721029,-86.8436520623721,
73.6675037772388));
#208170=CARTESIAN_POINT('Ctrl Pts',(-34.7415620763333,-86.8631076912814,
72.9185736740377));
#208171=CARTESIAN_POINT('Ctrl Pts',(-34.7144123214472,-86.7857495694007,
71.7936797547871));
#208172=CARTESIAN_POINT('Ctrl Pts',(-34.7052924697797,-86.7414362950188,
71.4160111223995));
#208173=CARTESIAN_POINT('Ctrl Pts',(-34.6776234151376,-86.5532565853733,
70.2854655652956));
#208174=CARTESIAN_POINT('Ctrl Pts',(-34.6588754588823,-86.3544340290832,
69.5437961207658));
#208175=CARTESIAN_POINT('Ctrl Pts',(-34.6371431145356,-86.039740020247,
68.7049215467144));
#208176=CARTESIAN_POINT('Ctrl Pts',(-34.634004382883,-85.9921284957838,
68.5840914644261));
#208177=CARTESIAN_POINT('Ctrl Pts',(-34.6308727573024,-85.9425570350204,
68.4641091549303));
#208178=CARTESIAN_POINT('Origin',(-33.5526503323277,-74.999949493375,72.9851176492631));
#208179=CARTESIAN_POINT('',(-32.5154663303127,-85.9425570368316,68.4641091593142));
#208180=CARTESIAN_POINT('',(-32.8170317104293,-85.9425570350204,68.4641091549303));
#208181=CARTESIAN_POINT('',(-33.5526503323277,-85.9425570350204,68.4641091549303));
#208182=CARTESIAN_POINT('Ctrl Pts',(-32.5154663303127,-85.9425570386429,
68.4641091636981));
#208183=CARTESIAN_POINT('Ctrl Pts',(-32.5362001555537,-86.2668363188511,
69.2489917644962));
#208184=CARTESIAN_POINT('Ctrl Pts',(-32.557236083159,-86.5057523881385,
70.0665438105178));
#208185=CARTESIAN_POINT('Ctrl Pts',(-32.5968013922866,-86.7889089507147,
71.6513218766206));
#208186=CARTESIAN_POINT('Ctrl Pts',(-32.615162670662,-86.8502293019532,
72.4111403324576));
#208187=CARTESIAN_POINT('Ctrl Pts',(-32.6432761203485,-86.8322269140453,
73.5541258685461));
#208188=CARTESIAN_POINT('Ctrl Pts',(-32.652734137142,-86.8076621161924,
73.9361595922706));
#208189=CARTESIAN_POINT('Ctrl Pts',(-32.6806312601401,-86.6807210837891,
75.0580105174267));
#208190=CARTESIAN_POINT('Ctrl Pts',(-32.6987270624398,-86.5268492396639,
75.7900945267301));
#208191=CARTESIAN_POINT('Ctrl Pts',(-32.7361038674274,-86.072800945195,
77.2493139389786));
#208192=CARTESIAN_POINT('Ctrl Pts',(-32.7554827092351,-85.7671494755215,
77.970977641766));
#208193=CARTESIAN_POINT('Ctrl Pts',(-32.7933507513484,-85.0286027385363,
79.3241718986652));
#208194=CARTESIAN_POINT('Ctrl Pts',(-32.8116761780355,-84.6012393545235,
79.9545317832694));
#208195=CARTESIAN_POINT('Ctrl Pts',(-32.8433914731719,-83.7772204243217,
80.9489310036303));
#208196=CARTESIAN_POINT('Ctrl Pts',(-32.8565470654291,-83.4108245921608,
81.3349671007405));
#208197=CARTESIAN_POINT('Ctrl Pts',(-32.8881540749963,-82.4647649214919,
82.2060616479441));
#208198=CARTESIAN_POINT('Ctrl Pts',(-32.9063137408051,-81.8622296586511,
82.6628441729054));
#208199=CARTESIAN_POINT('Ctrl Pts',(-32.9386784290198,-80.7376169810788,
83.3572544116666));
#208200=CARTESIAN_POINT('Ctrl Pts',(-32.9526892854524,-80.2340901273826,
83.6202395351201));
#208201=CARTESIAN_POINT('Ctrl Pts',(-32.9760241919647,-79.3619573895282,
83.9987481020109));
#208202=CARTESIAN_POINT('Ctrl Pts',(-32.9853290938375,-79.0030528840064,
84.1342132342873));
#208203=CARTESIAN_POINT('Ctrl Pts',(-33.021684079452,-77.5778963988193,
84.5944182705371));
#208204=CARTESIAN_POINT('Ctrl Pts',(-33.0491279220084,-76.4745400156204,
84.7854247804406));
#208205=CARTESIAN_POINT('Ctrl Pts',(-33.0854694913575,-74.980465276644,
84.8309867661896));
#208206=CARTESIAN_POINT('Ctrl Pts',(-33.0946577552981,-74.5997550705373,
84.8242409289454));
#208207=CARTESIAN_POINT('Ctrl Pts',(-33.1219281605486,-73.4779330231271,
84.7501826497521));
#208208=CARTESIAN_POINT('Ctrl Pts',(-33.1401535735411,-72.7420996480677,
84.6313784846082));
#208209=CARTESIAN_POINT('Ctrl Pts',(-33.1766698348767,-71.2979296906223,
84.2561142083526));
#208210=CARTESIAN_POINT('Ctrl Pts',(-33.1945877072639,-70.5930418352839,
83.9996298991068));
#208211=CARTESIAN_POINT('Ctrl Pts',(-33.2317699618309,-69.2101394892781,
83.3422884929469));
#208212=CARTESIAN_POINT('Ctrl Pts',(-33.2510343398721,-68.5382490198549,
82.9369675079239));
#208213=CARTESIAN_POINT('Ctrl Pts',(-33.2792118147758,-67.6064602754443,
82.2404585606285));
#208214=CARTESIAN_POINT('Ctrl Pts',(-33.288360827012,-67.3127942602629,
81.9980341361255));
#208215=CARTESIAN_POINT('Ctrl Pts',(-33.3155608745428,-66.4796786165661,
81.2399013997123));
#208216=CARTESIAN_POINT('Ctrl Pts',(-33.3337527617114,-65.9767107249673,
80.6869110301534));
#208217=CARTESIAN_POINT('Ctrl Pts',(-33.3701686604761,-65.0806050801455,
79.4924500424553));
#208218=CARTESIAN_POINT('Ctrl Pts',(-33.3880046373794,-64.6897046772445,
78.8534752942746));
#208219=CARTESIAN_POINT('Ctrl Pts',(-33.425040934158,-64.0177777461935,
77.4779861533712));
#208220=CARTESIAN_POINT('Ctrl Pts',(-33.4442621241825,-63.7446205166193,
76.7416494397302));
#208221=CARTESIAN_POINT('Ctrl Pts',(-33.4816087207476,-63.3532977961105,
75.246930029432));
#208222=CARTESIAN_POINT('Ctrl Pts',(-33.4997952030726,-63.2319444456281,
74.4932135551538));
#208223=CARTESIAN_POINT('Ctrl Pts',(-33.5330374949466,-63.145545437588,
73.1283034286607));
#208224=CARTESIAN_POINT('Ctrl Pts',(-33.5478768889659,-63.1537500521688,
72.5214778149435));
#208225=CARTESIAN_POINT('Ctrl Pts',(-33.5716714747802,-63.2426134751784,
71.5395860643369));
#208226=CARTESIAN_POINT('Ctrl Pts',(-33.5807808023606,-63.2950482259868,
71.1630861392373));
#208227=CARTESIAN_POINT('Ctrl Pts',(-33.6078524042025,-63.5033517585942,
70.0591665261869));
#208228=CARTESIAN_POINT('Ctrl Pts',(-33.6259682794434,-63.7097217364428,
69.3431821095985));
#208229=CARTESIAN_POINT('Ctrl Pts',(-33.662268627147,-64.2553500527025,
67.956002829771));
#208230=CARTESIAN_POINT('Ctrl Pts',(-33.6800825137929,-64.5940375698943,
67.2881526140567));
#208231=CARTESIAN_POINT('Ctrl Pts',(-33.7157469632136,-65.3815776410118,
66.042889402939));
#208232=CARTESIAN_POINT('Ctrl Pts',(-33.7335631257147,-65.825410317655,
65.4661129362375));
#208233=CARTESIAN_POINT('Ctrl Pts',(-33.7604159462386,-66.5782982246413,
64.6543886765407));
#208234=CARTESIAN_POINT('Ctrl Pts',(-33.7695669470442,-66.8506431649004,
64.3877888125575));
#208235=CARTESIAN_POINT('Ctrl Pts',(-33.8027431449097,-67.8788358770742,
63.4741163299476));
#208236=CARTESIAN_POINT('Ctrl Pts',(-33.827142276554,-68.702601483181,62.909761785841));
#208237=CARTESIAN_POINT('Ctrl Pts',(-33.8604848528591,-69.9252189508746,
62.2812977763039));
#208238=CARTESIAN_POINT('Ctrl Pts',(-33.8696328599145,-70.2714400569454,
62.1239091781696));
#208239=CARTESIAN_POINT('Ctrl Pts',(-33.9003328092002,-71.4511997282868,
61.6547236603846));
#208240=CARTESIAN_POINT('Ctrl Pts',(-33.9221676751438,-72.312188269407,
61.4201979082925));
#208241=CARTESIAN_POINT('Ctrl Pts',(-33.9531537549127,-73.5680468611588,
61.2260707245608));
#208242=CARTESIAN_POINT('Ctrl Pts',(-33.9623540947932,-73.9474159494766,
61.1860624480864));
#208243=CARTESIAN_POINT('Ctrl Pts',(-33.9965018365887,-75.3555213748371,
61.1060247664143));
#208244=CARTESIAN_POINT('Ctrl Pts',(-34.0218448050146,-76.386231106747,
61.1818348684424));
#208245=CARTESIAN_POINT('Ctrl Pts',(-34.0561679127487,-77.7662903919399,
61.4667855037677));
#208246=CARTESIAN_POINT('Ctrl Pts',(-34.0653565323773,-78.1345758463093,
61.5615133177659));
#208247=CARTESIAN_POINT('Ctrl Pts',(-34.0974356171225,-79.3961546242934,
61.9516218303033));
#208248=CARTESIAN_POINT('Ctrl Pts',(-34.1206717596298,-80.2583404983139,
62.335518771283));
#208249=CARTESIAN_POINT('Ctrl Pts',(-34.1623554485262,-81.723868123819,
63.2098449965164));
#208250=CARTESIAN_POINT('Ctrl Pts',(-34.1808330739508,-82.3421086083129,
63.6652602467367));
#208251=CARTESIAN_POINT('Ctrl Pts',(-34.2089868550122,-83.1944678041097,
64.4309251884236));
#208252=CARTESIAN_POINT('Ctrl Pts',(-34.2183626337148,-83.464557442567,
64.6980946367148));
#208253=CARTESIAN_POINT('Ctrl Pts',(-34.2461425538805,-84.2270339569193,
65.5285647318183));
#208254=CARTESIAN_POINT('Ctrl Pts',(-34.2641935850198,-84.6794134405699,
66.1260180139622));
#208255=CARTESIAN_POINT('Ctrl Pts',(-34.2981159583491,-85.4079851892409,
67.3052775198345));
#208256=CARTESIAN_POINT('Ctrl Pts',(-34.313900770577,-85.6989464536826,
67.874476335635));
#208257=CARTESIAN_POINT('Ctrl Pts',(-34.329622639475,-85.9425570350204,
68.4641091549303));
#208258=CARTESIAN_POINT('Ctrl Pts',(-34.6308727573024,-85.9425570350204,
68.4641091549303));
#208259=CARTESIAN_POINT('Ctrl Pts',(-34.6151647072309,-85.6939094978993,
67.8622849340018));
#208260=CARTESIAN_POINT('Ctrl Pts',(-34.5995663367215,-85.3959511601958,
67.2817919716973));
#208261=CARTESIAN_POINT('Ctrl Pts',(-34.5655837556822,-84.6567913948363,
66.0942658643999));
#208262=CARTESIAN_POINT('Ctrl Pts',(-34.5472770766257,-84.2028031741042,
65.4987349189203));
#208263=CARTESIAN_POINT('Ctrl Pts',(-34.5200847301104,-83.4375414062737,
64.6705548048399));
#208264=CARTESIAN_POINT('Ctrl Pts',(-34.5109387621908,-83.1660354729899,
64.4037452541574));
#208265=CARTESIAN_POINT('Ctrl Pts',(-34.4832349145176,-82.311491216871,
63.6413270748738));
#208266=CARTESIAN_POINT('Ctrl Pts',(-34.4644736135561,-81.6928392277928,
63.1886755374939));
#208267=CARTESIAN_POINT('Ctrl Pts',(-34.4243280928122,-80.2726580978869,
62.3472785062726));
#208268=CARTESIAN_POINT('Ctrl Pts',(-34.4031687356562,-79.4621584529842,
61.9826735535439));
#208269=CARTESIAN_POINT('Ctrl Pts',(-34.3722357835602,-78.2570183909637,
61.5958290693764));
#208270=CARTESIAN_POINT('Ctrl Pts',(-34.3629147924433,-77.8900599117489,
61.497226045264));
#208271=CARTESIAN_POINT('Ctrl Pts',(-34.337168562363,-76.8605944202191,
61.2730627926405));
#208272=CARTESIAN_POINT('Ctrl Pts',(-34.3210092948498,-76.1911532203512,
61.186165893322));
#208273=CARTESIAN_POINT('Ctrl Pts',(-34.2861632365182,-74.7591331587905,
61.1234518467949));
#208274=CARTESIAN_POINT('Ctrl Pts',(-34.267431052308,-73.998867303505,61.1633186959675));
#208275=CARTESIAN_POINT('Ctrl Pts',(-34.2289629584796,-72.4393952168317,
61.396688296194));
#208276=CARTESIAN_POINT('Ctrl Pts',(-34.2093290775955,-71.6458020749369,
61.6010130650712));
#208277=CARTESIAN_POINT('Ctrl Pts',(-34.1709722898193,-70.1796190276928,
62.1452799285413));
#208278=CARTESIAN_POINT('Ctrl Pts',(-34.1525829970362,-69.5057817321438,
62.4707561695213));
#208279=CARTESIAN_POINT('Ctrl Pts',(-34.1159813265182,-68.2174115294735,
63.2509391199804));
#208280=CARTESIAN_POINT('Ctrl Pts',(-34.0974918798712,-67.607089250711,
63.705965598118));
#208281=CARTESIAN_POINT('Ctrl Pts',(-34.0693558525949,-66.7616730010462,
64.4729568089905));
#208282=CARTESIAN_POINT('Ctrl Pts',(-34.0599244964905,-66.4913589481829,
64.7431536343941));
#208283=CARTESIAN_POINT('Ctrl Pts',(-34.0276097484789,-65.6032066065503,
65.7212682687524));
#208284=CARTESIAN_POINT('Ctrl Pts',(-34.0049076937857,-65.0568073308263,
66.4892561927314));
#208285=CARTESIAN_POINT('Ctrl Pts',(-33.9723045829328,-64.424060322569,
67.648783592834));
#208286=CARTESIAN_POINT('Ctrl Pts',(-33.9628625681978,-64.2575194562051,
67.9925139798112));
#208287=CARTESIAN_POINT('Ctrl Pts',(-33.9322576319219,-63.7679958418872,
69.141282453164));
#208288=CARTESIAN_POINT('Ctrl Pts',(-33.9113051902744,-63.5167514112302,
69.9738018899385));
#208289=CARTESIAN_POINT('Ctrl Pts',(-33.8805373415329,-63.2893595333419,
71.1999775036403));
#208290=CARTESIAN_POINT('Ctrl Pts',(-33.871125158333,-63.2380909746136,
71.5768113623866));
#208291=CARTESIAN_POINT('Ctrl Pts',(-33.8344560467218,-63.1085889999484,
73.0602747704319));
#208292=CARTESIAN_POINT('Ctrl Pts',(-33.8077248650607,-63.1678490565414,
74.1731844437304));
#208293=CARTESIAN_POINT('Ctrl Pts',(-33.7708161938028,-63.454971389584,
75.6386756413624));
#208294=CARTESIAN_POINT('Ctrl Pts',(-33.7613251527993,-63.5471871944812,
76.0120184497527));
#208295=CARTESIAN_POINT('Ctrl Pts',(-33.7371337110939,-63.8308436664368,
76.9596755610859));
#208296=CARTESIAN_POINT('Ctrl Pts',(-33.7224675453935,-64.0484396335758,
77.5249930695913));
#208297=CARTESIAN_POINT('Ctrl Pts',(-33.6892264539231,-64.6300104049382,
78.7475375743631));
#208298=CARTESIAN_POINT('Ctrl Pts',(-33.6706288940634,-65.0151972562429,
79.391821109661));
#208299=CARTESIAN_POINT('Ctrl Pts',(-33.636163194024,-65.8508815439249,
80.5292250138947));
#208300=CARTESIAN_POINT('Ctrl Pts',(-33.6201123825181,-66.2872178872439,
81.0292030096662));
#208301=CARTESIAN_POINT('Ctrl Pts',(-33.5854801377261,-67.299745686989,
82.0098175581747));
#208302=CARTESIAN_POINT('Ctrl Pts',(-33.5669967213151,-67.8844164122266,
82.4776171410633));
#208303=CARTESIAN_POINT('Ctrl Pts',(-33.5395581865594,-68.8273062489169,
83.0956700600044));
#208304=CARTESIAN_POINT('Ctrl Pts',(-33.530332062025,-69.1552135967341,
83.2887023103804));
#208305=CARTESIAN_POINT('Ctrl Pts',(-33.5024933750788,-70.1651020687282,
83.8194570842563));
#208306=CARTESIAN_POINT('Ctrl Pts',(-33.4836932287862,-70.8708904003669,
84.1075957813789));
#208307=CARTESIAN_POINT('Ctrl Pts',(-33.447667681666,-72.2815996444594,
84.5305913944526));
#208308=CARTESIAN_POINT('Ctrl Pts',(-33.4305476545864,-72.980848638184,
84.6731725681769));
#208309=CARTESIAN_POINT('Ctrl Pts',(-33.394829336192,-74.4338757657504,
84.8350957688325));
#208310=CARTESIAN_POINT('Ctrl Pts',(-33.3763130781836,-75.1852996757935,
84.8471610513085));
#208311=CARTESIAN_POINT('Ctrl Pts',(-33.3391165478215,-76.7129673545317,
84.7264211013359));
#208312=CARTESIAN_POINT('Ctrl Pts',(-33.3202618390324,-77.4850989654355,
84.5875600682735));
#208313=CARTESIAN_POINT('Ctrl Pts',(-33.2917857623872,-78.6040781646242,
84.2694159652127));
#208314=CARTESIAN_POINT('Ctrl Pts',(-33.2824360030289,-78.9650573931792,
84.1476913381386));
#208315=CARTESIAN_POINT('Ctrl Pts',(-33.254062435625,-80.0476596305296,
83.7234767364529));
#208316=CARTESIAN_POINT('Ctrl Pts',(-33.2353789478727,-80.745720185765,
83.3667290671081));
#208317=CARTESIAN_POINT('Ctrl Pts',(-33.1981196430006,-82.0334725466349,
82.538687540278));
#208318=CARTESIAN_POINT('Ctrl Pts',(-33.1797147752294,-82.6235959920657,
82.0747362894187));
#208319=CARTESIAN_POINT('Ctrl Pts',(-33.1436226430351,-83.7055676849677,
81.0441385737633));
#208320=CARTESIAN_POINT('Ctrl Pts',(-33.1257258711474,-84.1954717050216,
80.4803145839738));
#208321=CARTESIAN_POINT('Ctrl Pts',(-33.0982802356823,-84.8505358131933,
79.5647026712407));
#208322=CARTESIAN_POINT('Ctrl Pts',(-33.0889699029745,-85.0569077586568,
79.2447166974648));
#208323=CARTESIAN_POINT('Ctrl Pts',(-33.0527740201786,-85.802114638911,
77.9569840754069));
#208324=CARTESIAN_POINT('Ctrl Pts',(-33.0264446693192,-86.2195444900787,
76.9255385256059));
#208325=CARTESIAN_POINT('Ctrl Pts',(-32.9901049984065,-86.5801922871778,
75.480014196472));
#208326=CARTESIAN_POINT('Ctrl Pts',(-32.9807775636815,-86.6547558852012,
75.1045569825412));
#208327=CARTESIAN_POINT('Ctrl Pts',(-32.9575906005861,-86.7960016116233,
74.1544662681952));
#208328=CARTESIAN_POINT('Ctrl Pts',(-32.9437648169816,-86.8390166478088,
73.5773273636892));
#208329=CARTESIAN_POINT('Ctrl Pts',(-32.9115049719352,-86.8406196606171,
72.2448080764105));
#208330=CARTESIAN_POINT('Ctrl Pts',(-32.8929994830291,-86.7693936347077,
71.4918945661373));
#208331=CARTESIAN_POINT('Ctrl Pts',(-32.8608659891838,-86.5182184413046,
70.1847600179599));
#208332=CARTESIAN_POINT('Ctrl Pts',(-32.8470745479927,-86.3682277994023,
69.6273248605053));
#208333=CARTESIAN_POINT('Ctrl Pts',(-32.8277666912208,-86.1054186061404,
68.874455678897));
#208334=CARTESIAN_POINT('Ctrl Pts',(-32.8224045352257,-86.0268238377811,
68.6680677523439));
#208335=CARTESIAN_POINT('Ctrl Pts',(-32.8170317104293,-85.9425570350204,
68.4641091549303));
#208336=CARTESIAN_POINT('Origin',(-64.067537349647,-83.3180213346267,69.5522455184007));
#208337=CARTESIAN_POINT('',(-63.567539947994,-92.7913234097594,65.6382900020344));
#208338=CARTESIAN_POINT('',(-64.083662457183,-92.3143114107746,65.8353741883268));
#208339=CARTESIAN_POINT('',(-64.067537349647,-92.3292133594533,65.8292137334027));
#208340=CARTESIAN_POINT('',(-63.5675399484426,-93.4410622313485,71.1605188170969));
#208341=CARTESIAN_POINT('Origin',(-63.5675399484425,-83.3180213346267,69.5522455184007));
#208342=CARTESIAN_POINT('',(-63.5676514812565,-93.4397757524445,71.1683725272602));
#208343=CARTESIAN_POINT('Ctrl Pts',(-63.5675399484426,-93.4410622313485,
71.1605188170969));
#208344=CARTESIAN_POINT('Ctrl Pts',(-63.5675771260472,-93.4406459989832,
71.1631387308018));
#208345=CARTESIAN_POINT('Ctrl Pts',(-63.5676143036518,-93.4402287495399,
71.165758482921));
#208346=CARTESIAN_POINT('Ctrl Pts',(-63.5676514812565,-93.4398104831443,
71.1683780726647));
#208347=CARTESIAN_POINT('',(-64.0597104235077,-74.2995962206461,73.2782678282931));
#208348=CARTESIAN_POINT('Ctrl Pts',(-64.0597104235077,-74.2995962206461,
73.2782678282931));
#208349=CARTESIAN_POINT('Ctrl Pts',(-64.0451218652925,-74.5739578485729,
73.9805348271195));
#208350=CARTESIAN_POINT('Ctrl Pts',(-64.0303356772116,-74.9290239136475,
74.6495330209371));
#208351=CARTESIAN_POINT('Ctrl Pts',(-64.0010809330892,-75.7845158441104,
75.8907572272979));
#208352=CARTESIAN_POINT('Ctrl Pts',(-63.986792125037,-76.2828351876858,
76.4599526620537));
#208353=CARTESIAN_POINT('Ctrl Pts',(-63.9624118992683,-77.2155184999461,
77.3072526411669));
#208354=CARTESIAN_POINT('Ctrl Pts',(-63.9525239575834,-77.616940046916,
77.6190644691922));
#208355=CARTESIAN_POINT('Ctrl Pts',(-63.9304794831546,-78.5750656316906,
78.2509947667963));
#208356=CARTESIAN_POINT('Ctrl Pts',(-63.9183841578929,-79.1431948790861,
78.5508027796503));
#208357=CARTESIAN_POINT('Ctrl Pts',(-63.8936864137597,-80.3346488432265,
79.0391399714275));
#208358=CARTESIAN_POINT('Ctrl Pts',(-63.88113511846,-80.9569483078014,79.225797709248));
#208359=CARTESIAN_POINT('Ctrl Pts',(-63.856575596689,-82.2254688239188,
79.4740442805028));
#208360=CARTESIAN_POINT('Ctrl Pts',(-63.8444614159778,-82.8688166971958,
79.5360061975211));
#208361=CARTESIAN_POINT('Ctrl Pts',(-63.8259893536362,-83.8370504105001,
79.5355609346259));
#208362=CARTESIAN_POINT('Ctrl Pts',(-63.8197844751297,-84.160856180335,
79.5196743975064));
#208363=CARTESIAN_POINT('Ctrl Pts',(-63.8012616880294,-85.1257740309717,
79.4251632815208));
#208364=CARTESIAN_POINT('Ctrl Pts',(-63.7892155220507,-85.7599874091987,
79.3000344343668));
#208365=CARTESIAN_POINT('Ctrl Pts',(-63.7646866488347,-87.0084179082139,
78.9263816821825));
#208366=CARTESIAN_POINT('Ctrl Pts',(-63.7521500622743,-87.6198341036269,
78.6758456951227));
#208367=CARTESIAN_POINT('Ctrl Pts',(-63.7273750610242,-88.7762305561875,
78.0635093820405));
#208368=CARTESIAN_POINT('Ctrl Pts',(-63.7153700975349,-89.319391665153,
77.7044378425474));
#208369=CARTESIAN_POINT('Ctrl Pts',(-63.6918930293161,-90.2944582379416,
76.9159481552165));
#208370=CARTESIAN_POINT('Ctrl Pts',(-63.6804420652402,-90.7303042794259,
76.4937784653884));
#208371=CARTESIAN_POINT('Ctrl Pts',(-63.6520134359374,-91.7183627032395,
75.3484072926959));
#208372=CARTESIAN_POINT('Ctrl Pts',(-63.6354546893578,-92.2159813549411,
74.5842894596791));
#208373=CARTESIAN_POINT('Ctrl Pts',(-63.6099369967653,-92.8025924540037,
73.3532428180121));
#208374=CARTESIAN_POINT('Ctrl Pts',(-63.6013230942664,-92.9716293745234,
72.9269478107908));
#208375=CARTESIAN_POINT('Ctrl Pts',(-63.5843894744831,-93.2500904940269,
72.0578394046302));
#208376=CARTESIAN_POINT('Ctrl Pts',(-63.5760671502839,-93.3597171145667,
71.6159185090164));
#208377=CARTESIAN_POINT('Ctrl Pts',(-63.5676866568907,-93.439665725756,
71.1683542085753));
#208378=CARTESIAN_POINT('',(-64.5675364832709,-89.3666968340079,62.5539864962095));
#208379=CARTESIAN_POINT('Ctrl Pts',(-64.5675364837199,-89.3660909400407,
62.5534304824205));
#208380=CARTESIAN_POINT('Ctrl Pts',(-64.5559053154293,-88.9428563528895,
62.1723173071129));
#208381=CARTESIAN_POINT('Ctrl Pts',(-64.5443683788522,-88.4849430424168,
61.8309194745762));
#208382=CARTESIAN_POINT('Ctrl Pts',(-64.5208921017017,-87.5084101659867,
61.2336544858132));
#208383=CARTESIAN_POINT('Ctrl Pts',(-64.5090141235672,-86.9904281121737,
60.9793895503546));
#208384=CARTESIAN_POINT('Ctrl Pts',(-64.4895980530762,-86.0950101000261,
60.6390797274405));
#208385=CARTESIAN_POINT('Ctrl Pts',(-64.4819115658727,-85.7300076639216,
60.5255089913026));
#208386=CARTESIAN_POINT('Ctrl Pts',(-64.4637503035837,-84.8594397842324,
60.3120024769304));
#208387=CARTESIAN_POINT('Ctrl Pts',(-64.4532397072825,-84.3501047911803,
60.2307861428219));
#208388=CARTESIAN_POINT('Ctrl Pts',(-64.430296409186,-83.2270828504902,
60.1455432302508));
#208389=CARTESIAN_POINT('Ctrl Pts',(-64.4181229662858,-82.6146651702382,
60.1593209414688));
#208390=CARTESIAN_POINT('Ctrl Pts',(-64.393582019433,-81.4022762304732,
60.3048983612713));
#208391=CARTESIAN_POINT('Ctrl Pts',(-64.3811840907539,-80.8041396635978,
60.4364493233302));
#208392=CARTESIAN_POINT('Ctrl Pts',(-64.3626497400445,-79.930308439577,
60.7197347739201));
#208393=CARTESIAN_POINT('Ctrl Pts',(-64.3565059984246,-79.6422585301218,
60.8290195178736));
#208394=CARTESIAN_POINT('Ctrl Pts',(-64.3381789619652,-78.7985985588575,
61.1971140003165));
#208395=CARTESIAN_POINT('Ctrl Pts',(-64.3259769456409,-78.2617699565947,
61.496240439733));
#208396=CARTESIAN_POINT('Ctrl Pts',(-64.3074536245922,-77.5038467125482,
62.0201534087068));
#208397=CARTESIAN_POINT('Ctrl Pts',(-64.3012371111907,-77.2585003728539,
62.208028559282));
#208398=CARTESIAN_POINT('Ctrl Pts',(-64.2828087450528,-76.5537998802924,
62.8043768560138));
#208399=CARTESIAN_POINT('Ctrl Pts',(-64.2707866092118,-76.1242782080949,
63.2460995920489));
#208400=CARTESIAN_POINT('Ctrl Pts',(-64.2461815857642,-75.3497322038532,
64.2130030553009));
#208401=CARTESIAN_POINT('Ctrl Pts',(-64.2336243377818,-75.0072579412108,
64.7383397323998));
#208402=CARTESIAN_POINT('Ctrl Pts',(-64.2090209000687,-74.432058347237,
65.8442881461345));
#208403=CARTESIAN_POINT('Ctrl Pts',(-64.1969313758394,-74.1995909324638,
66.4223889606873));
#208404=CARTESIAN_POINT('Ctrl Pts',(-64.1741708575269,-73.8745334008848,
67.5280676131163));
#208405=CARTESIAN_POINT('Ctrl Pts',(-64.1635849873021,-73.7669170707043,
68.0497086663743));
#208406=CARTESIAN_POINT('Ctrl Pts',(-64.1375350595926,-73.6071678749721,
69.3669952652943));
#208407=CARTESIAN_POINT('Ctrl Pts',(-64.1221954863727,-73.6095231841362,
70.1665095515026));
#208408=CARTESIAN_POINT('Ctrl Pts',(-64.0986553233582,-73.75923543564,71.3543811017856));
#208409=CARTESIAN_POINT('Ctrl Pts',(-64.0907263636134,-73.8341657884656,
71.7497160050924));
#208410=CARTESIAN_POINT('Ctrl Pts',(-64.075116934318,-74.0319672483831,
72.5260089561058));
#208411=CARTESIAN_POINT('Ctrl Pts',(-64.0674339216932,-74.1543432419635,
72.9064724931334));
#208412=CARTESIAN_POINT('Ctrl Pts',(-64.0597104235077,-74.2995962206461,
73.2782678282931));
#208413=CARTESIAN_POINT('',(-64.5675364836265,-91.7950063492917,73.2537214834819));
#208414=CARTESIAN_POINT('Origin',(-64.5675364832709,-83.3180213346267,69.5522455184007));
#208415=CARTESIAN_POINT('Ctrl Pts',(-64.567536483719,-91.7951280360208,
73.2537614015208));
#208416=CARTESIAN_POINT('Ctrl Pts',(-64.5522519075793,-91.9023782991883,
73.0463357077703));
#208417=CARTESIAN_POINT('Ctrl Pts',(-64.5369913991239,-92.0019950641991,
72.8343190083415));
#208418=CARTESIAN_POINT('Ctrl Pts',(-64.5217503919341,-92.0936164747453,
72.6182897831504));
#208419=CARTESIAN_POINT('Ctrl Pts',(-64.5065149014817,-92.1852047213892,
72.4023387533511));
#208420=CARTESIAN_POINT('Ctrl Pts',(-64.4912988981798,-92.2688032584661,
72.182378323606));
#208421=CARTESIAN_POINT('Ctrl Pts',(-64.4760978205663,-92.3440946948215,
71.9590140988965));
#208422=CARTESIAN_POINT('Ctrl Pts',(-64.4609038574466,-92.4193508928554,
71.7357544143678));
#208423=CARTESIAN_POINT('Ctrl Pts',(-64.4457248060474,-92.4863076401705,
71.5090943516248));
#208424=CARTESIAN_POINT('Ctrl Pts',(-64.4305561113083,-92.5446940249905,
71.2796630007527));
#208425=CARTESIAN_POINT('Ctrl Pts',(-64.4153929780723,-92.6030590028226,
71.0503157693915));
#208426=CARTESIAN_POINT('Ctrl Pts',(-64.4002401939035,-92.6528597945351,
70.8181995207348));
#208427=CARTESIAN_POINT('Ctrl Pts',(-64.3850932087498,-92.6938735308666,
70.5839634489218));
#208428=CARTESIAN_POINT('Ctrl Pts',(-64.3699531840988,-92.7348684201324,
70.3498350157449));
#208429=CARTESIAN_POINT('Ctrl Pts',(-64.3548189531346,-92.7670842400402,
70.113588953226));
#208430=CARTESIAN_POINT('Ctrl Pts',(-64.3396859720749,-92.7903475986798,
69.8758907034768));
#208431=CARTESIAN_POINT('Ctrl Pts',(-64.334832339477,-92.797808904247,69.7996532477571));
#208432=CARTESIAN_POINT('Ctrl Pts',(-64.3299788354556,-92.8043496620271,
69.7232665234059));
#208433=CARTESIAN_POINT('Ctrl Pts',(-64.3251253100959,-92.809965244465,
69.6467527948062));
#208434=CARTESIAN_POINT('Ctrl Pts',(-64.3100488689152,-92.8274088533978,
69.4090792187455));
#208435=CARTESIAN_POINT('Ctrl Pts',(-64.2949725167306,-92.8359213053789,
69.1701838191067));
#208436=CARTESIAN_POINT('Ctrl Pts',(-64.2798981906764,-92.8353917560586,
68.9307425222424));
#208437=CARTESIAN_POINT('Ctrl Pts',(-64.2648429722307,-92.8348628779736,
68.6916047315219));
#208438=CARTESIAN_POINT('Ctrl Pts',(-64.2497897747822,-92.8253148473759,
68.4519226836682));
#208439=CARTESIAN_POINT('Ctrl Pts',(-64.2347405281082,-92.8066882622084,
68.2123797226621));
#208440=CARTESIAN_POINT('Ctrl Pts',(-64.2197180065402,-92.7880947549398,
67.9732621524508));
#208441=CARTESIAN_POINT('Ctrl Pts',(-64.2046994217271,-92.7604548736204,
67.7342834363879));
#208442=CARTESIAN_POINT('Ctrl Pts',(-64.1896866931837,-92.723761103761,
67.4961293606001));
#208443=CARTESIAN_POINT('Ctrl Pts',(-64.1746906332506,-92.6871080749401,
67.2582397069306));
#208444=CARTESIAN_POINT('Ctrl Pts',(-64.1597004165899,-92.641421230613,
67.0211731258062));
#208445=CARTESIAN_POINT('Ctrl Pts',(-64.1447179563298,-92.5867450112611,
66.7856152711169));
#208446=CARTESIAN_POINT('Ctrl Pts',(-64.1297582205193,-92.5321517213465,
66.550414695709));
#208447=CARTESIAN_POINT('Ctrl Pts',(-64.1148062175984,-92.4685963074583,
66.3167185364763));
#208448=CARTESIAN_POINT('Ctrl Pts',(-64.099863852003,-92.3961749399324,
66.0852075409147));
#208449=CARTESIAN_POINT('Ctrl Pts',(-64.0944699454781,-92.3700322194679,
66.0016365252302));
#208450=CARTESIAN_POINT('Ctrl Pts',(-64.0890772947653,-92.3427346928514,
65.9183502156652));
#208451=CARTESIAN_POINT('Ctrl Pts',(-64.0836859894461,-92.3142885460423,
65.8353804738359));
#208452=CARTESIAN_POINT('Origin',(-64.067537349647,-83.3180213346267,69.5522455184007));
#208453=CARTESIAN_POINT('',(-63.567539947994,-86.5649230506972,59.8300991896837));
#208454=CARTESIAN_POINT('Ctrl Pts',(-64.0833825702184,-92.3145833582915,
65.8352994300243));
#208455=CARTESIAN_POINT('Ctrl Pts',(-64.0619309619701,-92.2034972449534,
65.5102458841647));
#208456=CARTESIAN_POINT('Ctrl Pts',(-64.0405438036779,-92.0753868183421,
65.1915387606872));
#208457=CARTESIAN_POINT('Ctrl Pts',(-63.9975780848989,-91.7816127980817,
64.5599055048843));
#208458=CARTESIAN_POINT('Ctrl Pts',(-63.9760783705587,-91.6154651381155,
64.2483770552222));
#208459=CARTESIAN_POINT('Ctrl Pts',(-63.911488627533,-91.061916651673,63.3334815420053));
#208460=CARTESIAN_POINT('Ctrl Pts',(-63.8686493908154,-90.6225744631808,
62.7604124769523));
#208461=CARTESIAN_POINT('Ctrl Pts',(-63.803886666834,-89.8898307925944,
61.9886376949778));
#208462=CARTESIAN_POINT('Ctrl Pts',(-63.7825040517021,-89.6341955601574,
61.7463822267544));
#208463=CARTESIAN_POINT('Ctrl Pts',(-63.6782847466946,-88.314927314397,
60.6228146595869));
#208464=CARTESIAN_POINT('Ctrl Pts',(-63.6137547901258,-87.2878515244266,
60.1202593968735));
#208465=CARTESIAN_POINT('Ctrl Pts',(-63.567539947994,-86.5649230506972,
59.8300991896837));
#208466=CARTESIAN_POINT('Origin',(-63.5675399484425,-83.3180213346267,69.5522455184007));
#208467=CARTESIAN_POINT('Origin',(-33.9082782203809,-78.4305456687161,71.5715374392095));
#208468=CARTESIAN_POINT('',(-48.5675364832709,-86.6057727049752,68.1938899513175));
#208469=CARTESIAN_POINT('Origin',(-48.5675364832709,-82.0608411004817,70.0716575959921));
#208470=CARTESIAN_POINT('',(-38.5675364832709,-84.1293203724861,69.217052117043));
#208471=CARTESIAN_POINT('',(-32.6788877561441,-82.6710245849397,69.8195563755257));
#208472=CARTESIAN_POINT('Origin',(-38.5675364832709,-79.5843887679945,71.0948197617183));
#208473=CARTESIAN_POINT('Origin',(-33.5526503323277,-74.999949493375,72.9851176492631));
#208474=CARTESIAN_POINT('Ctrl Pts',(-32.8170317104293,-85.9425570350204,
68.4641091549303));
#208475=CARTESIAN_POINT('Ctrl Pts',(-32.8017220003837,-85.7024411991933,
67.8829349856529));
#208476=CARTESIAN_POINT('Ctrl Pts',(-32.7863496420861,-85.4162708021334,
67.3214853189258));
#208477=CARTESIAN_POINT('Ctrl Pts',(-32.7608347605554,-84.8617909280881,
66.4194041046769));
#208478=CARTESIAN_POINT('Ctrl Pts',(-32.7505255297521,-84.6172361447456,
66.0661359314734));
#208479=CARTESIAN_POINT('Ctrl Pts',(-32.7296708098251,-84.0889065869639,
65.3852438569607));
#208480=CARTESIAN_POINT('Ctrl Pts',(-32.7191392839043,-83.8052559543857,
65.0583404901236));
#208481=CARTESIAN_POINT('Ctrl Pts',(-32.7085755548516,-83.5043603266795,
64.7476924450699));
#208482=CARTESIAN_POINT('Ctrl Pts',(-32.405898694983,-83.5044136926724,
64.7477475410809));
#208483=CARTESIAN_POINT('Ctrl Pts',(-32.4327410348547,-84.2718992350309,
65.5401185566776));
#208484=CARTESIAN_POINT('Ctrl Pts',(-32.4600251083934,-84.9248984032721,
66.4358827107567));
#208485=CARTESIAN_POINT('Ctrl Pts',(-32.4959705871775,-85.6172563043794,
67.7327251559588));
#208486=CARTESIAN_POINT('Ctrl Pts',(-32.5048857483552,-85.7749346554537,
68.0642918789659));
#208487=CARTESIAN_POINT('Ctrl Pts',(-32.5143827756658,-85.9255506318068,
68.4231104132923));
#208488=CARTESIAN_POINT('Ctrl Pts',(-32.5149245145407,-85.9340829810812,
68.4435986323621));
#208489=CARTESIAN_POINT('Ctrl Pts',(-32.5154663303127,-85.9425570386429,
68.4641091636981));
#208490=CARTESIAN_POINT('Origin',(-27.5423496375577,-74.9965420974961,72.9903965241317));
#208491=CARTESIAN_POINT('',(-26.6969350937309,-64.1107405695911,68.3402735649356));
#208492=CARTESIAN_POINT('Ctrl Pts',(-27.3723203523406,-85.9391496445663,
68.4693880429103));
#208493=CARTESIAN_POINT('Ctrl Pts',(-27.3636996501605,-85.8050962805345,
68.1449265076006));
#208494=CARTESIAN_POINT('Ctrl Pts',(-27.3551097818568,-85.656602913772,
67.8264054854172));
#208495=CARTESIAN_POINT('Ctrl Pts',(-27.328549170573,-85.1502905081774,
66.8557319008512));
#208496=CARTESIAN_POINT('Ctrl Pts',(-27.3106304021217,-84.7452160106694,
66.230509408506));
#208497=CARTESIAN_POINT('Ctrl Pts',(-27.2831300851529,-84.0481868827491,
65.3488832284206));
#208498=CARTESIAN_POINT('Ctrl Pts',(-27.2737850478675,-83.7979132654584,
65.0619121673232));
#208499=CARTESIAN_POINT('Ctrl Pts',(-27.2366922027447,-82.7456789989978,
63.9667298171809));
#208500=CARTESIAN_POINT('Ctrl Pts',(-27.2095390063064,-81.8428519134459,
63.2639518915619));
#208501=CARTESIAN_POINT('Ctrl Pts',(-27.172318717458,-80.5203041019529,
62.5111129725245));
#208502=CARTESIAN_POINT('Ctrl Pts',(-27.1629537869745,-80.1778991930004,
62.337656384572));
#208503=CARTESIAN_POINT('Ctrl Pts',(-27.1380744267044,-79.2384073982333,
61.9177563454446));
#208504=CARTESIAN_POINT('Ctrl Pts',(-27.1225970943958,-78.6285864215056,
61.7030125447275));
#208505=CARTESIAN_POINT('Ctrl Pts',(-27.0887288513523,-77.2810534975722,
61.3490746452831));
#208506=CARTESIAN_POINT('Ctrl Pts',(-27.0703984326144,-76.5414194989774,
61.2280527602506));
#208507=CARTESIAN_POINT('Ctrl Pts',(-27.0432293521299,-75.4168264097566,
61.1520074257193));
#208508=CARTESIAN_POINT('Ctrl Pts',(-27.0341195638503,-75.0373145881522,
61.1446195136914));
#208509=CARTESIAN_POINT('Ctrl Pts',(-27.0064444237393,-73.8919104087149,
61.1773740424248));
#208510=CARTESIAN_POINT('Ctrl Pts',(-26.9876862066823,-73.1296576224682,
61.2736375504651));
#208511=CARTESIAN_POINT('Ctrl Pts',(-26.9501334588134,-71.6199605337841,
61.6154471013317));
#208512=CARTESIAN_POINT('Ctrl Pts',(-26.9315328934326,-70.8767923732291,
61.8630228528093));
#208513=CARTESIAN_POINT('Ctrl Pts',(-26.8944219015646,-69.4809320174234,
62.4871971090572));
#208514=CARTESIAN_POINT('Ctrl Pts',(-26.8761197995314,-68.8288518195583,
62.8563569561091));
#208515=CARTESIAN_POINT('Ctrl Pts',(-26.8450525151973,-67.7713377025379,
63.5951446125017));
#208516=CARTESIAN_POINT('Ctrl Pts',(-26.8320439690496,-67.3485935572221,
63.9359379853444));
#208517=CARTESIAN_POINT('Ctrl Pts',(-26.7989683136381,-66.3479106000214,
64.862881895046));
#208518=CARTESIAN_POINT('Ctrl Pts',(-26.7788449346443,-65.8048753902868,
65.482494524121));
#208519=CARTESIAN_POINT('Ctrl Pts',(-26.7490196891172,-65.0898279948038,
66.4934183077934));
#208520=CARTESIAN_POINT('Ctrl Pts',(-26.7390111532609,-64.8673881345169,
66.8459722428458));
#208521=CARTESIAN_POINT('Ctrl Pts',(-26.7187614620685,-64.4589394460568,
67.5760192654688));
#208522=CARTESIAN_POINT('Ctrl Pts',(-26.7085329599487,-64.2735326518323,
67.9531735113464));
#208523=CARTESIAN_POINT('Ctrl Pts',(-26.6982749890421,-64.1085581679634,
68.3393768975646));
#208524=CARTESIAN_POINT('',(-26.3969350937309,-64.1107405695911,68.3402735649356));
#208525=CARTESIAN_POINT('Origin',(-26.5469350937313,-53.5544436394318,63.827825737551));
#208526=CARTESIAN_POINT('Ctrl Pts',(-26.3955978506944,-64.1085838121623,
68.3393168652453));
#208527=CARTESIAN_POINT('Ctrl Pts',(-26.4061671472431,-64.2792160622287,
67.9398748093981));
#208528=CARTESIAN_POINT('Ctrl Pts',(-26.416751543022,-64.4717000818231,
67.5501256478087));
#208529=CARTESIAN_POINT('Ctrl Pts',(-26.4379920407315,-64.8967289793553,
66.7969093671376));
#208530=CARTESIAN_POINT('Ctrl Pts',(-26.4486306576851,-65.1285860795737,
66.4338005620371));
#208531=CARTESIAN_POINT('Ctrl Pts',(-26.4802936890649,-65.8773839632651,
65.391114314244));
#208532=CARTESIAN_POINT('Ctrl Pts',(-26.5008584501326,-66.4485211602495,
64.7539243141916));
#208533=CARTESIAN_POINT('Ctrl Pts',(-26.5358514447633,-67.5086683138891,
63.8013175177357));
#208534=CARTESIAN_POINT('Ctrl Pts',(-26.5500252944045,-67.9613287414215,
63.4503128844906));
#208535=CARTESIAN_POINT('Ctrl Pts',(-26.5826993387652,-69.0658984231094,
62.7153186995669));
#208536=CARTESIAN_POINT('Ctrl Pts',(-26.6009119883849,-69.7327527302829,
62.3582621384974));
#208537=CARTESIAN_POINT('Ctrl Pts',(-26.633610456032,-70.9611934406892,
61.844597299696));
#208538=CARTESIAN_POINT('Ctrl Pts',(-26.6479050391863,-71.5088946671322,
61.6612663526489));
#208539=CARTESIAN_POINT('Ctrl Pts',(-26.6715385593391,-72.4384356559061,
61.423952871691));
#208540=CARTESIAN_POINT('Ctrl Pts',(-26.6808599172737,-72.8134705822262,
61.3473416619736));
#208541=CARTESIAN_POINT('Ctrl Pts',(-26.7171740780291,-74.2854742744447,
61.1202789821206));
#208542=CARTESIAN_POINT('Ctrl Pts',(-26.7445727229865,-75.3976699648159,
61.1057679952971));
#208543=CARTESIAN_POINT('Ctrl Pts',(-26.7809426339764,-76.8730935556046,
61.2940917902757));
#208544=CARTESIAN_POINT('Ctrl Pts',(-26.7901838568864,-77.248031044884,
61.3604443251686));
#208545=CARTESIAN_POINT('Ctrl Pts',(-26.8176517904024,-78.3458986357085,
61.6098232698253));
#208546=CARTESIAN_POINT('Ctrl Pts',(-26.8360248015145,-79.0554657440672,
61.8431652991705));
#208547=CARTESIAN_POINT('Ctrl Pts',(-26.8728273181899,-80.4246542834376,
62.4416171656125));
#208548=CARTESIAN_POINT('Ctrl Pts',(-26.8908787881403,-81.0809298958973,
62.8060274152493));
#208549=CARTESIAN_POINT('Ctrl Pts',(-26.9283004549172,-82.3430537141758,
63.6726441225342));
#208550=CARTESIAN_POINT('Ctrl Pts',(-26.9476729115514,-82.9422950610507,
64.1780896202315));
#208551=CARTESIAN_POINT('Ctrl Pts',(-26.9760265130458,-83.7526521547964,
65.0119463436013));
#208552=CARTESIAN_POINT('Ctrl Pts',(-26.9852398453103,-84.0046681677395,
65.297620929492));
#208553=CARTESIAN_POINT('Ctrl Pts',(-27.0126466015813,-84.7090334743622,
66.1782317810865));
#208554=CARTESIAN_POINT('Ctrl Pts',(-27.0309784936996,-85.1193421781366,
66.804365126236));
#208555=CARTESIAN_POINT('Ctrl Pts',(-27.0583910322376,-85.6407014240736,
67.792404142075));
#208556=CARTESIAN_POINT('Ctrl Pts',(-27.0673916524933,-85.7979333834112,
68.1275894981264));
#208557=CARTESIAN_POINT('Ctrl Pts',(-27.0763524854127,-85.9391496391481,
68.4693880297962));
#208558=CARTESIAN_POINT('Origin',(-49.8209604129909,-85.5885787240481,68.6141501690631));
#208559=CARTESIAN_POINT('',(-47.4206117411878,-74.8936030761356,65.7294283639651));
#208560=CARTESIAN_POINT('',(-47.4206117411893,-80.0485688784053,78.2064603659041));
#208561=CARTESIAN_POINT('Ctrl Pts',(-47.4206117411876,-74.8936030761362,
65.729428363968));
#208562=CARTESIAN_POINT('Ctrl Pts',(-47.4072073505217,-74.5345429245089,
66.753376001073));
#208563=CARTESIAN_POINT('Ctrl Pts',(-47.3965597695574,-74.3257849510905,
67.8789541701247));
#208564=CARTESIAN_POINT('Ctrl Pts',(-47.3802442358666,-74.2939613105297,
70.3818352645528));
#208565=CARTESIAN_POINT('Ctrl Pts',(-47.3761425330335,-74.5723128478446,
71.7610264219768));
#208566=CARTESIAN_POINT('Ctrl Pts',(-47.3761425330335,-75.0680041243238,
72.9607930464209));
#208567=CARTESIAN_POINT('Ctrl Pts',(-47.3761425330335,-75.563695400803,
74.1605596708651));
#208568=CARTESIAN_POINT('Ctrl Pts',(-47.3802442358666,-76.3399893287414,
75.3340227356814));
#208569=CARTESIAN_POINT('Ctrl Pts',(-47.3965597695574,-78.1291388445427,
77.0845570904024));
#208570=CARTESIAN_POINT('Ctrl Pts',(-47.4072073505217,-79.0714850594923,
77.7345491805734));
#208571=CARTESIAN_POINT('Ctrl Pts',(-47.4206117411876,-80.0485688784058,
78.2064603659031));
#208572=CARTESIAN_POINT('',(-40.481003278332,-78.3300079219658,78.9164948483172));
#208573=CARTESIAN_POINT('',(-47.4206117411909,-80.0485688784039,78.2064603659047));
#208574=CARTESIAN_POINT('',(-40.5852420615047,-72.8362530306906,67.7517760446658));
#208575=CARTESIAN_POINT('Ctrl Pts',(-40.4810032783342,-78.3300079219668,
78.9164948483157));
#208576=CARTESIAN_POINT('Ctrl Pts',(-40.5701001577907,-77.3783739218292,
78.4341281348452));
#208577=CARTESIAN_POINT('Ctrl Pts',(-40.6461218070977,-76.4640165146777,
77.7789779463358));
#208578=CARTESIAN_POINT('Ctrl Pts',(-40.7676642501064,-74.7061160640781,
76.0175731138598));
#208579=CARTESIAN_POINT('Ctrl Pts',(-40.8007888323695,-73.936268721286,
74.8355718846972));
#208580=CARTESIAN_POINT('Ctrl Pts',(-40.8007888323695,-73.4396491234305,
73.6335583596984));
#208581=CARTESIAN_POINT('Ctrl Pts',(-40.8007888323695,-72.943029525575,
72.4315448346997));
#208582=CARTESIAN_POINT('Ctrl Pts',(-40.7676642501064,-72.6540848575873,
71.0508555808169));
#208583=CARTESIAN_POINT('Ctrl Pts',(-40.668740252843,-72.6557245993737,
69.0254326994105));
#208584=CARTESIAN_POINT('Ctrl Pts',(-40.6299225890052,-72.7174361037414,
68.3789914813538));
#208585=CARTESIAN_POINT('Ctrl Pts',(-40.5852420615047,-72.8362530306906,
67.7517760446658));
#208586=CARTESIAN_POINT('',(-40.481003278332,-73.1750421196974,66.4394628463787));
#208587=CARTESIAN_POINT('Ctrl Pts',(-40.5852420615047,-72.8362530306906,
67.7517760446658));
#208588=CARTESIAN_POINT('Ctrl Pts',(-40.5532232597647,-72.9213991970445,
67.3023031346757));
#208589=CARTESIAN_POINT('Ctrl Pts',(-40.5182082030456,-73.0357162226427,
66.8626329204887));
#208590=CARTESIAN_POINT('Ctrl Pts',(-40.481003278349,-73.175042119644,66.4394628465471));
#208591=CARTESIAN_POINT('',(-47.4206117411909,-74.8936030761349,65.7294283639646));
#208592=CARTESIAN_POINT('Origin',(-64.4265543961493,-83.3237128444373,69.5530424137804));
#208593=CARTESIAN_POINT('',(-64.5675364832711,-90.9537820568269,64.6166308207583));
#208594=CARTESIAN_POINT('Origin',(-64.5675364832709,-83.3237128444373,69.5530424137804));
#208595=CARTESIAN_POINT('',(-63.7081759237673,-74.9246006814762,73.0230612142441));
#208596=CARTESIAN_POINT('Ctrl Pts',(-64.5675364832717,-90.9537820568266,
64.6166308207584));
#208597=CARTESIAN_POINT('Ctrl Pts',(-64.5460054318702,-90.585927916916,
64.0480492722608));
#208598=CARTESIAN_POINT('Ctrl Pts',(-64.5242151510805,-90.1556468171482,
63.5223301109441));
#208599=CARTESIAN_POINT('Ctrl Pts',(-64.4802433842162,-89.1769113772055,
62.5671481746464));
#208600=CARTESIAN_POINT('Ctrl Pts',(-64.4585326795741,-88.629546564504,
62.142861546234));
#208601=CARTESIAN_POINT('Ctrl Pts',(-64.4216367999337,-87.647267127443,
61.5465778287499));
#208602=CARTESIAN_POINT('Ctrl Pts',(-64.4067804331069,-87.2376250724316,
61.3385500692314));
#208603=CARTESIAN_POINT('Ctrl Pts',(-64.3730365308061,-86.269447621911,
60.9358123869345));
#208604=CARTESIAN_POINT('Ctrl Pts',(-64.3544190590795,-85.7041004997053,
60.7628340472615));
#208605=CARTESIAN_POINT('Ctrl Pts',(-64.3166439831112,-84.5496212266027,
60.529236790111));
#208606=CARTESIAN_POINT('Ctrl Pts',(-64.2975574490637,-83.9632945784081,
60.4688337160353));
#208607=CARTESIAN_POINT('Ctrl Pts',(-64.2597495591603,-82.7850337136813,
60.4621504002003));
#208608=CARTESIAN_POINT('Ctrl Pts',(-64.241099252248,-82.1958827798751,
60.5163118771831));
#208609=CARTESIAN_POINT('Ctrl Pts',(-64.2031978910308,-81.0370119978244,
60.7380099725469));
#208610=CARTESIAN_POINT('Ctrl Pts',(-64.184061183931,-80.47002321394,60.9049062666254));
#208611=CARTESIAN_POINT('Ctrl Pts',(-64.1557944571638,-79.6496879702633,
61.2359124218976));
#208612=CARTESIAN_POINT('Ctrl Pts',(-64.146429116728,-79.3817015131536,
61.3595292794478));
#208613=CARTESIAN_POINT('Ctrl Pts',(-64.1276217352215,-78.8585717954617,
61.632454540492));
#208614=CARTESIAN_POINT('Ctrl Pts',(-64.1181904779767,-78.6037471974636,
61.7816127007718));
#208615=CARTESIAN_POINT('Ctrl Pts',(-64.0897741094685,-77.8630385676629,
62.2650675446127));
#208616=CARTESIAN_POINT('Ctrl Pts',(-64.0707214808186,-77.4019527181837,
62.6344941894086));
#208617=CARTESIAN_POINT('Ctrl Pts',(-64.0332160558767,-76.5577457470272,
63.4575197792184));
#208618=CARTESIAN_POINT('Ctrl Pts',(-64.014559870328,-76.176647047462,63.9091824285621));
#208619=CARTESIAN_POINT('Ctrl Pts',(-63.9767300455895,-75.5073339613555,
64.879936482934));
#208620=CARTESIAN_POINT('Ctrl Pts',(-63.9578042896901,-75.2207011334582,
65.3967325233348));
#208621=CARTESIAN_POINT('Ctrl Pts',(-63.9297910614553,-74.868773083817,
66.2083219024605));
#208622=CARTESIAN_POINT('Ctrl Pts',(-63.9204656552382,-74.7646490456164,
66.4845593731605));
#208623=CARTESIAN_POINT('Ctrl Pts',(-63.8941532883584,-74.5106147379155,
67.2727750530024));
#208624=CARTESIAN_POINT('Ctrl Pts',(-63.8770605769487,-74.3920488100204,
67.7935855420457));
#208625=CARTESIAN_POINT('Ctrl Pts',(-63.8344751232087,-74.2113796600219,
69.1147594772959));
#208626=CARTESIAN_POINT('Ctrl Pts',(-63.80958636877,-74.2081727225401,69.9186094113973));
#208627=CARTESIAN_POINT('Ctrl Pts',(-63.7713711901282,-74.3613121332033,
71.1091500668453));
#208628=CARTESIAN_POINT('Ctrl Pts',(-63.7585739829314,-74.438475725743,
71.5020572684976));
#208629=CARTESIAN_POINT('Ctrl Pts',(-63.7332377069486,-74.6439667049617,
72.2747690093804));
#208630=CARTESIAN_POINT('Ctrl Pts',(-63.7207474086347,-74.772021110162,
72.6537453670004));
#208631=CARTESIAN_POINT('Ctrl Pts',(-63.7081759237673,-74.9246006814762,
73.0230612142441));
#208632=CARTESIAN_POINT('Ctrl Pts',(-63.7081759237673,-74.9246006814762,
73.0230612142441));
#208633=CARTESIAN_POINT('Ctrl Pts',(-63.6875161657485,-75.1753472762659,
73.6299884083669));
#208634=CARTESIAN_POINT('Ctrl Pts',(-63.666633096272,-75.4911431224059,
74.2079528890717));
#208635=CARTESIAN_POINT('Ctrl Pts',(-63.6250338178037,-76.2415525476808,
75.2853977476081));
#208636=CARTESIAN_POINT('Ctrl Pts',(-63.6047129064916,-76.6739032033415,
75.7817602801854));
#208637=CARTESIAN_POINT('Ctrl Pts',(-63.5702347770154,-77.4769637327139,
76.5238902708087));
#208638=CARTESIAN_POINT('Ctrl Pts',(-63.5563499250238,-77.8189848016841,
76.7970165522735));
#208639=CARTESIAN_POINT('Ctrl Pts',(-63.5238782363532,-78.6651834829525,
77.3781042268529));
#208640=CARTESIAN_POINT('Ctrl Pts',(-63.5056266428151,-79.1823446748094,
77.6636872419475));
#208641=CARTESIAN_POINT('Ctrl Pts',(-63.4686546174705,-80.2639002161587,
78.1303410844429));
#208642=CARTESIAN_POINT('Ctrl Pts',(-63.4499671432275,-80.8256634980915,
78.3104533209256));
#208643=CARTESIAN_POINT('Ctrl Pts',(-63.4128436371221,-81.9770369928399,
78.5597118792829));
#208644=CARTESIAN_POINT('Ctrl Pts',(-63.3946215167477,-82.5639656279161,
78.6280860916995));
#208645=CARTESIAN_POINT('Ctrl Pts',(-63.3575823140899,-83.7422255350564,
78.6501758674783));
#208646=CARTESIAN_POINT('Ctrl Pts',(-63.3388446223193,-84.3307600947913,
78.6039452830317));
#208647=CARTESIAN_POINT('Ctrl Pts',(-63.3018702281337,-85.4898411231714,
78.3983799325527));
#208648=CARTESIAN_POINT('Ctrl Pts',(-63.2836465012631,-86.0576752351604,
78.2396736254702));
#208649=CARTESIAN_POINT('Ctrl Pts',(-63.2465196644465,-87.1559936228692,
77.8142404149129));
#208650=CARTESIAN_POINT('Ctrl Pts',(-63.2277373367691,-87.6837798863797,
77.5482653071632));
#208651=CARTESIAN_POINT('Ctrl Pts',(-63.1907483518579,-88.6799825607429,
76.9180689523048));
#208652=CARTESIAN_POINT('Ctrl Pts',(-63.1724068011774,-89.1460822825508,
76.5554173534264));
#208653=CARTESIAN_POINT('Ctrl Pts',(-63.1350988645249,-90.0016677266875,
75.7448462794557));
#208654=CARTESIAN_POINT('Ctrl Pts',(-63.1163171878295,-90.3890983500231,
75.2988106682674));
#208655=CARTESIAN_POINT('Ctrl Pts',(-63.0840698114675,-90.9838957856484,
74.4620982013951));
#208656=CARTESIAN_POINT('Ctrl Pts',(-63.070383528129,-91.2111472462665,
74.0879744284651));
#208657=CARTESIAN_POINT('Ctrl Pts',(-63.03575802426,-91.710095712682,73.1147421819726));
#208658=CARTESIAN_POINT('Ctrl Pts',(-63.0147220449659,-91.9454177103888,
72.499792039988));
#208659=CARTESIAN_POINT('Ctrl Pts',(-62.9836482387311,-92.1959506361543,
71.5473602390956));
#208660=CARTESIAN_POINT('Ctrl Pts',(-62.973330254332,-92.2622035221039,
71.2255528877244));
#208661=CARTESIAN_POINT('Ctrl Pts',(-62.9525789218377,-92.359488578991,
70.576864601696));
#208662=CARTESIAN_POINT('Ctrl Pts',(-62.9421606938526,-92.3905227868185,
70.2504729419997));
#208663=CARTESIAN_POINT('Ctrl Pts',(-62.931689741507,-92.4038646207268,
69.9231225687745));
#208664=CARTESIAN_POINT('',(-63.5151079737573,-74.9246636583587,73.0232136446285));
#208665=CARTESIAN_POINT('Ctrl Pts',(-63.5151079737573,-74.9246636583587,
73.0232136446285));
#208666=CARTESIAN_POINT('Ctrl Pts',(-63.4816571263961,-75.3228894994488,
73.9870618826492));
#208667=CARTESIAN_POINT('Ctrl Pts',(-63.4492397722482,-75.8840734303081,
74.875210590161));
#208668=CARTESIAN_POINT('Ctrl Pts',(-63.3824771659967,-77.266723687465,
76.4040445924905));
#208669=CARTESIAN_POINT('Ctrl Pts',(-63.3506340024212,-78.0719900071899,
77.0392102609248));
#208670=CARTESIAN_POINT('Ctrl Pts',(-63.2990803050339,-79.4817485896302,
77.8096342034867));
#208671=CARTESIAN_POINT('Ctrl Pts',(-63.2798627012716,-80.0239904395514,
78.0409065795314));
#208672=CARTESIAN_POINT('Ctrl Pts',(-63.2420148814413,-81.1452204755426,
78.3953145837462));
#208673=CARTESIAN_POINT('Ctrl Pts',(-63.2234726310312,-81.7215382041962,
78.5176753341718));
#208674=CARTESIAN_POINT('Ctrl Pts',(-63.1860449875657,-82.8898402949109,
78.649388820796));
#208675=CARTESIAN_POINT('Ctrl Pts',(-63.166902594635,-83.4790642592849,
78.6584039746957));
#208676=CARTESIAN_POINT('Ctrl Pts',(-63.1287565369763,-84.654596635391,
78.5621938389019));
#208677=CARTESIAN_POINT('Ctrl Pts',(-63.1099545802623,-85.238071552627,
78.4564857219072));
#208678=CARTESIAN_POINT('Ctrl Pts',(-63.0536399237439,-86.946444137016,
77.9711620727516));
#208679=CARTESIAN_POINT('Ctrl Pts',(-63.0151488836941,-88.0115737252524,
77.427869310999));
#208680=CARTESIAN_POINT('Ctrl Pts',(-62.9590083227095,-89.4046245324071,
76.3320095448116));
#208681=CARTESIAN_POINT('Ctrl Pts',(-62.940472460623,-89.8304017391483,
75.924453235268));
#208682=CARTESIAN_POINT('Ctrl Pts',(-62.9051701193412,-90.5438883000852,
75.0948322057969));
#208683=CARTESIAN_POINT('Ctrl Pts',(-62.8888430717836,-90.841321814152,
74.6841176910583));
#208684=CARTESIAN_POINT('Ctrl Pts',(-62.8485304202398,-91.4962742448335,
73.5995381859555));
#208685=CARTESIAN_POINT('Ctrl Pts',(-62.8249536297514,-91.8062103136783,
72.9014933147706));
#208686=CARTESIAN_POINT('Ctrl Pts',(-62.7883176531253,-92.1355141820709,
71.8077665761614));
#208687=CARTESIAN_POINT('Ctrl Pts',(-62.7760361700276,-92.2223818534238,
71.4359434158888));
#208688=CARTESIAN_POINT('Ctrl Pts',(-62.7516832489389,-92.3488415221792,
70.6837669566824));
#208689=CARTESIAN_POINT('Ctrl Pts',(-62.7396359874419,-92.3883312692993,
70.3041626149918));
#208690=CARTESIAN_POINT('Ctrl Pts',(-62.7276560748581,-92.4038614347471,
69.9232007305413));
#208691=CARTESIAN_POINT('Ctrl Pts',(-64.4174334691588,-91.7227797420337,
66.0829140514177));
#208692=CARTESIAN_POINT('Ctrl Pts',(-64.4028363514007,-91.5481748019053,
65.6603018539285));
#208693=CARTESIAN_POINT('Ctrl Pts',(-64.3882540732041,-91.3419199834527,
65.25146519838));
#208694=CARTESIAN_POINT('Ctrl Pts',(-64.3594594374539,-90.8700985124793,
64.4691034471845));
#208695=CARTESIAN_POINT('Ctrl Pts',(-64.3452859566336,-90.6053241305171,
64.0966231570146));
#208696=CARTESIAN_POINT('Ctrl Pts',(-64.3026020461293,-89.7311263547494,
63.0444153206984));
#208697=CARTESIAN_POINT('Ctrl Pts',(-64.2733419917296,-89.0463574965084,
62.4348613897139));
#208698=CARTESIAN_POINT('Ctrl Pts',(-64.2264360277325,-87.792722421711,
61.6185905971474));
#208699=CARTESIAN_POINT('Ctrl Pts',(-64.2084844170692,-87.2734286352503,
61.3477206114525));
#208700=CARTESIAN_POINT('Ctrl Pts',(-64.1715858830551,-86.1859714638437,
60.9078008299014));
#208701=CARTESIAN_POINT('Ctrl Pts',(-64.1527333829351,-85.620035237133,
60.740571750952));
#208702=CARTESIAN_POINT('Ctrl Pts',(-64.1156388678732,-84.4646051052493,
60.5181037819277));
#208703=CARTESIAN_POINT('Ctrl Pts',(-64.0974824423265,-83.8778773028571,
60.4632320055774));
#208704=CARTESIAN_POINT('Ctrl Pts',(-64.0608178975356,-82.7021876861606,
60.4675969790405));
#208705=CARTESIAN_POINT('Ctrl Pts',(-64.0420536917397,-82.1160066425151,
60.5268008159321));
#208706=CARTESIAN_POINT('Ctrl Pts',(-64.0046823853952,-80.9606971107092,
60.758105192194));
#208707=CARTESIAN_POINT('Ctrl Pts',(-63.9862707238914,-80.3943936764082,
60.9301738347671));
#208708=CARTESIAN_POINT('Ctrl Pts',(-63.9309385982088,-78.7527241764439,
61.6095368533426));
#208709=CARTESIAN_POINT('Ctrl Pts',(-63.8929716043318,-77.7559989133136,
62.2733600379412));
#208710=CARTESIAN_POINT('Ctrl Pts',(-63.8466555962397,-76.7059823331835,
63.3177676912197));
#208711=CARTESIAN_POINT('Ctrl Pts',(-63.837474495331,-76.5072261967547,
63.53569111148));
#208712=CARTESIAN_POINT('Ctrl Pts',(-63.8096802790241,-75.9433278344253,
64.2178338595459));
#208713=CARTESIAN_POINT('Ctrl Pts',(-63.7906821188187,-75.6124659229421,
64.7083354921592));
#208714=CARTESIAN_POINT('Ctrl Pts',(-63.7624535119922,-75.1910566622627,
65.4869514301863));
#208715=CARTESIAN_POINT('Ctrl Pts',(-63.7531028024434,-75.0633219800847,
65.7531559357367));
#208716=CARTESIAN_POINT('Ctrl Pts',(-63.7252693597624,-74.7205177873625,
66.5669362902439));
#208717=CARTESIAN_POINT('Ctrl Pts',(-63.7070369656083,-74.5453935091855,
67.1296354172816));
#208718=CARTESIAN_POINT('Ctrl Pts',(-63.6595559178276,-74.2430232701488,
68.585706164633));
#208719=CARTESIAN_POINT('Ctrl Pts',(-63.6306895989319,-74.1918705736881,
69.4884282042888));
#208720=CARTESIAN_POINT('Ctrl Pts',(-63.587999601034,-74.3156730368305,
70.8368975882274));
#208721=CARTESIAN_POINT('Ctrl Pts',(-63.5736937807602,-74.3912196648846,
71.2861404207558));
#208722=CARTESIAN_POINT('Ctrl Pts',(-63.5444429022993,-74.6089816180539,
72.1696493608413));
#208723=CARTESIAN_POINT('Ctrl Pts',(-63.5297035311655,-74.7509063821301,
72.6026592072826));
#208724=CARTESIAN_POINT('Ctrl Pts',(-63.5151079737573,-74.9246636583587,
73.0232136446285));
#208725=CARTESIAN_POINT('Origin',(-61.5936228798467,-83.3229197588524,69.5524554490053));
#208726=CARTESIAN_POINT('',(-56.4535514884217,-74.9216338018341,73.0234382919193));
#208727=CARTESIAN_POINT('Ctrl Pts',(-57.3654750299524,-91.7241837160232,
66.0814193573838));
#208728=CARTESIAN_POINT('Ctrl Pts',(-57.3511269999552,-91.5507897413691,
65.6617381696345));
#208729=CARTESIAN_POINT('Ctrl Pts',(-57.3367077978504,-91.3461263316519,
65.2554805117783));
#208730=CARTESIAN_POINT('Ctrl Pts',(-57.3043239281533,-90.8258831413671,
64.3908149809122));
#208731=CARTESIAN_POINT('Ctrl Pts',(-57.2864041853605,-90.4970161174915,
63.9427009497785));
#208732=CARTESIAN_POINT('Ctrl Pts',(-57.2496280960837,-89.7290101102497,
63.0750981369921));
#208733=CARTESIAN_POINT('Ctrl Pts',(-57.2305952659493,-89.2845818860741,
62.6638609750959));
#208734=CARTESIAN_POINT('Ctrl Pts',(-57.1954237150673,-88.4107163650698,
62.00361636557));
#208735=CARTESIAN_POINT('Ctrl Pts',(-57.1794898420337,-87.9954101214033,
61.7397429399961));
#208736=CARTESIAN_POINT('Ctrl Pts',(-57.148190326257,-87.1305333422187,
61.2839624331371));
#208737=CARTESIAN_POINT('Ctrl Pts',(-57.1328794922873,-86.6827338480033,
61.0921036329978));
#208738=CARTESIAN_POINT('Ctrl Pts',(-57.1009362166587,-85.7330339675864,
60.7725609603835));
#208739=CARTESIAN_POINT('Ctrl Pts',(-57.0843272617399,-85.2312276240352,
60.6500091943235));
#208740=CARTESIAN_POINT('Ctrl Pts',(-57.0580374834263,-84.4273521006678,
60.5248128591109));
#208741=CARTESIAN_POINT('Ctrl Pts',(-57.0484372892729,-84.1308721435515,
60.493464424947));
#208742=CARTESIAN_POINT('Ctrl Pts',(-57.0160579701305,-83.1170968390338,
60.4364443566522));
#208743=CARTESIAN_POINT('Ctrl Pts',(-56.9934400055393,-82.3985525487146,
60.4810956475757));
#208744=CARTESIAN_POINT('Ctrl Pts',(-56.952011193016,-81.1344679518802,
60.7115248476976));
#208745=CARTESIAN_POINT('Ctrl Pts',(-56.9336416424726,-80.5869234847169,
60.8653549620364));
#208746=CARTESIAN_POINT('Ctrl Pts',(-56.8975866077343,-79.5285546572155,
61.2727739287243));
#208747=CARTESIAN_POINT('Ctrl Pts',(-56.8796783662447,-79.0199942231926,
61.525303890454));
#208748=CARTESIAN_POINT('Ctrl Pts',(-56.844501527484,-78.0889398805368,
62.1016808290221));
#208749=CARTESIAN_POINT('Ctrl Pts',(-56.8273517502541,-77.6647293402901,
62.4184893748666));
#208750=CARTESIAN_POINT('Ctrl Pts',(-56.793853359515,-76.8816904338446,
63.1172871691854));
#208751=CARTESIAN_POINT('Ctrl Pts',(-56.7774870022801,-76.5234790420236,
63.4970084934137));
#208752=CARTESIAN_POINT('Ctrl Pts',(-56.7447381479169,-75.8849848717943,
64.3023881577202));
#208753=CARTESIAN_POINT('Ctrl Pts',(-56.7284256627339,-75.6039484340531,
64.7250797496552));
#208754=CARTESIAN_POINT('Ctrl Pts',(-56.6929753232929,-75.0722101191746,
65.6910700744627));
#208755=CARTESIAN_POINT('Ctrl Pts',(-56.6742621566029,-74.8368586036357,
66.2401636162399));
#208756=CARTESIAN_POINT('Ctrl Pts',(-56.6223104154658,-74.3414220898481,
67.8047577021512));
#208757=CARTESIAN_POINT('Ctrl Pts',(-56.5886870746332,-74.2001051532625,
68.8481768815298));
#208758=CARTESIAN_POINT('Ctrl Pts',(-56.5219062851257,-74.2795067556648,
70.9683983405147));
#208759=CARTESIAN_POINT('Ctrl Pts',(-56.4874132736607,-74.5105716502198,
72.0284893572482));
#208760=CARTESIAN_POINT('Ctrl Pts',(-56.4535514884216,-74.9216338018342,
73.0234382919195));
#208761=CARTESIAN_POINT('Ctrl Pts',(-56.4535514884216,-74.9216338018341,
73.0234382919192));
#208762=CARTESIAN_POINT('Ctrl Pts',(-56.4350025486387,-75.1468070182932,
73.5684552703803));
#208763=CARTESIAN_POINT('Ctrl Pts',(-56.4166167442774,-75.4244814744311,
74.0902687222035));
#208764=CARTESIAN_POINT('Ctrl Pts',(-56.3791654426711,-76.0776033798498,
75.0736682947515));
#208765=CARTESIAN_POINT('Ctrl Pts',(-56.3602283268396,-76.4516830269538,
75.5327997675719));
#208766=CARTESIAN_POINT('Ctrl Pts',(-56.3295967832577,-77.138278850674,
76.2253320098543));
#208767=CARTESIAN_POINT('Ctrl Pts',(-56.317634399164,-77.4259346773961,
76.4808487072807));
#208768=CARTESIAN_POINT('Ctrl Pts',(-56.2894402158142,-78.1341586306357,
77.0337944695028));
#208769=CARTESIAN_POINT('Ctrl Pts',(-56.2731540040184,-78.5655297897047,
77.3152453835778));
#208770=CARTESIAN_POINT('Ctrl Pts',(-56.2191304377677,-80.0620371547784,
78.1198401417049));
#208771=CARTESIAN_POINT('Ctrl Pts',(-56.1828647646033,-81.2054241562849,
78.4715164049074));
#208772=CARTESIAN_POINT('Ctrl Pts',(-56.1075989876639,-83.5623975802335,
78.7162692586896));
#208773=CARTESIAN_POINT('Ctrl Pts',(-56.0713507175757,-84.7533964787986,
78.6070995128668));
#208774=CARTESIAN_POINT('Ctrl Pts',(-56.0244312023155,-86.170417770195,
78.1899669454804));
#208775=CARTESIAN_POINT('Ctrl Pts',(-56.0151271433587,-86.4468088869935,
78.0938936972519));
#208776=CARTESIAN_POINT('Ctrl Pts',(-55.9899598034833,-87.1872017197583,
77.7957799154857));
#208777=CARTESIAN_POINT('Ctrl Pts',(-55.9743076251468,-87.6397370742522,
77.5680755958334));
#208778=CARTESIAN_POINT('Ctrl Pts',(-55.9325391950402,-88.7746966499046,
76.8728703508149));
#208779=CARTESIAN_POINT('Ctrl Pts',(-55.9060931852866,-89.416440799934,
76.3479941666282));
#208780=CARTESIAN_POINT('Ctrl Pts',(-55.8672462315126,-90.2595979929845,
75.4416090357902));
#208781=CARTESIAN_POINT('Ctrl Pts',(-55.8543960475012,-90.5197763975782,
75.1206589210597));
#208782=CARTESIAN_POINT('Ctrl Pts',(-55.8280947721969,-91.0005965893752,
74.4372739798999));
#208783=CARTESIAN_POINT('Ctrl Pts',(-55.8146661895194,-91.2195106834258,
74.0748461106465));
#208784=CARTESIAN_POINT('Ctrl Pts',(-55.8011708396429,-91.4123950525873,
73.6985038205813));
#208785=CARTESIAN_POINT('',(-56.2580209956237,-74.9217169067527,73.0236394350926));
#208786=CARTESIAN_POINT('Ctrl Pts',(-56.2580209956237,-74.9217169067527,
73.0236394350926));
#208787=CARTESIAN_POINT('Ctrl Pts',(-56.2443250754476,-75.0846204163747,
73.4179099304447));
#208788=CARTESIAN_POINT('Ctrl Pts',(-56.2305642181659,-75.2750783558321,
73.8002275282816));
#208789=CARTESIAN_POINT('Ctrl Pts',(-56.2033211069302,-75.7073605527732,
74.5337242263203));
#208790=CARTESIAN_POINT('Ctrl Pts',(-56.1898709563397,-75.9484320247352,
74.8841262966469));
#208791=CARTESIAN_POINT('Ctrl Pts',(-56.1512855608216,-76.707371854651,
75.8368058676944));
#208792=CARTESIAN_POINT('Ctrl Pts',(-56.1256639711523,-77.2807097395701,
76.3898681292522));
#208793=CARTESIAN_POINT('Ctrl Pts',(-56.0833810803596,-78.3407712514973,
77.1736969095166));
#208794=CARTESIAN_POINT('Ctrl Pts',(-56.0667865829977,-78.7893015442435,
77.4487477683126));
#208795=CARTESIAN_POINT('Ctrl Pts',(-56.0320548232101,-79.766401713918,
77.9370958618635));
#208796=CARTESIAN_POINT('Ctrl Pts',(-56.0136903834562,-80.2963550940178,
78.1426188139801));
#208797=CARTESIAN_POINT('Ctrl Pts',(-55.9724037787782,-81.5284216935346,
78.4921548134415));
#208798=CARTESIAN_POINT('Ctrl Pts',(-55.9499103502961,-82.2354030076385,
78.605397131529));
#208799=CARTESIAN_POINT('Ctrl Pts',(-55.903822487772,-83.6793637761405,
78.6649527140371));
#208800=CARTESIAN_POINT('Ctrl Pts',(-55.8800043454388,-84.4113738723253,
78.6067319429833));
#208801=CARTESIAN_POINT('Ctrl Pts',(-55.841858052403,-85.5806198022539,
78.3697661154032));
#208802=CARTESIAN_POINT('Ctrl Pts',(-55.8272928052752,-86.0251498845119,
78.2438378961145));
#208803=CARTESIAN_POINT('Ctrl Pts',(-55.7936110388135,-87.0184892669261,
77.8788240150679));
#208804=CARTESIAN_POINT('Ctrl Pts',(-55.7742461928925,-87.5571384948989,
77.6182491090811));
#208805=CARTESIAN_POINT('Ctrl Pts',(-55.7285410136335,-88.7711700519054,
76.8756090000868));
#208806=CARTESIAN_POINT('Ctrl Pts',(-55.7027970840579,-89.4139326223631,
76.3503647630469));
#208807=CARTESIAN_POINT('Ctrl Pts',(-55.6629912962453,-90.2582430102741,
75.4432276991302));
#208808=CARTESIAN_POINT('Ctrl Pts',(-55.6496589375082,-90.5186999191627,
75.1220745554689));
#208809=CARTESIAN_POINT('Ctrl Pts',(-55.6228882380845,-91.0000718362507,
74.4381366140566));
#208810=CARTESIAN_POINT('Ctrl Pts',(-55.6094895732802,-91.2192478132438,
74.0753471720817));
#208811=CARTESIAN_POINT('Ctrl Pts',(-55.5961206596756,-91.4123422054238,
73.6986069305967));
#208812=CARTESIAN_POINT('Ctrl Pts',(-56.2580209956237,-74.9217169067528,
73.0236394350929));
#208813=CARTESIAN_POINT('Ctrl Pts',(-56.2926073343763,-74.5103362988558,
72.027987245461));
#208814=CARTESIAN_POINT('Ctrl Pts',(-56.3260108520931,-74.2792109946535,
70.9670967281698));
#208815=CARTESIAN_POINT('Ctrl Pts',(-56.3941547954805,-74.2002081594267,
68.8445057035695));
#208816=CARTESIAN_POINT('Ctrl Pts',(-56.4265227223919,-74.3422523522542,
67.799546121765));
#208817=CARTESIAN_POINT('Ctrl Pts',(-56.4789203965196,-74.8393543049745,
66.2337698825305));
#208818=CARTESIAN_POINT('Ctrl Pts',(-56.4979976546502,-75.0751409611987,
65.684805115915));
#208819=CARTESIAN_POINT('Ctrl Pts',(-56.532736048018,-75.6092728256102,
64.7162223172105));
#208820=CARTESIAN_POINT('Ctrl Pts',(-56.5486714524192,-75.8927421873167,
64.291090652088));
#208821=CARTESIAN_POINT('Ctrl Pts',(-56.5812135927908,-76.5323260673472,
63.4874340775086));
#208822=CARTESIAN_POINT('Ctrl Pts',(-56.5977691595269,-76.8882118065885,
63.1110909781267));
#208823=CARTESIAN_POINT('Ctrl Pts',(-56.6308145738522,-77.6680096136265,
62.4159497907822));
#208824=CARTESIAN_POINT('Ctrl Pts',(-56.6471576114214,-78.091689623822,
62.0998077664478));
#208825=CARTESIAN_POINT('Ctrl Pts',(-56.6815228560717,-79.0221041166156,
61.5241819630653));
#208826=CARTESIAN_POINT('Ctrl Pts',(-56.6995260286931,-79.5306161311664,
61.2718387861529));
#208827=CARTESIAN_POINT('Ctrl Pts',(-56.7355244261045,-80.5888864316576,
60.8647416856394));
#208828=CARTESIAN_POINT('Ctrl Pts',(-56.7531344890569,-81.1363977495086,
60.711050953292));
#208829=CARTESIAN_POINT('Ctrl Pts',(-56.79331146269,-82.3999671727881,60.4809925255085));
#208830=CARTESIAN_POINT('Ctrl Pts',(-56.8160841288014,-83.1179966717957,
60.4364660564977));
#208831=CARTESIAN_POINT('Ctrl Pts',(-56.8481932963248,-84.1312184864888,
60.4934959311227));
#208832=CARTESIAN_POINT('Ctrl Pts',(-56.8575101479712,-84.4276804127036,
60.5248533740059));
#208833=CARTESIAN_POINT('Ctrl Pts',(-56.8828739882039,-85.2307648475454,
60.6499554820837));
#208834=CARTESIAN_POINT('Ctrl Pts',(-56.8989249433381,-85.7318063995676,
60.7722709986547));
#208835=CARTESIAN_POINT('Ctrl Pts',(-56.9306247496818,-86.6818969447094,
61.0917059720352));
#208836=CARTESIAN_POINT('Ctrl Pts',(-56.9461926174623,-87.1307544508128,
61.2839971590145));
#208837=CARTESIAN_POINT('Ctrl Pts',(-56.9770159340458,-87.9963784729066,
61.7403358608625));
#208838=CARTESIAN_POINT('Ctrl Pts',(-56.9922216198082,-88.4114715277067,
62.0041393763885));
#208839=CARTESIAN_POINT('Ctrl Pts',(-57.0265860548614,-89.2851086830678,
62.6643175577409));
#208840=CARTESIAN_POINT('Ctrl Pts',(-57.0458060216535,-89.7294982251628,
63.0755829320188));
#208841=CARTESIAN_POINT('Ctrl Pts',(-57.0826057296618,-90.497327911536,
63.9431144140599));
#208842=CARTESIAN_POINT('Ctrl Pts',(-57.0998328662142,-90.8260860586377,
64.3911245878254));
#208843=CARTESIAN_POINT('Ctrl Pts',(-57.1315082096315,-91.3461990421847,
65.2556240251727));
#208844=CARTESIAN_POINT('Ctrl Pts',(-57.1458823024629,-91.5508221368337,
65.6618165793203));
#208845=CARTESIAN_POINT('Ctrl Pts',(-57.1603612091034,-91.7241837160232,
66.0814193573838));
#208846=CARTESIAN_POINT('Origin',(-54.462516693425,-83.3223805071439,69.5544896765311));
#208847=CARTESIAN_POINT('',(-49.1982221066872,-74.9212163133617,73.0257672247191));
#208848=CARTESIAN_POINT('Ctrl Pts',(-50.1089321285242,-91.723644464317,
66.0834535849087));
#208849=CARTESIAN_POINT('Ctrl Pts',(-50.0994336195942,-91.6094380273631,
65.8070293711777));
#208850=CARTESIAN_POINT('Ctrl Pts',(-50.0898876520213,-91.4815881462714,
65.5362396202102));
#208851=CARTESIAN_POINT('Ctrl Pts',(-50.0645523224655,-91.1098859605774,
64.8402840168896));
#208852=CARTESIAN_POINT('Ctrl Pts',(-50.048674965668,-90.8447562790985,
64.4278108302642));
#208853=CARTESIAN_POINT('Ctrl Pts',(-50.0171304476547,-90.2470491828378,
63.6448533458755));
#208854=CARTESIAN_POINT('Ctrl Pts',(-50.0015374739218,-89.9146891796019,
63.276248714982));
#208855=CARTESIAN_POINT('Ctrl Pts',(-49.953823265501,-88.8252169616591,
62.2503795039651));
#208856=CARTESIAN_POINT('Ctrl Pts',(-49.9213980023652,-87.9881259655062,
61.689246247093));
#208857=CARTESIAN_POINT('Ctrl Pts',(-49.851974376817,-85.9975019173158,
60.786550076608));
#208858=CARTESIAN_POINT('Ctrl Pts',(-49.8136784471919,-84.8331530901671,
60.5128852669592));
#208859=CARTESIAN_POINT('Ctrl Pts',(-49.757645753811,-83.0691499064639,
60.4494351506318));
#208860=CARTESIAN_POINT('Ctrl Pts',(-49.7392083102798,-82.4885041654403,
60.4841651943603));
#208861=CARTESIAN_POINT('Ctrl Pts',(-49.7021735698838,-81.3528530603487,
60.6621205125193));
#208862=CARTESIAN_POINT('Ctrl Pts',(-49.6838072996849,-80.8000654677217,
60.8028492188456));
#208863=CARTESIAN_POINT('Ctrl Pts',(-49.6476580471214,-79.7267203638698,
61.1863260386364));
#208864=CARTESIAN_POINT('Ctrl Pts',(-49.6296403007662,-79.2086380689463,
61.4284787014464));
#208865=CARTESIAN_POINT('Ctrl Pts',(-49.5932027578465,-78.2292218191738,
62.0040753822869));
#208866=CARTESIAN_POINT('Ctrl Pts',(-49.5749140332662,-77.7695427425373,
62.335415857715));
#208867=CARTESIAN_POINT('Ctrl Pts',(-49.5342133395524,-76.802880990269,
63.1794756229899));
#208868=CARTESIAN_POINT('Ctrl Pts',(-49.5117063431937,-76.3199648523112,
63.7140396907855));
#208869=CARTESIAN_POINT('Ctrl Pts',(-49.4705593303023,-75.5773352695081,
64.7623231305718));
#208870=CARTESIAN_POINT('Ctrl Pts',(-49.4523615418275,-75.2936591039501,
65.2544623510051));
#208871=CARTESIAN_POINT('Ctrl Pts',(-49.4165436367922,-74.8206065012855,
66.2874806875142));
#208872=CARTESIAN_POINT('Ctrl Pts',(-49.398696196724,-74.6327097900308,
66.8262797100903));
#208873=CARTESIAN_POINT('Ctrl Pts',(-49.3655773179496,-74.3838357000045,
67.8360056556622));
#208874=CARTESIAN_POINT('Ctrl Pts',(-49.3504647070004,-74.306869465203,
68.3009628121704));
#208875=CARTESIAN_POINT('Ctrl Pts',(-49.3198705092816,-74.2235999212939,
69.2619573658559));
#208876=CARTESIAN_POINT('Ctrl Pts',(-49.3045062806606,-74.2211464531685,
69.7567928371245));
#208877=CARTESIAN_POINT('Ctrl Pts',(-49.2588282011871,-74.3320963837926,
71.2039321493425));
#208878=CARTESIAN_POINT('Ctrl Pts',(-49.2281734459348,-74.5556207774409,
72.1409551971163));
#208879=CARTESIAN_POINT('Ctrl Pts',(-49.1982221066872,-74.9212163133618,
73.0257672247193));
#208880=CARTESIAN_POINT('',(-48.6677134573783,-88.926319310838,76.7064654074423));
#208881=CARTESIAN_POINT('Ctrl Pts',(-49.1982221066872,-74.9212163133617,
73.025767224719));
#208882=CARTESIAN_POINT('Ctrl Pts',(-49.1846980474795,-75.086295264689,
73.4252902694153));
#208883=CARTESIAN_POINT('Ctrl Pts',(-49.17120111885,-75.279663006462,73.81252823487));
#208884=CARTESIAN_POINT('Ctrl Pts',(-49.143988944538,-75.7186383315664,
74.554183972483));
#208885=CARTESIAN_POINT('Ctrl Pts',(-49.1303097652266,-75.9633548844277,
74.9078602464795));
#208886=CARTESIAN_POINT('Ctrl Pts',(-49.0903095232135,-76.7519488993082,
75.8907898221601));
#208887=CARTESIAN_POINT('Ctrl Pts',(-49.0648068938641,-77.3580971968119,
76.4643810297756));
#208888=CARTESIAN_POINT('Ctrl Pts',(-49.0230777052332,-78.4328567586469,
77.2332123424207));
#208889=CARTESIAN_POINT('Ctrl Pts',(-49.0074210140729,-78.8545159359737,
77.4859716780431));
#208890=CARTESIAN_POINT('Ctrl Pts',(-48.9742148604392,-79.7976971077219,
77.9521673686708));
#208891=CARTESIAN_POINT('Ctrl Pts',(-48.9568877803953,-80.3228403383812,
78.153742319573));
#208892=CARTESIAN_POINT('Ctrl Pts',(-48.9237288223427,-81.3401391481041,
78.439615953681));
#208893=CARTESIAN_POINT('Ctrl Pts',(-48.908019142487,-81.8272225374683,
78.5344253341945));
#208894=CARTESIAN_POINT('Ctrl Pts',(-48.8736831345182,-82.9016621136855,
78.6536821415626));
#208895=CARTESIAN_POINT('Ctrl Pts',(-48.8554489915002,-83.4886161210103,
78.6618866050423));
#208896=CARTESIAN_POINT('Ctrl Pts',(-48.8094548302731,-84.9538475193705,
78.5405982968361));
#208897=CARTESIAN_POINT('Ctrl Pts',(-48.7811658042173,-85.8200663471706,
78.3393276526718));
#208898=CARTESIAN_POINT('Ctrl Pts',(-48.7396885127796,-87.0478114546505,
77.8574497617519));
#208899=CARTESIAN_POINT('Ctrl Pts',(-48.7261817247739,-87.4402347937579,
77.6699847384728));
#208900=CARTESIAN_POINT('Ctrl Pts',(-48.69851862242,-88.2047631247771,77.2349803582429));
#208901=CARTESIAN_POINT('Ctrl Pts',(-48.6843884534109,-88.5750682105596,
76.9866399293904));
#208902=CARTESIAN_POINT('Ctrl Pts',(-48.6701794005809,-88.9256751617519,
76.7121720277593));
#208903=CARTESIAN_POINT('',(-48.4675099033474,-88.9256126608575,76.7079526484011));
#208904=CARTESIAN_POINT('Ctrl Pts',(-48.6675364832709,-88.925670370627,
76.7064311666085));
#208905=CARTESIAN_POINT('Ctrl Pts',(-48.6008609566297,-88.9257458498605,
76.7121166899682));
#208906=CARTESIAN_POINT('Ctrl Pts',(-48.5341854299886,-88.9257458498605,
76.7121166899682));
#208907=CARTESIAN_POINT('Ctrl Pts',(-48.4675099033474,-88.9256126608575,
76.7079526484011));
#208908=CARTESIAN_POINT('',(-49.0012377727688,-74.9211148625051,73.0255216838241));
#208909=CARTESIAN_POINT('Ctrl Pts',(-49.0012377727688,-74.9211148625051,
73.0255216838241));
#208910=CARTESIAN_POINT('Ctrl Pts',(-48.9869942993802,-75.089699356929,
73.4335626117807));
#208911=CARTESIAN_POINT('Ctrl Pts',(-48.9727665448755,-75.2877888236457,
73.8287836060104));
#208912=CARTESIAN_POINT('Ctrl Pts',(-48.9446794933811,-75.7378818958822,
74.5840306230201));
#208913=CARTESIAN_POINT('Ctrl Pts',(-48.9308529409634,-75.988815789032,
74.943342021598));
#208914=CARTESIAN_POINT('Ctrl Pts',(-48.8896864538057,-76.8041834998098,
75.9478730052195));
#208915=CARTESIAN_POINT('Ctrl Pts',(-48.8618295254185,-77.4349142322651,
76.5330266535213));
#208916=CARTESIAN_POINT('Ctrl Pts',(-48.8153368443144,-78.6323171351225,
77.3643920918584));
#208917=CARTESIAN_POINT('Ctrl Pts',(-48.7964053555968,-79.1593375887011,
77.6575966005903));
#208918=CARTESIAN_POINT('Ctrl Pts',(-48.7622406355031,-80.1315986182241,
78.0784464647309));
#208919=CARTESIAN_POINT('Ctrl Pts',(-48.7474157728212,-80.5648917952641,
78.2283117360319));
#208920=CARTESIAN_POINT('Ctrl Pts',(-48.7035598203036,-81.8874291244707,
78.5765719982373));
#208921=CARTESIAN_POINT('Ctrl Pts',(-48.6750545183272,-82.7970469727182,
78.6748551441189));
#208922=CARTESIAN_POINT('Ctrl Pts',(-48.6306159838848,-84.1726571729396,
78.6167461339182));
#208923=CARTESIAN_POINT('Ctrl Pts',(-48.6156168883726,-84.637081559956,
78.5611000819166));
#208924=CARTESIAN_POINT('Ctrl Pts',(-48.5787691667439,-85.7727895048833,
78.3352724470895));
#208925=CARTESIAN_POINT('Ctrl Pts',(-48.5570481635015,-86.4328395490297,
78.1237188431876));
#208926=CARTESIAN_POINT('Ctrl Pts',(-48.5231754596634,-87.3916298392153,
77.6908842886861));
#208927=CARTESIAN_POINT('Ctrl Pts',(-48.5115549194922,-87.7115877986523,
77.5228376567632));
#208928=CARTESIAN_POINT('Ctrl Pts',(-48.4883063582056,-88.3347227938847,
77.1466111270654));
#208929=CARTESIAN_POINT('Ctrl Pts',(-48.4767027792111,-88.6369798719034,
76.93818233476));
#208930=CARTESIAN_POINT('Ctrl Pts',(-48.4651187514169,-88.9258151777998,
76.7120624158844));
#208931=CARTESIAN_POINT('Ctrl Pts',(-49.0012377727688,-74.9211148625051,
73.0255216838243));
#208932=CARTESIAN_POINT('Ctrl Pts',(-49.0300579383319,-74.5800019255054,
72.1998939187861));
#208933=CARTESIAN_POINT('Ctrl Pts',(-49.0579275328701,-74.3624530212605,
71.3284842431545));
#208934=CARTESIAN_POINT('Ctrl Pts',(-49.1024052105896,-74.2271701161775,
69.9454212245552));
#208935=CARTESIAN_POINT('Ctrl Pts',(-49.1184482023418,-74.2193918386184,
69.4483149280677));
#208936=CARTESIAN_POINT('Ctrl Pts',(-49.148701269016,-74.2819747701981,
68.5044907200461));
#208937=CARTESIAN_POINT('Ctrl Pts',(-49.1628092336948,-74.344955084967,
68.0587394864049));
#208938=CARTESIAN_POINT('Ctrl Pts',(-49.1997883134222,-74.5938130420238,
66.916478032258));
#208939=CARTESIAN_POINT('Ctrl Pts',(-49.2228683860683,-74.8298972452911,
66.2341433446612));
#208940=CARTESIAN_POINT('Ctrl Pts',(-49.2639268800242,-75.3906777671344,
65.0782215789127));
#208941=CARTESIAN_POINT('Ctrl Pts',(-49.2815569067501,-75.6843228254867,
64.5937476630907));
#208942=CARTESIAN_POINT('Ctrl Pts',(-49.3203981633498,-76.4170658727824,
63.6057160228744));
#208943=CARTESIAN_POINT('Ctrl Pts',(-49.3416920089049,-76.8704570668344,
63.1167925672631));
#208944=CARTESIAN_POINT('Ctrl Pts',(-49.3806443144535,-77.7958426459659,
62.3157496485224));
#208945=CARTESIAN_POINT('Ctrl Pts',(-49.3980155450531,-78.2514659505196,
61.9895834962571));
#208946=CARTESIAN_POINT('Ctrl Pts',(-49.4335438607192,-79.2258756161993,
61.419846811469));
#208947=CARTESIAN_POINT('Ctrl Pts',(-49.4516749204165,-79.7435212891671,
61.1791973110947));
#208948=CARTESIAN_POINT('Ctrl Pts',(-49.4879074009792,-80.8161365724487,
60.7982663185702));
#208949=CARTESIAN_POINT('Ctrl Pts',(-49.5056126479794,-81.368685559789,
60.6586599453322));
#208950=CARTESIAN_POINT('Ctrl Pts',(-49.5415855326542,-82.5035879300481,
60.4828280189462));
#208951=CARTESIAN_POINT('Ctrl Pts',(-49.5599179145507,-83.0837029875439,
60.4490798928174));
#208952=CARTESIAN_POINT('Ctrl Pts',(-49.6160241474124,-84.8471661869708,
60.5152178061111));
#208953=CARTESIAN_POINT('Ctrl Pts',(-49.6522879316194,-86.0112414920116,
60.7907328663199));
#208954=CARTESIAN_POINT('Ctrl Pts',(-49.7214250071374,-87.9922109798468,
61.6928355956797));
#208955=CARTESIAN_POINT('Ctrl Pts',(-49.7518751356753,-88.8214775823457,
62.2488159886867));
#208956=CARTESIAN_POINT('Ctrl Pts',(-49.7991169299812,-89.9108243913346,
63.2716368906033));
#208957=CARTESIAN_POINT('Ctrl Pts',(-49.815167059316,-90.2480015101607,
63.6453776917895));
#208958=CARTESIAN_POINT('Ctrl Pts',(-49.8463623528132,-90.8484992053569,
64.4334279320365));
#208959=CARTESIAN_POINT('Ctrl Pts',(-49.8614853611635,-91.1126658038604,
64.8450102511));
#208960=CARTESIAN_POINT('Ctrl Pts',(-49.886164854335,-91.4827887918636,
65.5387831313055));
#208961=CARTESIAN_POINT('Ctrl Pts',(-49.8955642184998,-91.6099752738436,
65.8083297176374));
#208962=CARTESIAN_POINT('Ctrl Pts',(-49.9050113929448,-91.723644464317,
66.0834535849087));
#208963=CARTESIAN_POINT('Ctrl Pts',(-48.6992141518181,-88.6234275459005,
76.9087096781305));
#208964=CARTESIAN_POINT('Ctrl Pts',(-48.6491771284881,-89.9491017707071,
76.0595009463133));
#208965=CARTESIAN_POINT('Ctrl Pts',(-48.5491030818342,-92.1856846035653,
73.6287810246092));
#208966=CARTESIAN_POINT('Ctrl Pts',(-48.3989920118381,-93.3103166936467,
68.6586256876712));
#208967=CARTESIAN_POINT('Ctrl Pts',(-48.2488809418481,-91.7677199889504,
63.6554187246849));
#208968=CARTESIAN_POINT('Ctrl Pts',(-48.1488068951881,-89.1478110606889,
61.2125219408772));
#208969=CARTESIAN_POINT('Ctrl Pts',(-48.0987698718642,-87.5969606882947,
60.3923995585769));
#208970=CARTESIAN_POINT('Ctrl Pts',(-48.6180189895515,-88.6234275459005,
76.9087096781305));
#208971=CARTESIAN_POINT('Ctrl Pts',(-48.5679819662217,-89.9491017707071,
76.0595009463133));
#208972=CARTESIAN_POINT('Ctrl Pts',(-48.4679079195627,-92.1856846035653,
73.6287810246092));
#208973=CARTESIAN_POINT('Ctrl Pts',(-48.3177968495717,-93.3103166936467,
68.6586256876712));
#208974=CARTESIAN_POINT('Ctrl Pts',(-48.1676857795814,-91.7677199889504,
63.6554187246849));
#208975=CARTESIAN_POINT('Ctrl Pts',(-48.0676117329217,-89.1478110606889,
61.2125219408772));
#208976=CARTESIAN_POINT('Ctrl Pts',(-48.0175747095927,-87.5969606882947,
60.3923995585769));
#208977=CARTESIAN_POINT('Ctrl Pts',(-48.536823827284,-88.6234275459005,
76.9087096781305));
#208978=CARTESIAN_POINT('Ctrl Pts',(-48.4867868039552,-89.9491017707071,
76.0595009463133));
#208979=CARTESIAN_POINT('Ctrl Pts',(-48.3867127572953,-92.1856846035653,
73.6287810246092));
#208980=CARTESIAN_POINT('Ctrl Pts',(-48.2366016873052,-93.3103166936467,
68.6586256876712));
#208981=CARTESIAN_POINT('Ctrl Pts',(-48.086490617314,-91.7677199889504,
63.6554187246849));
#208982=CARTESIAN_POINT('Ctrl Pts',(-47.9864165706552,-89.1478110606889,
61.2125219408772));
#208983=CARTESIAN_POINT('Ctrl Pts',(-47.9363795473253,-87.5969606882947,
60.3923995585769));
#208984=CARTESIAN_POINT('Ctrl Pts',(-48.4556286650124,-88.6234275459005,
76.9087096781305));
#208985=CARTESIAN_POINT('Ctrl Pts',(-48.4055916416887,-89.9491017707071,
76.0595009463133));
#208986=CARTESIAN_POINT('Ctrl Pts',(-48.3055175950287,-92.1856846035653,
73.6287810246092));
#208987=CARTESIAN_POINT('Ctrl Pts',(-48.1554065250387,-93.3103166936467,
68.6586256876712));
#208988=CARTESIAN_POINT('Ctrl Pts',(-48.0052954550424,-91.7677199889504,
63.6554187246849));
#208989=CARTESIAN_POINT('Ctrl Pts',(-47.9052214083887,-89.1478110606889,
61.2125219408772));
#208990=CARTESIAN_POINT('Ctrl Pts',(-47.8551843850587,-87.5969606882947,
60.3923995585769));
#208991=CARTESIAN_POINT('',(-48.0901869004046,-87.9505400884526,60.5887241650105));
#208992=CARTESIAN_POINT('Ctrl Pts',(-48.6675364832709,-88.9255866918527,
76.7063115883213));
#208993=CARTESIAN_POINT('Ctrl Pts',(-48.6312818813982,-89.8622753124554,
76.0508334282851));
#208994=CARTESIAN_POINT('Ctrl Pts',(-48.5950272795265,-90.6834819943738,
75.2089926204495));
#208995=CARTESIAN_POINT('Ctrl Pts',(-48.5587726776542,-91.3266685573513,
74.2361378408557));
#208996=CARTESIAN_POINT('Ctrl Pts',(-48.5488391350575,-91.5028978024944,
73.9695814895414));
#208997=CARTESIAN_POINT('Ctrl Pts',(-48.5389055924608,-91.6657627683633,
73.6931898159694));
#208998=CARTESIAN_POINT('Ctrl Pts',(-48.5289720498641,-91.813977577031,
73.4081017822123));
#208999=CARTESIAN_POINT('Ctrl Pts',(-48.4789350265345,-92.5605619669258,
71.9720625789632));
#209000=CARTESIAN_POINT('Ctrl Pts',(-48.4288980032028,-92.9354393302862,
70.3153441333172));
#209001=CARTESIAN_POINT('Ctrl Pts',(-48.378860979872,-92.8657785611838,
68.6531170833298));
#209002=CARTESIAN_POINT('Ctrl Pts',(-48.3288239565412,-92.7961177920813,
66.9908900333425));
#209003=CARTESIAN_POINT('Ctrl Pts',(-48.2787869332112,-92.2819188905158,
65.3231543790137));
#209004=CARTESIAN_POINT('Ctrl Pts',(-48.2287499098812,-91.3698422076677,
63.8785623558974));
#209005=CARTESIAN_POINT('Ctrl Pts',(-48.1929768543094,-90.7177696483925,
62.8457776840203));
#209006=CARTESIAN_POINT('Ctrl Pts',(-48.1572037987375,-89.8623194913236,
61.9270378615952));
#209007=CARTESIAN_POINT('Ctrl Pts',(-48.1214304257687,-88.8608821258745,
61.1874783364655));
#209008=CARTESIAN_POINT('Ctrl Pts',(-48.1110157930562,-88.5693356073277,
60.9721718058239));
#209009=CARTESIAN_POINT('Ctrl Pts',(-48.1006011334425,-88.2654160984107,
60.7720515629503));
#209010=CARTESIAN_POINT('Ctrl Pts',(-48.090186439096,-87.9505401496632,
60.5887240860841));
#209011=CARTESIAN_POINT('',(-47.8901874902887,-87.9505401262583,60.5887240720849));
#209012=CARTESIAN_POINT('',(-48.0901862140809,-87.9505401261674,60.5887240724043));
#209013=CARTESIAN_POINT('Ctrl Pts',(-48.4675451203219,-88.9253730646099,
76.7064610762623));
#209014=CARTESIAN_POINT('Ctrl Pts',(-48.4374727537661,-89.7023621699198,
76.1627715126034));
#209015=CARTESIAN_POINT('Ctrl Pts',(-48.4076478871442,-90.393251570204,
75.4956452737586));
#209016=CARTESIAN_POINT('Ctrl Pts',(-48.3478038746687,-91.5558518713347,
73.9693330989564));
#209017=CARTESIAN_POINT('Ctrl Pts',(-48.3182577310618,-92.0138637347129,
73.1182182398338));
#209018=CARTESIAN_POINT('Ctrl Pts',(-48.2515859642631,-92.7341784031747,
71.0669096930217));
#209019=CARTESIAN_POINT('Ctrl Pts',(-48.2150542464285,-92.9161625724017,
69.8554430328749));
#209020=CARTESIAN_POINT('Ctrl Pts',(-48.1419859937645,-92.8144445035439,
67.4281199427107));
#209021=CARTESIAN_POINT('Ctrl Pts',(-48.1054696631337,-92.5225233986339,
66.2128718196244));
#209022=CARTESIAN_POINT('Ctrl Pts',(-48.0390051710523,-91.6008694441996,
64.1561131800471));
#209023=CARTESIAN_POINT('Ctrl Pts',(-48.0094233078613,-91.040000796683,
63.3004156653558));
#209024=CARTESIAN_POINT('Ctrl Pts',(-47.9496630882316,-89.6603235361633,
61.7718652461384));
#209025=CARTESIAN_POINT('Ctrl Pts',(-47.9198152757014,-88.8463284293892,
61.1102710786235));
#209026=CARTESIAN_POINT('Ctrl Pts',(-47.8901874908167,-87.9505401260834,
60.5887240723554));
#209027=CARTESIAN_POINT('Ctrl Pts',(-63.7104920345709,-92.1934303316092,
74.8099293892526));
#209028=CARTESIAN_POINT('Ctrl Pts',(-63.6718652093945,-92.8968687267479,
73.6224666938168));
#209029=CARTESIAN_POINT('Ctrl Pts',(-63.5946115590417,-93.8203341640412,
70.961991106913));
#209030=CARTESIAN_POINT('Ctrl Pts',(-63.4787310835129,-93.5364438833945,
66.7467220222676));
#209031=CARTESIAN_POINT('Ctrl Pts',(-63.3628506079829,-91.6282348476794,
62.977524645695));
#209032=CARTESIAN_POINT('Ctrl Pts',(-63.2469701324539,-88.3991168492557,
60.25336151795));
#209033=CARTESIAN_POINT('Ctrl Pts',(-63.1310896569249,-84.3623407018535,
59.0072882090149));
#209034=CARTESIAN_POINT('Ctrl Pts',(-63.0152091813959,-80.1595688410345,
59.4373596262817));
#209035=CARTESIAN_POINT('Ctrl Pts',(-62.8993287058659,-76.4588404646688,
61.4752179418164));
#209036=CARTESIAN_POINT('Ctrl Pts',(-62.7834482303369,-73.8483960341625,
64.7969396843518));
#209037=CARTESIAN_POINT('Ctrl Pts',(-62.6675677548079,-72.7431720463215,
68.8745291515197));
#209038=CARTESIAN_POINT('Ctrl Pts',(-62.5516872792779,-73.3188466353806,
73.0598433065361));
#209039=CARTESIAN_POINT('Ctrl Pts',(-62.4358068037489,-75.4839148855997,
76.6876160812524));
#209040=CARTESIAN_POINT('Ctrl Pts',(-62.3199263282199,-78.8942338216446,
79.1812039750164));
#209041=CARTESIAN_POINT('Ctrl Pts',(-62.2040458526899,-83.0077247744123,
80.1442449974989));
#209042=CARTESIAN_POINT('Ctrl Pts',(-62.0881653771609,-87.1705381364528,
79.4236613850277));
#209043=CARTESIAN_POINT('Ctrl Pts',(-61.9722849016309,-90.7209843805715,
77.1339916933007));
#209044=CARTESIAN_POINT('Ctrl Pts',(-61.8564044261019,-93.0947112545776,
73.6391846088869));
#209045=CARTESIAN_POINT('Ctrl Pts',(-61.7405239505729,-93.9144089739031,
69.4947484013197));
#209046=CARTESIAN_POINT('Ctrl Pts',(-61.6246434750429,-93.0497845493678,
65.3594515033776));
#209047=CARTESIAN_POINT('Ctrl Pts',(-61.5087629995139,-90.638272181575,
61.8906096318565));
#209048=CARTESIAN_POINT('Ctrl Pts',(-61.3928825239839,-87.0631877532088,
59.6396038211845));
#209049=CARTESIAN_POINT('Ctrl Pts',(-61.2770020484549,-82.8927998170843,
58.9642370379884));
#209050=CARTESIAN_POINT('Ctrl Pts',(-61.1611215729249,-78.790001897706,
59.9718605105236));
#209051=CARTESIAN_POINT('Ctrl Pts',(-61.0452410973959,-75.4069439184922,
62.5023099842148));
#209052=CARTESIAN_POINT('Ctrl Pts',(-60.9293606218659,-73.2813713510347,
66.1533642278691));
#209053=CARTESIAN_POINT('Ctrl Pts',(-60.8134801463369,-72.7511492362934,
70.3446790977719));
#209054=CARTESIAN_POINT('Ctrl Pts',(-60.6975996708069,-73.9005576968343,
74.4100346812925));
#209055=CARTESIAN_POINT('Ctrl Pts',(-60.5817191952779,-76.5468954019475,
77.7032326073398));
#209056=CARTESIAN_POINT('Ctrl Pts',(-60.4658387197479,-80.2695203981129,
79.7008108830386));
#209057=CARTESIAN_POINT('Ctrl Pts',(-60.3499582442189,-84.4767121926759,
80.0852494781352));
#209058=CARTESIAN_POINT('Ctrl Pts',(-60.2340777686899,-88.4997271963806,
78.7954409227263));
#209059=CARTESIAN_POINT('Ctrl Pts',(-60.1181972931599,-91.6990971784923,
76.0364034914596));
#209060=CARTESIAN_POINT('Ctrl Pts',(-60.0023168176309,-93.566274330974,
72.2466930393405));
#209061=CARTESIAN_POINT('Ctrl Pts',(-59.8864363421009,-93.8044662060933,
68.0286934589439));
#209062=CARTESIAN_POINT('Ctrl Pts',(-59.7705558665719,-92.375811613486,
64.0528662639258));
#209063=CARTESIAN_POINT('Ctrl Pts',(-59.6546753910419,-89.5073987503684,
60.9511790655875));
#209064=CARTESIAN_POINT('Ctrl Pts',(-59.5387949155129,-85.6551689684265,
59.2166527507833));
#209065=CARTESIAN_POINT('Ctrl Pts',(-59.4229144399829,-81.4314437630425,
59.1249945869912));
#209066=CARTESIAN_POINT('Ctrl Pts',(-59.3070339644539,-77.5075947501924,
60.6907738670809));
#209067=CARTESIAN_POINT('Ctrl Pts',(-59.1911534889249,-74.5073274799646,
63.6651060840353));
#209068=CARTESIAN_POINT('Ctrl Pts',(-59.0752730133949,-72.9075418896531,
67.575213741715));
#209069=CARTESIAN_POINT('Ctrl Pts',(-58.9593925378659,-72.9625278737866,
71.7995755125808));
#209070=CARTESIAN_POINT('Ctrl Pts',(-58.8435120623359,-74.6635452735643,
75.6667185969865));
#209071=CARTESIAN_POINT('Ctrl Pts',(-58.7276315868069,-77.740213146816,
78.5619509930675));
#209072=CARTESIAN_POINT('Ctrl Pts',(-58.6117511112779,-81.7034874905648,
80.0250683177526));
#209073=CARTESIAN_POINT('Ctrl Pts',(-58.4958706357479,-85.923396000422,
79.8235044369147));
#209074=CARTESIAN_POINT('Ctrl Pts',(-58.3799901602189,-89.7291737336331,
77.9892984302229));
#209075=CARTESIAN_POINT('Ctrl Pts',(-58.2641096846899,-92.5158828633906,
74.8140018998643));
#209076=CARTESIAN_POINT('Ctrl Pts',(-58.1482292091609,-93.8405690494499,
70.8023361189094));
#209077=CARTESIAN_POINT('Ctrl Pts',(-58.0323487336309,-93.4926701311195,
66.5919653309314));
#209078=CARTESIAN_POINT('Ctrl Pts',(-57.9164682581019,-91.5274855058807,
62.8521384340946));
#209079=CARTESIAN_POINT('Ctrl Pts',(-57.8005877825729,-88.2573861527595,
60.1773102058844));
#209080=CARTESIAN_POINT('Ctrl Pts',(-57.6847073070439,-84.2021624890806,
58.992651239347));
#209081=CARTESIAN_POINT('Ctrl Pts',(-57.5688268315149,-80.0064023920941,
59.4864660203554));
#209082=CARTESIAN_POINT('Ctrl Pts',(-57.4529463559859,-76.3370323543386,
61.5802614638165));
#209083=CARTESIAN_POINT('Ctrl Pts',(-57.3370658804569,-73.7773078604179,
64.9412235766449));
#209084=CARTESIAN_POINT('Ctrl Pts',(-57.2211854049279,-72.7341034791027,
69.0351190986164));
#209085=CARTESIAN_POINT('Ctrl Pts',(-57.1053049293989,-73.3732391374036,
73.2112130953808));
#209086=CARTESIAN_POINT('Ctrl Pts',(-56.9894244538699,-75.5931226397066,
76.8057053079184));
#209087=CARTESIAN_POINT('Ctrl Pts',(-56.8735439783409,-79.0408979677858,
79.2472413050084));
#209088=CARTESIAN_POINT('Ctrl Pts',(-56.7576635028119,-83.1685327406974,
80.1477364670454));
#209089=CARTESIAN_POINT('Ctrl Pts',(-56.6417830272829,-87.3199288790655,
79.3640414392398));
#209090=CARTESIAN_POINT('Ctrl Pts',(-56.5259025517539,-90.8352126833059,
77.0207765453072));
#209091=CARTESIAN_POINT('Ctrl Pts',(-56.4100220762249,-93.155617208859,
73.4902227664913));
#209092=CARTESIAN_POINT('Ctrl Pts',(-56.3327684258729,-93.6600875746688,
70.7195859421521));
#209093=CARTESIAN_POINT('Ctrl Pts',(-56.2941416006959,-93.6316506207481,
69.3397002336783));
#209094=CARTESIAN_POINT('Ctrl Pts',(-63.4863639242949,-91.8230019028041,
74.5904921130553));
#209095=CARTESIAN_POINT('Ctrl Pts',(-63.4477370991189,-92.4970812476076,
73.4525899438658));
#209096=CARTESIAN_POINT('Ctrl Pts',(-63.3704834487659,-93.3820044778794,
70.903153272674));
#209097=CARTESIAN_POINT('Ctrl Pts',(-63.2546029732369,-93.1099627814073,
66.863814728757));
#209098=CARTESIAN_POINT('Ctrl Pts',(-63.1387224977069,-91.2813956951746,
63.2519304250261));
#209099=CARTESIAN_POINT('Ctrl Pts',(-63.0228420221779,-88.1870497514119,
60.6414643074804));
#209100=CARTESIAN_POINT('Ctrl Pts',(-62.9069615466489,-84.3187544758582,
59.4473977261369));
#209101=CARTESIAN_POINT('Ctrl Pts',(-62.7910810711199,-80.2913915654904,
59.8595194715136));
#209102=CARTESIAN_POINT('Ctrl Pts',(-62.6752005955899,-76.7451186061521,
61.8123247315614));
#209103=CARTESIAN_POINT('Ctrl Pts',(-62.5593201200609,-74.2436249664418,
64.9954094640758));
#209104=CARTESIAN_POINT('Ctrl Pts',(-62.4434396445319,-73.1845291497573,
68.9028146546496));
#209105=CARTESIAN_POINT('Ctrl Pts',(-62.3275591690019,-73.7361771014411,
72.9134484825933));
#209106=CARTESIAN_POINT('Ctrl Pts',(-62.2116786934729,-75.8108829998573,
76.3898107511057));
#209107=CARTESIAN_POINT('Ctrl Pts',(-62.0957982179439,-79.0788671899051,
78.7793250358795));
#209108=CARTESIAN_POINT('Ctrl Pts',(-61.9799177424139,-83.0206754640438,
79.7021721052772));
#209109=CARTESIAN_POINT('Ctrl Pts',(-61.8640372668849,-87.0097476031586,
79.0116631243528));
#209110=CARTESIAN_POINT('Ctrl Pts',(-61.7481567913549,-90.4120106791324,
76.8175562113822));
#209111=CARTESIAN_POINT('Ctrl Pts',(-61.6322763158259,-92.6866665225346,
73.468610111819));
#209112=CARTESIAN_POINT('Ctrl Pts',(-61.5163958402969,-93.4721529352706,
69.4971481292357));
#209113=CARTESIAN_POINT('Ctrl Pts',(-61.4005153647669,-92.6436149003541,
65.5344440135603));
#209114=CARTESIAN_POINT('Ctrl Pts',(-61.2846348892379,-90.332750597095,
62.210379430011));
#209115=CARTESIAN_POINT('Ctrl Pts',(-61.1687544137079,-86.9068776482263,
60.0533227033745));
#209116=CARTESIAN_POINT('Ctrl Pts',(-61.0528739381789,-82.9105470711673,
59.4061433599308));
#209117=CARTESIAN_POINT('Ctrl Pts',(-60.9369934626489,-78.9789855407346,
60.3717121643543));
#209118=CARTESIAN_POINT('Ctrl Pts',(-60.8211129871199,-75.7371245308333,
62.7965495560486));
#209119=CARTESIAN_POINT('Ctrl Pts',(-60.7052325115899,-73.7002659039675,
66.2952216066778));
#209120=CARTESIAN_POINT('Ctrl Pts',(-60.5893520360609,-73.192173399811,
70.3116057007245));
#209121=CARTESIAN_POINT('Ctrl Pts',(-60.4734715605309,-74.2936095843438,
74.2072876070263));
#209122=CARTESIAN_POINT('Ctrl Pts',(-60.3575910850019,-76.8294984393236,
77.3630390070701));
#209123=CARTESIAN_POINT('Ctrl Pts',(-60.2417106094719,-80.3967541303873,
79.277245374799));
#209124=CARTESIAN_POINT('Ctrl Pts',(-60.1258301339429,-84.4283525019679,
79.6456388518811));
#209125=CARTESIAN_POINT('Ctrl Pts',(-60.0099496584129,-88.2834609756893,
78.4096623797982));
#209126=CARTESIAN_POINT('Ctrl Pts',(-59.8940691828839,-91.3493004809464,
75.765777489781));
#209127=CARTESIAN_POINT('Ctrl Pts',(-59.7781887073549,-93.13854821078,72.1342362543011));
#209128=CARTESIAN_POINT('Ctrl Pts',(-59.6623082318249,-93.3667987928187,
68.0922811759415));
#209129=CARTESIAN_POINT('Ctrl Pts',(-59.5464277562959,-91.997771229922,
64.282391057355));
#209130=CARTESIAN_POINT('Ctrl Pts',(-59.4305472807659,-89.2490758548062,
61.3101573992296));
#209131=CARTESIAN_POINT('Ctrl Pts',(-59.3146668052369,-85.5576246269588,
59.6480241265653));
#209132=CARTESIAN_POINT('Ctrl Pts',(-59.1987863297069,-81.5101828911056,
59.5601914529124));
#209133=CARTESIAN_POINT('Ctrl Pts',(-59.0829058541779,-77.7501015677444,
61.0606205999848));
#209134=CARTESIAN_POINT('Ctrl Pts',(-58.9670253786489,-74.875054925804,
63.9108146267733));
#209135=CARTESIAN_POINT('Ctrl Pts',(-58.8511449031189,-73.3420387725811,
67.6577281109136));
#209136=CARTESIAN_POINT('Ctrl Pts',(-58.7352644275899,-73.3947298346776,
71.7057798442351));
#209137=CARTESIAN_POINT('Ctrl Pts',(-58.6193839520599,-75.0247527368537,
75.4115219456312));
#209138=CARTESIAN_POINT('Ctrl Pts',(-58.5035034765309,-77.9730112887291,
78.1859175005156));
#209139=CARTESIAN_POINT('Ctrl Pts',(-58.3876230010019,-81.7708724680175,
79.5879694419674));
#209140=CARTESIAN_POINT('Ctrl Pts',(-58.2717425254719,-85.8146568038164,
79.394818130247));
#209141=CARTESIAN_POINT('Ctrl Pts',(-58.1558620499429,-89.4615947284621,
77.6371654462713));
#209142=CARTESIAN_POINT('Ctrl Pts',(-58.0399815744139,-92.1319963973636,
74.5943946513581));
#209143=CARTESIAN_POINT('Ctrl Pts',(-57.9241010988849,-93.4013948301736,
70.7501617236546));
#209144=CARTESIAN_POINT('Ctrl Pts',(-57.8082206233549,-93.0680159919581,
66.7155170386891));
#209145=CARTESIAN_POINT('Ctrl Pts',(-57.6923401478259,-91.1848512773756,
63.1317773939326));
#209146=CARTESIAN_POINT('Ctrl Pts',(-57.5764596722969,-88.0512343968762,
60.568587110321));
#209147=CARTESIAN_POINT('Ctrl Pts',(-57.4605791967679,-84.1652615396361,
59.4333716522234));
#209148=CARTESIAN_POINT('Ctrl Pts',(-57.3446987212389,-80.1446177466814,
59.9065763370039));
#209149=CARTESIAN_POINT('Ctrl Pts',(-57.2288182457099,-76.6283943389352,
61.9129841055395));
#209150=CARTESIAN_POINT('Ctrl Pts',(-57.1129377701809,-74.1755037636287,
65.1336714529826));
#209151=CARTESIAN_POINT('Ctrl Pts',(-56.9970572946509,-73.1758390727135,
69.0567021408465));
#209152=CARTESIAN_POINT('Ctrl Pts',(-56.8811768191219,-73.7882994512876,
73.0585006275909));
#209153=CARTESIAN_POINT('Ctrl Pts',(-56.7652963435929,-75.9155328055053,
76.5029713478119));
#209154=CARTESIAN_POINT('Ctrl Pts',(-56.6494158680649,-79.2194100892149,
78.8426061994354));
#209155=CARTESIAN_POINT('Ctrl Pts',(-56.5335353925359,-83.1747718700718,
79.705517853136));
#209156=CARTESIAN_POINT('Ctrl Pts',(-56.4176549170069,-87.1529033003677,
78.9545315059016));
#209157=CARTESIAN_POINT('Ctrl Pts',(-56.3017744414779,-90.5214714933247,
76.7090662664086));
#209158=CARTESIAN_POINT('Ctrl Pts',(-56.1858939659489,-92.7450304759939,
73.3258654140387));
#209159=CARTESIAN_POINT('Ctrl Pts',(-56.1086403155959,-93.2284460188592,
70.6708652489211));
#209160=CARTESIAN_POINT('Ctrl Pts',(-56.0700134904199,-93.2011959236129,
69.348571128068));
#209161=CARTESIAN_POINT('Ctrl Pts',(-63.2622358140189,-91.452573473999,
74.371054836858));
#209162=CARTESIAN_POINT('Ctrl Pts',(-63.2236089888419,-92.0972937684766,
73.282713193911));
#209163=CARTESIAN_POINT('Ctrl Pts',(-63.1463553384899,-92.9436747917172,
70.8443154384341));
#209164=CARTESIAN_POINT('Ctrl Pts',(-63.0304748629609,-92.6834816794201,
66.9809074352464));
#209165=CARTESIAN_POINT('Ctrl Pts',(-62.9145943874309,-90.9345565426601,
63.5263362043601));
#209166=CARTESIAN_POINT('Ctrl Pts',(-62.7987139119019,-87.9749826535781,
61.0295670970088));
#209167=CARTESIAN_POINT('Ctrl Pts',(-62.6828334363729,-84.2751682498535,
59.8875072432627));
#209168=CARTESIAN_POINT('Ctrl Pts',(-62.5669529608439,-80.4232142899493,
60.2816793167476));
#209169=CARTESIAN_POINT('Ctrl Pts',(-62.4510724853139,-77.0313967476354,
62.1494315213011));
#209170=CARTESIAN_POINT('Ctrl Pts',(-62.3351920097849,-74.6388538987226,
65.1938792437981));
#209171=CARTESIAN_POINT('Ctrl Pts',(-62.2193115342559,-73.6258862531933,
68.9311001577751));
#209172=CARTESIAN_POINT('Ctrl Pts',(-62.1034310587259,-74.1535075675003,
72.7670536586458));
#209173=CARTESIAN_POINT('Ctrl Pts',(-61.9875505831969,-76.137851114111,
76.0920054209541));
#209174=CARTESIAN_POINT('Ctrl Pts',(-61.8716701076679,-79.26350055816,78.3774460967395));
#209175=CARTESIAN_POINT('Ctrl Pts',(-61.7557896321379,-83.0336261536677,
79.2600992130555));
#209176=CARTESIAN_POINT('Ctrl Pts',(-61.6399091566089,-86.8489570698533,
78.5996648636749));
#209177=CARTESIAN_POINT('Ctrl Pts',(-61.5240286810789,-90.1030369776855,
76.5011207294713));
#209178=CARTESIAN_POINT('Ctrl Pts',(-61.4081482055499,-92.2786217904858,
73.2980356147633));
#209179=CARTESIAN_POINT('Ctrl Pts',(-61.2922677300209,-93.0298968966431,
69.4995478571636));
#209180=CARTESIAN_POINT('Ctrl Pts',(-61.1763872544909,-92.2374452513553,
65.7094365237526));
#209181=CARTESIAN_POINT('Ctrl Pts',(-61.0605067789619,-90.0272290126204,
62.5301492281784));
#209182=CARTESIAN_POINT('Ctrl Pts',(-60.9446263034319,-86.7505675432666,
60.4670415855671));
#209183=CARTESIAN_POINT('Ctrl Pts',(-60.8287458279029,-82.9282943252811,
59.8480496818692));
#209184=CARTESIAN_POINT('Ctrl Pts',(-60.7128653523729,-79.1679691837779,
60.7715638181681));
#209185=CARTESIAN_POINT('Ctrl Pts',(-60.5969848768439,-76.0673051431882,
63.0907891278659));
#209186=CARTESIAN_POINT('Ctrl Pts',(-60.4811044013139,-74.1191604569068,
66.4370789854654));
#209187=CARTESIAN_POINT('Ctrl Pts',(-60.3652239257849,-73.6331975633271,
70.2785323036529));
#209188=CARTESIAN_POINT('Ctrl Pts',(-60.2493434502549,-74.6866614718425,
74.004540532737));
#209189=CARTESIAN_POINT('Ctrl Pts',(-60.1334629747259,-77.112101476679,
77.0228454067829));
#209190=CARTESIAN_POINT('Ctrl Pts',(-60.0175824991959,-80.5239878626353,
78.8536798665507));
#209191=CARTESIAN_POINT('Ctrl Pts',(-59.9017020236669,-84.3799928112316,
79.2060282256322));
#209192=CARTESIAN_POINT('Ctrl Pts',(-59.7858215481369,-88.0671947549688,
78.0238838368779));
#209193=CARTESIAN_POINT('Ctrl Pts',(-59.6699410726079,-90.9995037833793,
75.4951514881295));
#209194=CARTESIAN_POINT('Ctrl Pts',(-59.5540605970789,-92.7108220905774,
72.0217794692934));
#209195=CARTESIAN_POINT('Ctrl Pts',(-59.4381801215489,-92.9291313795479,
68.1558688929745));
#209196=CARTESIAN_POINT('Ctrl Pts',(-59.3222996460199,-91.6197308463801,
64.5119158508118));
#209197=CARTESIAN_POINT('Ctrl Pts',(-59.2064191704899,-88.9907529592742,
61.6691357328928));
#209198=CARTESIAN_POINT('Ctrl Pts',(-59.0905386949609,-85.4600802855175,
60.079395502359));
#209199=CARTESIAN_POINT('Ctrl Pts',(-58.9746582194309,-81.5889220192099,
59.9953883188284));
#209200=CARTESIAN_POINT('Ctrl Pts',(-58.8587777439019,-77.9926083853276,
61.4304673328671));
#209201=CARTESIAN_POINT('Ctrl Pts',(-58.7428972683729,-75.2427823716655,
64.1565231694806));
#209202=CARTESIAN_POINT('Ctrl Pts',(-58.6270167928429,-73.7765356555165,
67.7402424800745));
#209203=CARTESIAN_POINT('Ctrl Pts',(-58.5111363173139,-73.8269317955608,
71.6119841758515));
#209204=CARTESIAN_POINT('Ctrl Pts',(-58.3952558417839,-75.3859602001198,
75.1563252942432));
#209205=CARTESIAN_POINT('Ctrl Pts',(-58.2793753662549,-78.2058094306096,
77.8098840079436));
#209206=CARTESIAN_POINT('Ctrl Pts',(-58.1634948907259,-81.8382574454312,
79.1508705661768));
#209207=CARTESIAN_POINT('Ctrl Pts',(-58.0476144151959,-85.7059176071747,
78.9661318235942));
#209208=CARTESIAN_POINT('Ctrl Pts',(-57.9317339396669,-89.1940157232479,
77.2850324623463));
#209209=CARTESIAN_POINT('Ctrl Pts',(-57.8158534641379,-91.7481099313085,
74.3747874028884));
#209210=CARTESIAN_POINT('Ctrl Pts',(-57.6999729886089,-92.9622206108914,
70.6979873284379));
#209211=CARTESIAN_POINT('Ctrl Pts',(-57.5840925130789,-92.6433618528013,
66.8390687464838));
#209212=CARTESIAN_POINT('Ctrl Pts',(-57.4682120375499,-90.8422170489019,
63.4114163537942));
#209213=CARTESIAN_POINT('Ctrl Pts',(-57.3523315620209,-87.8450826410214,
60.9598640147741));
#209214=CARTESIAN_POINT('Ctrl Pts',(-57.2364510864919,-84.1283605902155,
59.8740920651051));
#209215=CARTESIAN_POINT('Ctrl Pts',(-57.1205706109629,-80.2828331013019,
60.3266866536539));
#209216=CARTESIAN_POINT('Ctrl Pts',(-57.0046901354339,-76.9197563235507,
62.2457067472406));
#209217=CARTESIAN_POINT('Ctrl Pts',(-56.8888096599039,-74.5736996668511,
65.326119329296));
#209218=CARTESIAN_POINT('Ctrl Pts',(-56.7729291843749,-73.6175746663254,
69.0782851830545));
#209219=CARTESIAN_POINT('Ctrl Pts',(-56.6570487088459,-74.2033597651635,
72.9057881597824));
#209220=CARTESIAN_POINT('Ctrl Pts',(-56.5411682333169,-76.2379429712918,
76.2002373876932));
#209221=CARTESIAN_POINT('Ctrl Pts',(-56.4252877577879,-79.3979222106296,
78.4379710938565));
#209222=CARTESIAN_POINT('Ctrl Pts',(-56.3094072822599,-83.1810109994346,
79.263299239227));
#209223=CARTESIAN_POINT('Ctrl Pts',(-56.1935268067309,-86.9858777216637,
78.545021572567));
#209224=CARTESIAN_POINT('Ctrl Pts',(-56.0776463312019,-90.2077303033346,
76.3973559875148));
#209225=CARTESIAN_POINT('Ctrl Pts',(-55.9617658556729,-92.3344437431285,
73.1615080615852));
#209226=CARTESIAN_POINT('Ctrl Pts',(-55.8845122053199,-92.7968044630577,
70.6221445556835));
#209227=CARTESIAN_POINT('Ctrl Pts',(-55.8458853801439,-92.7707412264758,
69.357442022453));
#209228=CARTESIAN_POINT('Ctrl Pts',(-63.0381077037429,-91.0821450451938,
74.1516175606607));
#209229=CARTESIAN_POINT('Ctrl Pts',(-62.9994808785659,-91.6975062893363,
73.1128364439599));
#209230=CARTESIAN_POINT('Ctrl Pts',(-62.9222272282139,-92.5053451055553,
70.7854776041952));
#209231=CARTESIAN_POINT('Ctrl Pts',(-62.8063467526839,-92.2570005774417,
67.098000141731));
#209232=CARTESIAN_POINT('Ctrl Pts',(-62.6904662771549,-90.5877173901553,
63.8007419836912));
#209233=CARTESIAN_POINT('Ctrl Pts',(-62.5745858016259,-87.7629155557435,
61.4176698865353));
#209234=CARTESIAN_POINT('Ctrl Pts',(-62.4587053260969,-84.2315820238582,
60.3276167603847));
#209235=CARTESIAN_POINT('Ctrl Pts',(-62.3428248505679,-80.5550370144063,
60.7038391619823));
#209236=CARTESIAN_POINT('Ctrl Pts',(-62.2269443750379,-77.3176748891168,
62.4865383110414));
#209237=CARTESIAN_POINT('Ctrl Pts',(-62.1110638995089,-75.0340828310024,
65.3923490235231));
#209238=CARTESIAN_POINT('Ctrl Pts',(-61.9951834239799,-74.0672433566291,
68.9593856609049));
#209239=CARTESIAN_POINT('Ctrl Pts',(-61.8793029484499,-74.570838033561,
72.620658834703));
#209240=CARTESIAN_POINT('Ctrl Pts',(-61.7634224729209,-76.4648192283687,
75.7942000908074));
#209241=CARTESIAN_POINT('Ctrl Pts',(-61.6475419973919,-79.4481339264209,
77.9755671576036));
#209242=CARTESIAN_POINT('Ctrl Pts',(-61.5316615218619,-83.0465768432993,
78.8180263208338));
#209243=CARTESIAN_POINT('Ctrl Pts',(-61.4157810463329,-86.6881665365578,
78.1876666029972));
#209244=CARTESIAN_POINT('Ctrl Pts',(-61.2999005708029,-89.7940632762463,
76.1846852475528));
#209245=CARTESIAN_POINT('Ctrl Pts',(-61.1840200952739,-91.8705770584431,
73.1274611176964));
#209246=CARTESIAN_POINT('Ctrl Pts',(-61.0681396197439,-92.5876408580107,
69.5019475850796));
#209247=CARTESIAN_POINT('Ctrl Pts',(-60.9522591442149,-91.8312756023416,
65.8844290339352));
#209248=CARTESIAN_POINT('Ctrl Pts',(-60.8363786686859,-89.7217074281312,
62.8499190263368));
#209249=CARTESIAN_POINT('Ctrl Pts',(-60.7204981931559,-86.5942574382841,
60.8807604677571));
#209250=CARTESIAN_POINT('Ctrl Pts',(-60.6046177176269,-82.9460415793733,
60.2899560038079));
#209251=CARTESIAN_POINT('Ctrl Pts',(-60.4887372420969,-79.3569528268042,
61.1714154719932));
#209252=CARTESIAN_POINT('Ctrl Pts',(-60.3728567665679,-76.3974857555292,
63.3850286996998));
#209253=CARTESIAN_POINT('Ctrl Pts',(-60.2569762910379,-74.5380550098396,
66.578936364274));
#209254=CARTESIAN_POINT('Ctrl Pts',(-60.1410958155089,-74.0742217268447,
70.2454589066055));
#209255=CARTESIAN_POINT('Ctrl Pts',(-60.0252153399789,-75.0797133593528,
73.8017934584711));
#209256=CARTESIAN_POINT('Ctrl Pts',(-59.9093348644499,-77.3947045140554,
76.682651806513));
#209257=CARTESIAN_POINT('Ctrl Pts',(-59.7934543889199,-80.65122159491,78.430114358312));
#209258=CARTESIAN_POINT('Ctrl Pts',(-59.6775739133909,-84.3316331205256,
78.7664175993805));
#209259=CARTESIAN_POINT('Ctrl Pts',(-59.5616934378609,-87.850928534276,
77.6381052939461));
#209260=CARTESIAN_POINT('Ctrl Pts',(-59.4458129623319,-90.6497070858334,
75.2245254864509));
#209261=CARTESIAN_POINT('Ctrl Pts',(-59.3299324868019,-92.283095970383,
71.9093226842531));
#209262=CARTESIAN_POINT('Ctrl Pts',(-59.2140520112729,-92.4914639662642,
68.2194566099759));
#209263=CARTESIAN_POINT('Ctrl Pts',(-59.0981715357439,-91.2416904628249,
64.7414406442362));
#209264=CARTESIAN_POINT('Ctrl Pts',(-58.9822910602139,-88.7324300637027,
62.0281140665388));
#209265=CARTESIAN_POINT('Ctrl Pts',(-58.8664105846849,-85.3625359440494,
60.5107668781401));
#209266=CARTESIAN_POINT('Ctrl Pts',(-58.7505301091549,-81.6676611472649,
60.4305851847562));
#209267=CARTESIAN_POINT('Ctrl Pts',(-58.6346496336259,-78.2351152028796,
61.8003140657709));
#209268=CARTESIAN_POINT('Ctrl Pts',(-58.5187691580959,-75.6105098175054,
64.4022317122195));
#209269=CARTESIAN_POINT('Ctrl Pts',(-58.4028886825669,-74.2110325384453,
67.822756849275));
#209270=CARTESIAN_POINT('Ctrl Pts',(-58.2870082070379,-74.259133756452,
71.5181885075058));
#209271=CARTESIAN_POINT('Ctrl Pts',(-58.1711277315079,-75.7471676634089,
74.901128642888));
#209272=CARTESIAN_POINT('Ctrl Pts',(-58.0552472559789,-78.4386075725234,
77.4338505153925));
#209273=CARTESIAN_POINT('Ctrl Pts',(-57.9393667804499,-81.9056424228852,
78.7137716903922));
#209274=CARTESIAN_POINT('Ctrl Pts',(-57.8234863049199,-85.5971784105718,
78.5374455169307));
#209275=CARTESIAN_POINT('Ctrl Pts',(-57.7076058293909,-88.9264367180665,
76.9328994783958));
#209276=CARTESIAN_POINT('Ctrl Pts',(-57.5917253538619,-91.3642234652816,
74.1551801543822));
#209277=CARTESIAN_POINT('Ctrl Pts',(-57.4758448783329,-92.523046391615,
70.6458129331831));
#209278=CARTESIAN_POINT('Ctrl Pts',(-57.3599644028029,-92.2187077136396,
66.9626204542406));
#209279=CARTESIAN_POINT('Ctrl Pts',(-57.2440839272739,-90.4995828203968,
63.6910553136321));
#209280=CARTESIAN_POINT('Ctrl Pts',(-57.1282034517449,-87.6389308851381,
61.3511409192107));
#209281=CARTESIAN_POINT('Ctrl Pts',(-57.0123229762159,-84.091459640771,
60.3148124779814));
#209282=CARTESIAN_POINT('Ctrl Pts',(-56.8964425006869,-80.4210484558933,
60.7467969703094));
#209283=CARTESIAN_POINT('Ctrl Pts',(-56.7805620251579,-77.2111183081457,
62.57842938896));
#209284=CARTESIAN_POINT('Ctrl Pts',(-56.6646815496279,-74.9718955700618,
65.5185672056337));
#209285=CARTESIAN_POINT('Ctrl Pts',(-56.5488010740989,-74.0593102599364,
69.0998682252855));
#209286=CARTESIAN_POINT('Ctrl Pts',(-56.4329205985699,-74.6184200790472,
72.7530756919931));
#209287=CARTESIAN_POINT('Ctrl Pts',(-56.3170401230409,-76.560353137091,
75.8975034275876));
#209288=CARTESIAN_POINT('Ctrl Pts',(-56.2011596475119,-79.5764343320587,
78.0333359882835));
#209289=CARTESIAN_POINT('Ctrl Pts',(-56.0852791719829,-83.18725012881,78.8210806253173));
#209290=CARTESIAN_POINT('Ctrl Pts',(-55.9693986964549,-86.8188521429664,
78.1355116392275));
#209291=CARTESIAN_POINT('Ctrl Pts',(-55.8535182209259,-89.8939891133529,
76.0856457086153));
#209292=CARTESIAN_POINT('Ctrl Pts',(-55.7376377453969,-91.9238570102634,
72.9971507091326));
#209293=CARTESIAN_POINT('Ctrl Pts',(-55.6603840950439,-92.3651629072477,
70.5734238624515));
#209294=CARTESIAN_POINT('Ctrl Pts',(-55.6217572698679,-92.3402865293407,
69.3663129168427));
#209295=CARTESIAN_POINT('',(-63.5337774910882,-93.5594520463458,69.970329252864));
#209296=CARTESIAN_POINT('',(-63.5337571161032,-93.5594128863229,69.970328227734));
#209297=CARTESIAN_POINT('Ctrl Pts',(-63.5337978660732,-93.5594912063686,
69.970330277994));
#209298=CARTESIAN_POINT('Ctrl Pts',(-63.5216568454269,-93.5772513864428,
69.5352741201867));
#209299=CARTESIAN_POINT('Ctrl Pts',(-63.5094960824503,-93.567271818938,
69.0995306219549));
#209300=CARTESIAN_POINT('Ctrl Pts',(-63.4851355856958,-93.4926516929353,
68.2399799410843));
#209301=CARTESIAN_POINT('Ctrl Pts',(-63.4729651705743,-93.4290976072566,
67.8169422519278));
#209302=CARTESIAN_POINT('Ctrl Pts',(-63.4379180895563,-93.1701049116124,
66.6115153529615));
#209303=CARTESIAN_POINT('Ctrl Pts',(-63.4157214108481,-92.9086267996816,
65.8466098604295));
#209304=CARTESIAN_POINT('Ctrl Pts',(-63.3779422794529,-92.3269878674592,
64.6336904127012));
#209305=CARTESIAN_POINT('Ctrl Pts',(-63.3626137085537,-92.0556170188198,
64.1663309373524));
#209306=CARTESIAN_POINT('Ctrl Pts',(-63.3174905710142,-91.1530081274075,
62.8610167967825));
#209307=CARTESIAN_POINT('Ctrl Pts',(-63.2888250790043,-90.4287485210572,
62.0958974953315));
#209308=CARTESIAN_POINT('Ctrl Pts',(-63.2498582130389,-89.3411459094481,
61.2520762780945));
#209309=CARTESIAN_POINT('Ctrl Pts',(-63.2404883841634,-89.0715219048256,
61.0629540782528));
#209310=CARTESIAN_POINT('Ctrl Pts',(-63.2015300107886,-87.9132450973876,
60.3310706918349));
#209311=CARTESIAN_POINT('Ctrl Pts',(-63.1730383758105,-86.9536282367546,
59.9123017459371));
#209312=CARTESIAN_POINT('Ctrl Pts',(-63.134252165677,-85.6291328319174,
59.5607618447651));
#209313=CARTESIAN_POINT('Ctrl Pts',(-63.1248770310096,-85.3069013144664,
59.4916621526057));
#209314=CARTESIAN_POINT('Ctrl Pts',(-63.085746995258,-83.9490150716827,
59.2682734165905));
#209315=CARTESIAN_POINT('Ctrl Pts',(-63.0570979218165,-82.8961668763337,
59.2575730468926));
#209316=CARTESIAN_POINT('Ctrl Pts',(-63.0181490486881,-81.5341877143882,
59.4532947949565));
#209317=CARTESIAN_POINT('Ctrl Pts',(-63.0087782602271,-81.2107874689418,
59.5157903455767));
#209318=CARTESIAN_POINT('Ctrl Pts',(-62.9697840933728,-79.878386152212,
59.8405200251187));
#209319=CARTESIAN_POINT('Ctrl Pts',(-62.9412592415125,-78.9093534753847,
60.2402985218569));
#209320=CARTESIAN_POINT('Ctrl Pts',(-62.896957577525,-77.5697157187439,
61.049717858937));
#209321=CARTESIAN_POINT('Ctrl Pts',(-62.8820052873794,-77.1434642908388,
61.3540239697376));
#209322=CARTESIAN_POINT('Ctrl Pts',(-62.857887191323,-76.4879137579722,
61.9022713082005));
#209323=CARTESIAN_POINT('Ctrl Pts',(-62.8486522391764,-76.2440012611628,
62.1272393924664));
#209324=CARTESIAN_POINT('Ctrl Pts',(-62.8017138500491,-75.063531698435,
63.3270843462837));
#209325=CARTESIAN_POINT('Ctrl Pts',(-62.76323536298,-74.3154953579531,64.468569951771));
#209326=CARTESIAN_POINT('Ctrl Pts',(-62.6904861241906,-73.3407129438074,
66.8883539708659));
#209327=CARTESIAN_POINT('Ctrl Pts',(-62.6546385270754,-73.089478660267,
68.1310048344221));
#209328=CARTESIAN_POINT('Ctrl Pts',(-62.6006605552128,-73.0585228854009,
70.062917874554));
#209329=CARTESIAN_POINT('Ctrl Pts',(-62.5819189575496,-73.1143987731514,
70.7372259394319));
#209330=CARTESIAN_POINT('Ctrl Pts',(-62.543672183343,-73.3580133050627,
72.0656433597821));
#209331=CARTESIAN_POINT('Ctrl Pts',(-62.52435918621,-73.5452782999503,72.7164894035513));
#209332=CARTESIAN_POINT('Ctrl Pts',(-62.5042445607632,-73.8114572910648,
73.3849557517124));
#209333=CARTESIAN_POINT('Ctrl Pts',(-62.503018276399,-73.8279591515225,
73.4256350243488));
#209334=CARTESIAN_POINT('Ctrl Pts',(-62.5017927901943,-73.8447192658304,
73.466201051278));
#209335=CARTESIAN_POINT('',(-56.402655786563,-92.4407016401285,74.2253115652726));
#209336=CARTESIAN_POINT('Ctrl Pts',(-56.5793858481529,-89.1716495247985,
78.0464295027995));
#209337=CARTESIAN_POINT('Ctrl Pts',(-56.5407590229759,-90.3081071926132,
77.2632582583921));
#209338=CARTESIAN_POINT('Ctrl Pts',(-56.4635053726229,-92.2618542008096,
75.2350099031932));
#209339=CARTESIAN_POINT('Ctrl Pts',(-56.3476248970939,-93.7712830739489,
71.289035799845));
#209340=CARTESIAN_POINT('Ctrl Pts',(-56.2317444215639,-93.6190186885821,
67.0670781799152));
#209341=CARTESIAN_POINT('Ctrl Pts',(-56.1158639460339,-91.8294176899935,
63.2401216789652));
#209342=CARTESIAN_POINT('Ctrl Pts',(-55.9999834705049,-88.686900381402,
60.4164989490926));
#209343=CARTESIAN_POINT('Ctrl Pts',(-55.8841029949749,-84.6909887425699,
59.0450242272283));
#209344=CARTESIAN_POINT('Ctrl Pts',(-55.7682225194459,-80.4768398974234,
59.3436988676507));
#209345=CARTESIAN_POINT('Ctrl Pts',(-55.6523420439159,-76.7143040687269,
61.2650472476524));
#209346=CARTESIAN_POINT('Ctrl Pts',(-55.5364615683869,-74.0014454626398,
64.5036664147486));
#209347=CARTESIAN_POINT('Ctrl Pts',(-55.4205810928579,-72.7694797521119,
68.5447697661598));
#209348=CARTESIAN_POINT('Ctrl Pts',(-55.3047006173279,-73.2142309326136,
72.746013893864));
#209349=CARTESIAN_POINT('Ctrl Pts',(-55.1888201417989,-75.2650047030302,
76.4396006022121));
#209350=CARTESIAN_POINT('Ctrl Pts',(-55.0729396662689,-78.5958254759494,
79.0384251072975));
#209351=CARTESIAN_POINT('Ctrl Pts',(-54.9570591907399,-82.6772510137972,
80.1293977965975));
#209352=CARTESIAN_POINT('Ctrl Pts',(-54.8411787152099,-86.8605285862284,
79.5391058504835));
#209353=CARTESIAN_POINT('Ctrl Pts',(-54.7252982396809,-90.4807158290425,
77.3613776404707));
#209354=CARTESIAN_POINT('Ctrl Pts',(-54.6094177641509,-92.9623749849825,
73.9423684764853));
#209355=CARTESIAN_POINT('Ctrl Pts',(-54.4935372886209,-93.9110401651089,
69.8255383602718));
#209356=CARTESIAN_POINT('Ctrl Pts',(-54.3776568130909,-93.1759186818892,
65.6652676678046));
#209357=CARTESIAN_POINT('Ctrl Pts',(-54.2617763375609,-90.8738599216446,
62.1228417625684));
#209358=CARTESIAN_POINT('Ctrl Pts',(-54.1458958620309,-87.3707818441818,
59.7613380439862));
#209359=CARTESIAN_POINT('Ctrl Pts',(-54.0300153865009,-83.2235074139119,
58.956123395707));
#209360=CARTESIAN_POINT('Ctrl Pts',(-53.9141349109709,-79.0912562061879,
59.8351886867613));
#209361=CARTESIAN_POINT('Ctrl Pts',(-53.7982544354409,-75.6308598177706,
62.258804304951));
#209362=CARTESIAN_POINT('Ctrl Pts',(-53.6823739599209,-73.3923568525672,
65.8417305258611));
#209363=CARTESIAN_POINT('Ctrl Pts',(-53.5664934843909,-72.7315629188536,
70.0144523242639));
#209364=CARTESIAN_POINT('Ctrl Pts',(-53.4506130088609,-73.7535128542524,
74.113705202441));
#209365=CARTESIAN_POINT('Ctrl Pts',(-53.3347325333309,-76.2957651773164,
77.487902730087));
#209366=CARTESIAN_POINT('Ctrl Pts',(-53.2188520578009,-79.9542225646198,
79.6007078263948));
#209367=CARTESIAN_POINT('Ctrl Pts',(-53.1029715822709,-84.1473641243655,
80.1162848716646));
#209368=CARTESIAN_POINT('Ctrl Pts',(-52.9870911067409,-88.2086795870379,
78.9526816135227));
#209369=CARTESIAN_POINT('Ctrl Pts',(-52.8712106312109,-91.4926127687853,
76.2948556810079));
#209370=CARTESIAN_POINT('Ctrl Pts',(-52.7553301556809,-93.477174330855,
72.5652751099481));
#209371=CARTESIAN_POINT('Ctrl Pts',(-52.6394496801509,-93.84691328197,68.3567659989079));
#209372=CARTESIAN_POINT('Ctrl Pts',(-52.5235692046209,-92.5430586971659,
64.338281327871));
#209373=CARTESIAN_POINT('Ctrl Pts',(-52.4076887290909,-89.7728615023466,
61.1485692199366));
#209374=CARTESIAN_POINT('Ctrl Pts',(-52.2918082535609,-85.9766514246951,
59.2946423400516));
#209375=CARTESIAN_POINT('Ctrl Pts',(-52.1759277780309,-81.7578454883824,
59.0711869721971));
#209376=CARTESIAN_POINT('Ctrl Pts',(-52.0600473025109,-77.7870333793684,
60.5137219022862));
#209377=CARTESIAN_POINT('Ctrl Pts',(-51.9441668269809,-74.6953855485565,
63.3929526189662));
#209378=CARTESIAN_POINT('Ctrl Pts',(-51.8282863514509,-72.9743271003957,
67.2512182458574));
#209379=CARTESIAN_POINT('Ctrl Pts',(-51.7124058759209,-72.8974245514948,
71.4752378750255));
#209380=CARTESIAN_POINT('Ctrl Pts',(-51.5965254003909,-74.4769017530788,
75.3935930910951));
#209381=CARTESIAN_POINT('Ctrl Pts',(-51.4806449248609,-77.4616968794652,
78.383451596628));
#209382=CARTESIAN_POINT('Ctrl Pts',(-51.3647644493309,-81.3773693290668,
79.9695679533435));
#209383=CARTESIAN_POINT('Ctrl Pts',(-51.2488839738009,-85.6015132368418,
79.8998250253565));
#209384=CARTESIAN_POINT('Ctrl Pts',(-51.1330034982709,-89.462690433018,
78.1853086243629));
#209385=CARTESIAN_POINT('Ctrl Pts',(-51.0171230227409,-92.3471572085029,
75.0985453923105));
#209386=CARTESIAN_POINT('Ctrl Pts',(-50.9012425472109,-93.7964204023591,
71.1301840145485));
#209387=CARTESIAN_POINT('Ctrl Pts',(-50.7853620716809,-93.5801160289695,
66.9110053921681));
#209388=CARTESIAN_POINT('Ctrl Pts',(-50.6694815961509,-91.7326262059582,
63.111658450455));
#209389=CARTESIAN_POINT('Ctrl Pts',(-50.5536011206309,-88.5476140310613,
60.3360588260279));
#209390=CARTESIAN_POINT('Ctrl Pts',(-50.4377206451009,-84.5313451033357,
59.0253949753285));
#209391=CARTESIAN_POINT('Ctrl Pts',(-50.3218401695709,-80.3222153474369,
59.3880001752185));
#209392=CARTESIAN_POINT('Ctrl Pts',(-50.2059596940409,-76.5892763983811,
61.3662374236589));
#209393=CARTESIAN_POINT('Ctrl Pts',(-50.0900792185109,-73.9258881698316,
64.6456610117156));
#209394=CARTESIAN_POINT('Ctrl Pts',(-49.9741987429809,-72.7554028660613,
68.7049983484054));
#209395=CARTESIAN_POINT('Ctrl Pts',(-49.8583182674509,-73.2638719310397,
72.8990079143938));
#209396=CARTESIAN_POINT('Ctrl Pts',(-49.7424377919209,-75.3704733291652,
76.5610405859094));
#209397=CARTESIAN_POINT('Ctrl Pts',(-49.6265573163909,-78.7403560946919,
79.1090104644245));
#209398=CARTESIAN_POINT('Ctrl Pts',(-49.5106768408609,-82.8378743604903,
80.1378991151166));
#209399=CARTESIAN_POINT('Ctrl Pts',(-49.3947963653309,-87.0116973704533,
79.4842080039733));
#209400=CARTESIAN_POINT('Ctrl Pts',(-49.2789158898109,-90.5984604020873,
77.251671755215));
#209401=CARTESIAN_POINT('Ctrl Pts',(-49.2016622394509,-92.2179930301717,
74.9477549101844));
#209402=CARTESIAN_POINT('Ctrl Pts',(-49.1630354142809,-92.7706651531469,
73.6830625549966));
#209403=CARTESIAN_POINT('Ctrl Pts',(-56.3552577378769,-88.9273396238135,
77.6919120683441));
#209404=CARTESIAN_POINT('Ctrl Pts',(-56.3166309126999,-90.0163655362671,
76.9414276436266));
#209405=CARTESIAN_POINT('Ctrl Pts',(-56.2393772623469,-91.8885699997907,
74.9978312579016));
#209406=CARTESIAN_POINT('Ctrl Pts',(-56.1234967868169,-93.335000608173,
71.2165482676822));
#209407=CARTESIAN_POINT('Ctrl Pts',(-56.0076163112879,-93.1890912039718,
67.1708003444751));
#209408=CARTESIAN_POINT('Ctrl Pts',(-55.8917358357579,-91.4741818715764,
63.5035675795474));
#209409=CARTESIAN_POINT('Ctrl Pts',(-55.7758553602289,-88.4628222087298,
60.7977929546752));
#209410=CARTESIAN_POINT('Ctrl Pts',(-55.6599748846989,-84.6336859005426,
59.4835587753601));
#209411=CARTESIAN_POINT('Ctrl Pts',(-55.5440944091699,-80.5954208412564,
59.7697677843112));
#209412=CARTESIAN_POINT('Ctrl Pts',(-55.4282139336399,-76.9899200557673,
61.6109258247081));
#209413=CARTESIAN_POINT('Ctrl Pts',(-55.3123334581109,-74.3902866488067,
64.7143763916865));
#209414=CARTESIAN_POINT('Ctrl Pts',(-55.1964529825809,-73.2097388642188,
68.58681826895));
#209415=CARTESIAN_POINT('Ctrl Pts',(-55.0805725070519,-73.6359276910248,
72.6127172084169));
#209416=CARTESIAN_POINT('Ctrl Pts',(-54.9646920315229,-75.6011093601795,
76.152146567904));
#209417=CARTESIAN_POINT('Ctrl Pts',(-54.8488115559929,-78.7929133614815,
78.6425052571067));
#209418=CARTESIAN_POINT('Ctrl Pts',(-54.7329310804639,-82.7039945186047,
79.687944574445));
#209419=CARTESIAN_POINT('Ctrl Pts',(-54.6170506049339,-86.7126767637781,
79.1222893429069));
#209420=CARTESIAN_POINT('Ctrl Pts',(-54.5011701294009,-90.1817700938727,
77.035451866986));
#209421=CARTESIAN_POINT('Ctrl Pts',(-54.3852896538709,-92.5598535044851,
73.7591401486176));
#209422=CARTESIAN_POINT('Ctrl Pts',(-54.2694091783509,-93.4689247287331,
69.8141320760029));
#209423=CARTESIAN_POINT('Ctrl Pts',(-54.1535287028209,-92.764484636779,
65.8274964843525));
#209424=CARTESIAN_POINT('Ctrl Pts',(-54.0376482272909,-90.5585057315378,
62.4329190064618));
#209425=CARTESIAN_POINT('Ctrl Pts',(-53.9217677517609,-87.2016338411459,
60.1699761668685));
#209426=CARTESIAN_POINT('Ctrl Pts',(-53.8058872762309,-83.2274520933251,
59.3983683526049));
#209427=CARTESIAN_POINT('Ctrl Pts',(-53.6900068007009,-79.2676665514421,
60.2407445429474));
#209428=CARTESIAN_POINT('Ctrl Pts',(-53.5741263251709,-75.9516949661677,
62.5632069494066));
#209429=CARTESIAN_POINT('Ctrl Pts',(-53.4582458496409,-73.8066192600998,
65.9965944019082));
#209430=CARTESIAN_POINT('Ctrl Pts',(-53.3423653741109,-73.1734045465354,
69.9951614340195));
#209431=CARTESIAN_POINT('Ctrl Pts',(-53.2264848985809,-74.15270187753,73.9233258808396));
#209432=CARTESIAN_POINT('Ctrl Pts',(-53.1106044230509,-76.5888495090847,
77.1566962433291));
#209433=CARTESIAN_POINT('Ctrl Pts',(-52.9947239475209,-80.0946157221245,
79.1813202684909));
#209434=CARTESIAN_POINT('Ctrl Pts',(-52.8788434719909,-84.1127502663909,
79.6753789369893));
#209435=CARTESIAN_POINT('Ctrl Pts',(-52.7629629964609,-88.0045606723086,
78.5603403958907));
#209436=CARTESIAN_POINT('Ctrl Pts',(-52.6470825209309,-91.1514340059658,
76.0134427918171));
#209437=CARTESIAN_POINT('Ctrl Pts',(-52.5312020454009,-93.053166932025,
72.4395218271453));
#209438=CARTESIAN_POINT('Ctrl Pts',(-52.4153215698809,-93.4074742766868,
68.4066611192533));
#209439=CARTESIAN_POINT('Ctrl Pts',(-52.2994410943509,-92.1580380071747,
64.5558938980169));
#209440=CARTESIAN_POINT('Ctrl Pts',(-52.1835606188209,-89.5034591229898,
61.4993091811534));
#209441=CARTESIAN_POINT('Ctrl Pts',(-52.0676801432909,-85.8656895335373,
59.7227587040344));
#209442=CARTESIAN_POINT('Ctrl Pts',(-51.9517996677609,-81.8229617537302,
59.5086295791554));
#209443=CARTESIAN_POINT('Ctrl Pts',(-51.8359191922309,-78.0178774090514,
60.8909581629449));
#209444=CARTESIAN_POINT('Ctrl Pts',(-51.7200387167009,-75.0552641104844,
63.6500198923845));
#209445=CARTESIAN_POINT('Ctrl Pts',(-51.6041582411709,-73.4060366029682,
67.3472550501956));
#209446=CARTESIAN_POINT('Ctrl Pts',(-51.4882777656409,-73.3323436966194,
71.3949789216125));
#209447=CARTESIAN_POINT('Ctrl Pts',(-51.3723972901109,-74.8458990620047,
75.1497957399931));
#209448=CARTESIAN_POINT('Ctrl Pts',(-51.2565168145809,-77.7061193131001,
78.0148680425531));
#209449=CARTESIAN_POINT('Ctrl Pts',(-51.1406363390509,-81.4583653342733,
79.534785468025));
#209450=CARTESIAN_POINT('Ctrl Pts',(-51.0247558635209,-85.5062082973436,
79.4679533651301));
#209451=CARTESIAN_POINT('Ctrl Pts',(-50.9088753880009,-89.206233505757,
77.8249948626797));
#209452=CARTESIAN_POINT('Ctrl Pts',(-50.7929949124709,-91.9703127592713,
74.8670622968578));
#209453=CARTESIAN_POINT('Ctrl Pts',(-50.6771144369409,-93.3590887926927,
71.06432639851));
#209454=CARTESIAN_POINT('Ctrl Pts',(-50.5612339614109,-93.1518122048732,
67.0212414872382));
#209455=CARTESIAN_POINT('Ctrl Pts',(-50.4453534858809,-91.3814301244552,
63.3804659554293));
#209456=CARTESIAN_POINT('Ctrl Pts',(-50.3294730103509,-88.3293491819053,
60.7207101200916));
#209457=CARTESIAN_POINT('Ctrl Pts',(-50.2135925348209,-84.4807052266326,
59.4647487795594));
#209458=CARTESIAN_POINT('Ctrl Pts',(-50.0977120592909,-80.447249777423,
59.8122201107395));
#209459=CARTESIAN_POINT('Ctrl Pts',(-49.9818315837609,-76.8701106016706,
61.7078926778295));
#209460=CARTESIAN_POINT('Ctrl Pts',(-49.8659511082309,-74.3178828522775,
64.8504446324207));
#209461=CARTESIAN_POINT('Ctrl Pts',(-49.7500706327009,-73.1962494979973,
68.7403594723971));
#209462=CARTESIAN_POINT('Ctrl Pts',(-49.6341901571709,-73.6834968483606,
72.7593257953695));
#209463=CARTESIAN_POINT('Ctrl Pts',(-49.5183096816509,-75.7021760959367,
76.2685180728017));
#209464=CARTESIAN_POINT('Ctrl Pts',(-49.4024292061209,-78.9314117793381,
78.710144629103));
#209465=CARTESIAN_POINT('Ctrl Pts',(-49.2865487305909,-82.8579140104155,
79.6960910777588));
#209466=CARTESIAN_POINT('Ctrl Pts',(-49.1706682550609,-86.8575362933791,
79.0696827398739));
#209467=CARTESIAN_POINT('Ctrl Pts',(-49.0547877795309,-90.2946004215829,
76.9303247204407));
#209468=CARTESIAN_POINT('Ctrl Pts',(-48.9775341291809,-91.8465394405205,
74.7225652803544));
#209469=CARTESIAN_POINT('Ctrl Pts',(-48.9389073040009,-92.3761449683377,
73.5106567464228));
#209470=CARTESIAN_POINT('Ctrl Pts',(-56.1311296275999,-88.6830297228196,
77.3373946338934));
#209471=CARTESIAN_POINT('Ctrl Pts',(-56.0925028024239,-89.7246238799117,
76.6195970288649));
#209472=CARTESIAN_POINT('Ctrl Pts',(-56.0152491520709,-91.5152857987813,
74.760652612607));
#209473=CARTESIAN_POINT('Ctrl Pts',(-55.8993686765409,-92.8987181423976,
71.1440607355203));
#209474=CARTESIAN_POINT('Ctrl Pts',(-55.7834882010119,-92.7591637193615,
67.274522509035));
#209475=CARTESIAN_POINT('Ctrl Pts',(-55.6676077254819,-91.1189460531508,
63.7670134801353));
#209476=CARTESIAN_POINT('Ctrl Pts',(-55.5517272499529,-88.2387440360669,
61.179086960254));
#209477=CARTESIAN_POINT('Ctrl Pts',(-55.4358467744229,-84.5763830585068,
59.9220933234976));
#209478=CARTESIAN_POINT('Ctrl Pts',(-55.3199662988939,-80.7140017850856,
60.1958367009625));
#209479=CARTESIAN_POINT('Ctrl Pts',(-55.2040858233639,-77.2655360428094,
61.9568044017577));
#209480=CARTESIAN_POINT('Ctrl Pts',(-55.0882053478349,-74.7791278349758,
64.9250863686191));
#209481=CARTESIAN_POINT('Ctrl Pts',(-54.9723248723049,-73.6499979763262,
68.6288667717323));
#209482=CARTESIAN_POINT('Ctrl Pts',(-54.8564443967759,-74.0576244494326,
72.4794205229618));
#209483=CARTESIAN_POINT('Ctrl Pts',(-54.7405639212469,-75.9372140173222,
75.8646925335888));
#209484=CARTESIAN_POINT('Ctrl Pts',(-54.6246834457169,-78.9900012470032,
78.2465854069093));
#209485=CARTESIAN_POINT('Ctrl Pts',(-54.5088029701909,-82.7307380233984,
79.2464913522906));
#209486=CARTESIAN_POINT('Ctrl Pts',(-54.3929224946609,-86.5648249413073,
78.7054728353225));
#209487=CARTESIAN_POINT('Ctrl Pts',(-54.2770420191309,-89.8828243586779,
76.7095260935192));
#209488=CARTESIAN_POINT('Ctrl Pts',(-54.1611615436009,-92.1573320239741,
73.5759118207695));
#209489=CARTESIAN_POINT('Ctrl Pts',(-54.0452810680709,-93.026809292365,
69.8027257917525));
#209490=CARTESIAN_POINT('Ctrl Pts',(-53.9294005925409,-92.353050591669,
65.9897253009272));
#209491=CARTESIAN_POINT('Ctrl Pts',(-53.8135201170109,-90.2431515414503,
62.7429962503755));
#209492=CARTESIAN_POINT('Ctrl Pts',(-53.6976396414809,-87.0324858381458,
60.5786142897588));
#209493=CARTESIAN_POINT('Ctrl Pts',(-53.5817591659509,-83.2313967727705,
59.8406133095025));
#209494=CARTESIAN_POINT('Ctrl Pts',(-53.4658786904209,-79.4440768967273,
60.6463003991196));
#209495=CARTESIAN_POINT('Ctrl Pts',(-53.3499982148909,-76.2725301145909,
62.8676095938363));
#209496=CARTESIAN_POINT('Ctrl Pts',(-53.2341177393609,-74.2208816676457,
66.1514582779195));
#209497=CARTESIAN_POINT('Ctrl Pts',(-53.1182372638309,-73.6152461742155,
69.9758705437336));
#209498=CARTESIAN_POINT('Ctrl Pts',(-53.0023567883009,-74.5518909007893,
73.7329465591992));
#209499=CARTESIAN_POINT('Ctrl Pts',(-52.8864763127809,-76.8819338408193,
76.8254897565407));
#209500=CARTESIAN_POINT('Ctrl Pts',(-52.7705958372509,-80.2350088795841,
78.761932710572));
#209501=CARTESIAN_POINT('Ctrl Pts',(-52.6547153617209,-84.0781364083665,
79.234473002314));
#209502=CARTESIAN_POINT('Ctrl Pts',(-52.5388348861909,-87.8004417575374,
78.167999178288));
#209503=CARTESIAN_POINT('Ctrl Pts',(-52.4229544106609,-90.8102552431185,
75.7320299026639));
#209504=CARTESIAN_POINT('Ctrl Pts',(-52.3070739351309,-92.6291595331741,
72.3137685443966));
#209505=CARTESIAN_POINT('Ctrl Pts',(-52.1911934596009,-92.9680352714057,
68.4565562396562));
#209506=CARTESIAN_POINT('Ctrl Pts',(-52.0753129840709,-91.7730173172237,
64.7735064682078));
#209507=CARTESIAN_POINT('Ctrl Pts',(-51.9594325085409,-89.2340567436806,
61.8500491424068));
#209508=CARTESIAN_POINT('Ctrl Pts',(-51.8435520330109,-85.7547276424399,
60.1508750680323));
#209509=CARTESIAN_POINT('Ctrl Pts',(-51.7276715574809,-81.8880780191402,
59.9460721861074));
#209510=CARTESIAN_POINT('Ctrl Pts',(-51.6117910819509,-78.2487214387897,
61.2681944235775));
#209511=CARTESIAN_POINT('Ctrl Pts',(-51.4959106064209,-75.4151426724483,
63.9070871657534));
#209512=CARTESIAN_POINT('Ctrl Pts',(-51.3800301308909,-73.837746105554,
67.443291854472));
#209513=CARTESIAN_POINT('Ctrl Pts',(-51.2641496553709,-73.7672628417323,
71.3147199681372));
#209514=CARTESIAN_POINT('Ctrl Pts',(-51.1482691798409,-75.2148963708959,
74.9059983888393));
#209515=CARTESIAN_POINT('Ctrl Pts',(-51.0323887043109,-77.9505417466829,
77.6462844884434));
#209516=CARTESIAN_POINT('Ctrl Pts',(-50.9165082287809,-81.5393613394195,
79.1000029826967));
#209517=CARTESIAN_POINT('Ctrl Pts',(-50.8006277532509,-85.4109033577874,
79.0360817049178));
#209518=CARTESIAN_POINT('Ctrl Pts',(-50.6847472777209,-88.9497765784368,
77.4646811010361));
#209519=CARTESIAN_POINT('Ctrl Pts',(-50.5688668021909,-91.5934683099975,
74.6355792014604));
#209520=CARTESIAN_POINT('Ctrl Pts',(-50.4529863266609,-92.9217571830265,
70.9984687825244));
#209521=CARTESIAN_POINT('Ctrl Pts',(-50.3371058511309,-92.7235083807798,
67.1314775823677));
#209522=CARTESIAN_POINT('Ctrl Pts',(-50.2212253756009,-91.0302340429712,
63.6492734604498));
#209523=CARTESIAN_POINT('Ctrl Pts',(-50.1053449000709,-88.1110843328011,
61.105361414176));
#209524=CARTESIAN_POINT('Ctrl Pts',(-49.9894644245409,-84.4300653499657,
59.9041025837992));
#209525=CARTESIAN_POINT('Ctrl Pts',(-49.8735839490209,-80.5722842074503,
60.2364400462553));
#209526=CARTESIAN_POINT('Ctrl Pts',(-49.7577034734909,-77.1509448049911,
62.0495479319753));
#209527=CARTESIAN_POINT('Ctrl Pts',(-49.6418229979609,-74.7098775347402,
65.055228253093));
#209528=CARTESIAN_POINT('Ctrl Pts',(-49.5259425224309,-73.6370961299356,
68.7757205963565));
#209529=CARTESIAN_POINT('Ctrl Pts',(-49.4100620469009,-74.1031217656728,
72.6196436763184));
#209530=CARTESIAN_POINT('Ctrl Pts',(-49.2941815713709,-76.0338788626926,
75.9759955596767));
#209531=CARTESIAN_POINT('Ctrl Pts',(-49.1783010958409,-79.1224674639693,
78.3112787937738));
#209532=CARTESIAN_POINT('Ctrl Pts',(-49.0624206203109,-82.8779536603277,
79.254283040401));
#209533=CARTESIAN_POINT('Ctrl Pts',(-48.9465401447809,-86.7033752162974,
78.6551574757721));
#209534=CARTESIAN_POINT('Ctrl Pts',(-48.8306596692509,-89.9907404410874,
76.6089776856617));
#209535=CARTESIAN_POINT('Ctrl Pts',(-48.7534060189009,-91.4750858508685,
74.4973756505227));
#209536=CARTESIAN_POINT('Ctrl Pts',(-48.7147791937209,-91.9816247835266,
73.3382509378444));
#209537=CARTESIAN_POINT('Ctrl Pts',(-55.9070015173239,-88.4387198218353,
76.9828771994399));
#209538=CARTESIAN_POINT('Ctrl Pts',(-55.8683746921479,-89.4328822235564,
76.2977664141032));
#209539=CARTESIAN_POINT('Ctrl Pts',(-55.7911210417949,-91.1420015977624,
74.5234739673153));
#209540=CARTESIAN_POINT('Ctrl Pts',(-55.6752405662649,-92.4624356766218,
71.0715732033575));
#209541=CARTESIAN_POINT('Ctrl Pts',(-55.5593600907359,-92.32923623476,67.3782446735901));
#209542=CARTESIAN_POINT('Ctrl Pts',(-55.4434796152059,-90.7637102347341,
64.0304593807184));
#209543=CARTESIAN_POINT('Ctrl Pts',(-55.3275991396769,-88.0146658633944,
61.5603809658357));
#209544=CARTESIAN_POINT('Ctrl Pts',(-55.2117186641469,-84.5190802164795,
60.3606278716294));
#209545=CARTESIAN_POINT('Ctrl Pts',(-55.0958381886179,-80.8325827289163,
60.6219056176175));
#209546=CARTESIAN_POINT('Ctrl Pts',(-54.9799577130879,-77.5411520298483,
62.3026829788096));
#209547=CARTESIAN_POINT('Ctrl Pts',(-54.8640772375589,-75.1679690211427,
65.135796345557));
#209548=CARTESIAN_POINT('Ctrl Pts',(-54.7481967620289,-74.0902570884328,
68.6709152745216));
#209549=CARTESIAN_POINT('Ctrl Pts',(-54.6323162864999,-74.4793212078432,
72.3461238375152));
#209550=CARTESIAN_POINT('Ctrl Pts',(-54.5164358109709,-76.2733186744711,
75.5772384992808));
#209551=CARTESIAN_POINT('Ctrl Pts',(-54.4005553354409,-79.1870891325353,
77.8506655567185));
#209552=CARTESIAN_POINT('Ctrl Pts',(-54.2846748599109,-82.7574815282069,
78.8050381301377));
#209553=CARTESIAN_POINT('Ctrl Pts',(-54.1687943843809,-86.416973118854,
78.2886563277362));
#209554=CARTESIAN_POINT('Ctrl Pts',(-54.0529139088509,-89.5838786235081,
76.3836003200345));
#209555=CARTESIAN_POINT('Ctrl Pts',(-53.9370334333209,-91.7548105434674,
73.3926834929055));
#209556=CARTESIAN_POINT('Ctrl Pts',(-53.8211529577909,-92.5846938559892,
69.7913195074835));
#209557=CARTESIAN_POINT('Ctrl Pts',(-53.7052724822609,-91.9416165465586,
66.1519541174746));
#209558=CARTESIAN_POINT('Ctrl Pts',(-53.5893920067309,-89.9277973513432,
63.053073494268));
#209559=CARTESIAN_POINT('Ctrl Pts',(-53.4735115312009,-86.8633378351191,
60.9872524126373));
#209560=CARTESIAN_POINT('Ctrl Pts',(-53.3576310556809,-83.2353414521743,
60.2828582664042));
#209561=CARTESIAN_POINT('Ctrl Pts',(-53.2417505801509,-79.6204872419811,
61.0518562553048));
#209562=CARTESIAN_POINT('Ctrl Pts',(-53.1258701046209,-76.5933652629879,
63.172012238292));
#209563=CARTESIAN_POINT('Ctrl Pts',(-53.0099896290909,-74.6351440751773,
66.306322153967));
#209564=CARTESIAN_POINT('Ctrl Pts',(-52.8941091535609,-74.0570878018971,
69.9565796534892));
#209565=CARTESIAN_POINT('Ctrl Pts',(-52.7782286780309,-74.9510799240673,
73.5425672375985));
#209566=CARTESIAN_POINT('Ctrl Pts',(-52.6623482025009,-77.1750181725883,
76.4942832697836));
#209567=CARTESIAN_POINT('Ctrl Pts',(-52.5464677269709,-80.3754020370897,
78.3425451526677));
#209568=CARTESIAN_POINT('Ctrl Pts',(-52.4305872514409,-84.0435225503917,
78.7935670676356));
#209569=CARTESIAN_POINT('Ctrl Pts',(-52.3147067759109,-87.5963228428119,
77.7756579606599));
#209570=CARTESIAN_POINT('Ctrl Pts',(-52.1988263003809,-90.4690764803083,
75.4506170134693));
#209571=CARTESIAN_POINT('Ctrl Pts',(-52.0829458248509,-92.2051521343437,
72.1880152615928));
#209572=CARTESIAN_POINT('Ctrl Pts',(-51.9670653493209,-92.5285962661224,
68.5064513600015));
#209573=CARTESIAN_POINT('Ctrl Pts',(-51.8511848737909,-91.3879966272414,
64.991119038349));
#209574=CARTESIAN_POINT('Ctrl Pts',(-51.7353043982609,-88.9646543643234,
62.2007891036226));
#209575=CARTESIAN_POINT('Ctrl Pts',(-51.6194239227409,-85.643765751282,
60.5789914320152));
#209576=CARTESIAN_POINT('Ctrl Pts',(-51.5035434472109,-81.9531942844895,
60.3835147930695));
#209577=CARTESIAN_POINT('Ctrl Pts',(-51.3876629716809,-78.479565468472,
61.6454306842398));
#209578=CARTESIAN_POINT('Ctrl Pts',(-51.2717824961509,-75.7750212343761,
64.164154439174));
#209579=CARTESIAN_POINT('Ctrl Pts',(-51.1559020206209,-74.2694556081259,
67.5393286588115));
#209580=CARTESIAN_POINT('Ctrl Pts',(-51.0400215450909,-74.2021819868569,
71.2344610147253));
#209581=CARTESIAN_POINT('Ctrl Pts',(-50.9241410695609,-75.5838936798222,
74.6622010377381));
#209582=CARTESIAN_POINT('Ctrl Pts',(-50.8082605940309,-78.1949641803186,
77.2777009343681));
#209583=CARTESIAN_POINT('Ctrl Pts',(-50.6923801185009,-81.6203573446273,
78.6652204973786));
#209584=CARTESIAN_POINT('Ctrl Pts',(-50.5764996429709,-85.3155984182905,
78.604210044692));
#209585=CARTESIAN_POINT('Ctrl Pts',(-50.4606191674409,-88.6933196511762,
77.1043673393538));
#209586=CARTESIAN_POINT('Ctrl Pts',(-50.3447386919109,-91.2166238607655,
74.4040961060068));
#209587=CARTESIAN_POINT('Ctrl Pts',(-50.2288582163809,-92.484425573369,
70.9326111664812));
#209588=CARTESIAN_POINT('Ctrl Pts',(-50.1129777408609,-92.2952045566739,
67.2417136774408));
#209589=CARTESIAN_POINT('Ctrl Pts',(-49.9970972653309,-90.6790379614674,
63.9180809654222));
#209590=CARTESIAN_POINT('Ctrl Pts',(-49.8812167898009,-87.8928194836539,
61.4900127082349));
#209591=CARTESIAN_POINT('Ctrl Pts',(-49.7653363142709,-84.3794254732619,
60.3434563880282));
#209592=CARTESIAN_POINT('Ctrl Pts',(-49.6494558387409,-80.6973186374278,
60.6606599817841));
#209593=CARTESIAN_POINT('Ctrl Pts',(-49.5335753632109,-77.4317790082792,
62.3912031861476));
#209594=CARTESIAN_POINT('Ctrl Pts',(-49.4176948876809,-75.1018722171853,
65.2600118737984));
#209595=CARTESIAN_POINT('Ctrl Pts',(-49.3018144121509,-74.0779427618718,
68.8110817203492));
#209596=CARTESIAN_POINT('Ctrl Pts',(-49.1859339366209,-74.5227466829941,
72.4799615572945));
#209597=CARTESIAN_POINT('Ctrl Pts',(-49.0700534610909,-76.365581629465,
75.6834730465697));
#209598=CARTESIAN_POINT('Ctrl Pts',(-48.9541729855609,-79.3135231486161,
77.912412958451));
#209599=CARTESIAN_POINT('Ctrl Pts',(-48.8382925100409,-82.8979933102528,
78.8124750030432));
#209600=CARTESIAN_POINT('Ctrl Pts',(-48.7224120345109,-86.5492141392223,
78.2406322116708));
#209601=CARTESIAN_POINT('Ctrl Pts',(-48.6065315589809,-89.686880460583,
76.2876306508874));
#209602=CARTESIAN_POINT('Ctrl Pts',(-48.5292779086209,-91.103632261208,
74.2721860206966));
#209603=CARTESIAN_POINT('Ctrl Pts',(-48.4906510834509,-91.5871045987178,
73.1658451292715));
#209604=CARTESIAN_POINT('Ctrl Pts',(-49.2716875596105,-89.6376853052957,
77.6221314644383));
#209605=CARTESIAN_POINT('Ctrl Pts',(-49.1710275888522,-89.5185411919897,
77.4698472271473));
#209606=CARTESIAN_POINT('Ctrl Pts',(-49.0703675024719,-89.3993929535507,
77.3175659292054));
#209607=CARTESIAN_POINT('Ctrl Pts',(-48.8698648872584,-89.1620562864648,
77.0142463336982));
#209608=CARTESIAN_POINT('Ctrl Pts',(-48.7700220939601,-89.0438676089703,
76.8632075858943));
#209609=CARTESIAN_POINT('Ctrl Pts',(-48.6701794005812,-88.9256751617442,
76.7121720277652));
#209610=CARTESIAN_POINT('Ctrl Pts',(-49.3172045433909,-89.3404582498078,
77.9029428178255));
#209611=CARTESIAN_POINT('Ctrl Pts',(-49.2671675200609,-90.8384471580197,
76.9294625104546));
#209612=CARTESIAN_POINT('Ctrl Pts',(-49.1670934734009,-93.3533237193631,
74.1587488145407));
#209613=CARTESIAN_POINT('Ctrl Pts',(-49.0169824034109,-94.5869930790562,
68.5383989146951));
#209614=CARTESIAN_POINT('Ctrl Pts',(-48.8668713334209,-92.8158926798989,
62.9167841918778));
#209615=CARTESIAN_POINT('Ctrl Pts',(-48.7667972867609,-89.8591099411729,
60.1918250007294));
#209616=CARTESIAN_POINT('Ctrl Pts',(-48.7167602634309,-88.1157743146814,
59.2817848695541));
#209617=CARTESIAN_POINT('Ctrl Pts',(-49.0930764331109,-89.0886145980675,
77.5537369843529));
#209618=CARTESIAN_POINT('Ctrl Pts',(-49.0430394097809,-90.5260811899022,
76.6239047484312));
#209619=CARTESIAN_POINT('Ctrl Pts',(-48.9429653631309,-92.9432122733185,
73.9726075199026));
#209620=CARTESIAN_POINT('Ctrl Pts',(-48.7928542931309,-94.1385843271853,
68.5806263247324));
#209621=CARTESIAN_POINT('Ctrl Pts',(-48.6427432231409,-92.4477415858012,
63.176215785295));
#209622=CARTESIAN_POINT('Ctrl Pts',(-48.5426691764809,-89.609279485427,
60.5503257501768));
#209623=CARTESIAN_POINT('Ctrl Pts',(-48.4926321531609,-87.9335507117994,
59.6718675500254));
#209624=CARTESIAN_POINT('Ctrl Pts',(-48.8689483228409,-88.8367709463283,
77.204531150883));
#209625=CARTESIAN_POINT('Ctrl Pts',(-48.8189112995109,-90.2137152217751,
76.3183469864107));
#209626=CARTESIAN_POINT('Ctrl Pts',(-48.7188372528509,-92.5331008272736,
73.7864662252636));
#209627=CARTESIAN_POINT('Ctrl Pts',(-48.5687261828609,-93.6901755753147,
68.6228537347706));
#209628=CARTESIAN_POINT('Ctrl Pts',(-48.4186151128609,-92.0795904917139,
63.4356473787111));
#209629=CARTESIAN_POINT('Ctrl Pts',(-48.3185410662109,-89.3594490296811,
60.9088264996243));
#209630=CARTESIAN_POINT('Ctrl Pts',(-48.2685040428809,-87.7513271089174,
60.0619502304968));
#209631=CARTESIAN_POINT('Ctrl Pts',(-48.6448202125609,-88.5849272945795,
76.855325317416));
#209632=CARTESIAN_POINT('Ctrl Pts',(-48.5947831892309,-89.9013492536484,
76.0127892243911));
#209633=CARTESIAN_POINT('Ctrl Pts',(-48.4947091425709,-92.1229893812291,
73.6003249306254));
#209634=CARTESIAN_POINT('Ctrl Pts',(-48.3445980725809,-93.2417668234437,
68.6650811448079));
#209635=CARTESIAN_POINT('Ctrl Pts',(-48.1944870025909,-91.7114393976162,
63.6950789721283));
#209636=CARTESIAN_POINT('Ctrl Pts',(-48.0944129559309,-89.1096185739352,
61.2673272490717));
#209637=CARTESIAN_POINT('Ctrl Pts',(-48.0443759326009,-87.5691035060354,
60.4520329109681));
#209638=CARTESIAN_POINT('Ctrl Pts',(-48.173560826516,-88.0240721664226,
60.4464459620599));
#209639=CARTESIAN_POINT('Ctrl Pts',(-48.1596729098132,-88.0118235639595,
60.4701459438197));
#209640=CARTESIAN_POINT('Ctrl Pts',(-48.1457849931372,-87.99957496149,60.4938459255919));
#209641=CARTESIAN_POINT('Ctrl Pts',(-48.1179938256803,-87.9750642324048,
60.5412720571842));
#209642=CARTESIAN_POINT('Ctrl Pts',(-48.1040905748995,-87.9628021057893,
60.5649982070044));
#209643=CARTESIAN_POINT('Ctrl Pts',(-48.0901873241469,-87.9505399791669,
60.5887243568376));
#209644=CARTESIAN_POINT('Origin',(-47.9901862140809,-88.4831990770459,59.5580752732411));
#209645=CARTESIAN_POINT('Ctrl Pts',(-47.890187490573,-87.9505401263848,
60.5887240719836));
#209646=CARTESIAN_POINT('Ctrl Pts',(-47.8762912240803,-87.9627960889656,
60.5650098490354));
#209647=CARTESIAN_POINT('Ctrl Pts',(-47.8623949575891,-87.9750520515467,
60.5412956260866));
#209648=CARTESIAN_POINT('Ctrl Pts',(-47.8346038364013,-87.9995627315646,
60.4938695894352));
#209649=CARTESIAN_POINT('Ctrl Pts',(-47.8207089817047,-88.0118174490013,
60.4701577757326));
#209650=CARTESIAN_POINT('Ctrl Pts',(-47.8068141270095,-88.0240721664383,
60.4464459620294));
#209651=CARTESIAN_POINT('Ctrl Pts',(-48.5133467647509,-88.5849272945888,
76.8553253174122));
#209652=CARTESIAN_POINT('Ctrl Pts',(-48.4633097414209,-89.9013492536481,
76.0127892243902));
#209653=CARTESIAN_POINT('Ctrl Pts',(-48.3632356947609,-92.1229893812287,
73.6003249306245));
#209654=CARTESIAN_POINT('Ctrl Pts',(-48.2131246247709,-93.2417668234433,
68.665081144807));
#209655=CARTESIAN_POINT('Ctrl Pts',(-48.0630135547809,-91.7114393976162,
63.6950789721283));
#209656=CARTESIAN_POINT('Ctrl Pts',(-47.9629395081209,-89.1096185739352,
61.2673272490717));
#209657=CARTESIAN_POINT('Ctrl Pts',(-47.9129024847909,-87.5691035060354,
60.4520329109681));
#209658=CARTESIAN_POINT('Ctrl Pts',(-48.2892186544709,-88.8367709463279,
77.2045311508821));
#209659=CARTESIAN_POINT('Ctrl Pts',(-48.2391816311409,-90.2137152217747,
76.3183469864098));
#209660=CARTESIAN_POINT('Ctrl Pts',(-48.1391075844909,-92.5331008272732,
73.7864662252626));
#209661=CARTESIAN_POINT('Ctrl Pts',(-47.9889965144909,-93.6901755753147,
68.6228537347706));
#209662=CARTESIAN_POINT('Ctrl Pts',(-47.8388854445009,-92.0795904917135,
63.4356473787102));
#209663=CARTESIAN_POINT('Ctrl Pts',(-47.7388113978409,-89.3594490296811,
60.9088264996243));
#209664=CARTESIAN_POINT('Ctrl Pts',(-47.6887743745209,-87.7513271089174,
60.0619502304968));
#209665=CARTESIAN_POINT('Ctrl Pts',(-48.0650905442009,-89.0886145980675,
77.5537369843529));
#209666=CARTESIAN_POINT('Ctrl Pts',(-48.0150535208709,-90.5260811899018,
76.6239047484302));
#209667=CARTESIAN_POINT('Ctrl Pts',(-47.9149794742109,-92.9432122733182,
73.9726075199017));
#209668=CARTESIAN_POINT('Ctrl Pts',(-47.7648684042209,-94.1385843271853,
68.5806263247324));
#209669=CARTESIAN_POINT('Ctrl Pts',(-47.6147573342209,-92.4477415858012,
63.176215785295));
#209670=CARTESIAN_POINT('Ctrl Pts',(-47.5146832875709,-89.609279485427,
60.5503257501768));
#209671=CARTESIAN_POINT('Ctrl Pts',(-47.4646462642409,-87.9335507117994,
59.6718675500254));
#209672=CARTESIAN_POINT('Ctrl Pts',(-47.8409624339209,-89.3404582498171,
77.9029428178217));
#209673=CARTESIAN_POINT('Ctrl Pts',(-47.7909254105909,-90.8384471580193,
76.9294625104536));
#209674=CARTESIAN_POINT('Ctrl Pts',(-47.6908513639309,-93.3533237193627,
74.1587488145398));
#209675=CARTESIAN_POINT('Ctrl Pts',(-47.5407402939409,-94.5869930790562,
68.5383989146951));
#209676=CARTESIAN_POINT('Ctrl Pts',(-47.3906292239509,-92.8158926798989,
62.9167841918778));
#209677=CARTESIAN_POINT('Ctrl Pts',(-47.2905551772909,-89.8591099411729,
60.1918250007294));
#209678=CARTESIAN_POINT('Ctrl Pts',(-47.2405181539609,-88.1157743146814,
59.2817848695541));
#209679=CARTESIAN_POINT('Ctrl Pts',(-48.4651187514177,-88.9258151777763,
76.7120624159033));
#209680=CARTESIAN_POINT('Ctrl Pts',(-48.3651833302526,-89.0441273831064,
76.8632423418457));
#209681=CARTESIAN_POINT('Ctrl Pts',(-48.2652478086818,-89.1624358230597,
77.0144254663974));
#209682=CARTESIAN_POINT('Ctrl Pts',(-48.064741788983,-89.3997965906428,
77.3177584516766));
#209683=CARTESIAN_POINT('Ctrl Pts',(-47.9641710688051,-89.5188491313808,
77.4699086873536));
#209684=CARTESIAN_POINT('Ctrl Pts',(-47.8636004674101,-89.637897562514,
77.6220618559046));
#209685=CARTESIAN_POINT('Ctrl Pts',(-55.7755280695129,-88.4387198218353,
76.9828771994399));
#209686=CARTESIAN_POINT('Ctrl Pts',(-55.7369012443359,-89.4328822235564,
76.2977664141032));
#209687=CARTESIAN_POINT('Ctrl Pts',(-55.6596475939829,-91.1420015977624,
74.5234739673153));
#209688=CARTESIAN_POINT('Ctrl Pts',(-55.5437671184529,-92.4624356766218,
71.0715732033575));
#209689=CARTESIAN_POINT('Ctrl Pts',(-55.4278866429239,-92.32923623476,67.3782446735901));
#209690=CARTESIAN_POINT('Ctrl Pts',(-55.3120061673939,-90.7637102347341,
64.0304593807184));
#209691=CARTESIAN_POINT('Ctrl Pts',(-55.1961256918649,-88.0146658633944,
61.5603809658357));
#209692=CARTESIAN_POINT('Ctrl Pts',(-55.0802452163349,-84.5190802164795,
60.3606278716294));
#209693=CARTESIAN_POINT('Ctrl Pts',(-54.9643647408059,-80.8325827289163,
60.6219056176175));
#209694=CARTESIAN_POINT('Ctrl Pts',(-54.8484842652759,-77.5411520298483,
62.3026829788096));
#209695=CARTESIAN_POINT('Ctrl Pts',(-54.7326037897459,-75.1679690211427,
65.135796345557));
#209696=CARTESIAN_POINT('Ctrl Pts',(-54.6167233142169,-74.0902570884328,
68.6709152745216));
#209697=CARTESIAN_POINT('Ctrl Pts',(-54.5008428386909,-74.4793212078431,
72.3461238375152));
#209698=CARTESIAN_POINT('Ctrl Pts',(-54.3849623631609,-76.2733186744711,
75.5772384992808));
#209699=CARTESIAN_POINT('Ctrl Pts',(-54.2690818876309,-79.1870891325353,
77.8506655567185));
#209700=CARTESIAN_POINT('Ctrl Pts',(-54.1532014121009,-82.7574815282069,
78.8050381301377));
#209701=CARTESIAN_POINT('Ctrl Pts',(-54.0373209365709,-86.416973118854,
78.2886563277362));
#209702=CARTESIAN_POINT('Ctrl Pts',(-53.9214404610409,-89.5838786235081,
76.3836003200345));
#209703=CARTESIAN_POINT('Ctrl Pts',(-53.8055599855109,-91.7548105434674,
73.3926834929055));
#209704=CARTESIAN_POINT('Ctrl Pts',(-53.6896795099809,-92.5846938559892,
69.7913195074835));
#209705=CARTESIAN_POINT('Ctrl Pts',(-53.5737990344509,-91.9416165465586,
66.1519541174746));
#209706=CARTESIAN_POINT('Ctrl Pts',(-53.4579185589209,-89.9277973513432,
63.053073494268));
#209707=CARTESIAN_POINT('Ctrl Pts',(-53.3420380833909,-86.8633378351191,
60.9872524126373));
#209708=CARTESIAN_POINT('Ctrl Pts',(-53.2261576078609,-83.2353414521743,
60.2828582664042));
#209709=CARTESIAN_POINT('Ctrl Pts',(-53.1102771323309,-79.6204872419811,
61.0518562553048));
#209710=CARTESIAN_POINT('Ctrl Pts',(-52.9943966568009,-76.5933652629879,
63.172012238292));
#209711=CARTESIAN_POINT('Ctrl Pts',(-52.8785161812709,-74.6351440751773,
66.306322153967));
#209712=CARTESIAN_POINT('Ctrl Pts',(-52.7626357057409,-74.0570878018971,
69.9565796534892));
#209713=CARTESIAN_POINT('Ctrl Pts',(-52.6467552302109,-74.9510799240673,
73.5425672375985));
#209714=CARTESIAN_POINT('Ctrl Pts',(-52.5308747546809,-77.1750181725883,
76.4942832697836));
#209715=CARTESIAN_POINT('Ctrl Pts',(-52.4149942791509,-80.3754020370897,
78.3425451526677));
#209716=CARTESIAN_POINT('Ctrl Pts',(-52.2991138036209,-84.0435225503917,
78.7935670676356));
#209717=CARTESIAN_POINT('Ctrl Pts',(-52.1832333281009,-87.5963228428119,
77.7756579606599));
#209718=CARTESIAN_POINT('Ctrl Pts',(-52.0673528525709,-90.4690764803083,
75.4506170134693));
#209719=CARTESIAN_POINT('Ctrl Pts',(-51.9514723770409,-92.2051521343437,
72.1880152615928));
#209720=CARTESIAN_POINT('Ctrl Pts',(-51.8355919015109,-92.5285962661224,
68.5064513600015));
#209721=CARTESIAN_POINT('Ctrl Pts',(-51.7197114259809,-91.3879966272414,
64.991119038349));
#209722=CARTESIAN_POINT('Ctrl Pts',(-51.6038309504509,-88.9646543643234,
62.2007891036226));
#209723=CARTESIAN_POINT('Ctrl Pts',(-51.4879504749209,-85.643765751282,
60.5789914320152));
#209724=CARTESIAN_POINT('Ctrl Pts',(-51.3720699993909,-81.9531942844895,
60.3835147930695));
#209725=CARTESIAN_POINT('Ctrl Pts',(-51.2561895238609,-78.479565468472,
61.6454306842398));
#209726=CARTESIAN_POINT('Ctrl Pts',(-51.1403090483309,-75.7750212343761,
64.164154439174));
#209727=CARTESIAN_POINT('Ctrl Pts',(-51.0244285728009,-74.2694556081259,
67.5393286588115));
#209728=CARTESIAN_POINT('Ctrl Pts',(-50.9085480972709,-74.2021819868569,
71.2344610147253));
#209729=CARTESIAN_POINT('Ctrl Pts',(-50.7926676217409,-75.5838936798222,
74.6622010377381));
#209730=CARTESIAN_POINT('Ctrl Pts',(-50.6767871462109,-78.1949641803186,
77.2777009343681));
#209731=CARTESIAN_POINT('Ctrl Pts',(-50.5609066706809,-81.6203573446273,
78.6652204973786));
#209732=CARTESIAN_POINT('Ctrl Pts',(-50.4450261951609,-85.3155984182905,
78.604210044692));
#209733=CARTESIAN_POINT('Ctrl Pts',(-50.3291457196309,-88.6933196511762,
77.1043673393538));
#209734=CARTESIAN_POINT('Ctrl Pts',(-50.2132652441009,-91.2166238607655,
74.4040961060068));
#209735=CARTESIAN_POINT('Ctrl Pts',(-50.0973847685709,-92.484425573369,
70.9326111664812));
#209736=CARTESIAN_POINT('Ctrl Pts',(-49.9815042930409,-92.2952045566739,
67.2417136774408));
#209737=CARTESIAN_POINT('Ctrl Pts',(-49.8656238175109,-90.6790379614674,
63.9180809654222));
#209738=CARTESIAN_POINT('Ctrl Pts',(-49.7497433419809,-87.8928194836539,
61.4900127082349));
#209739=CARTESIAN_POINT('Ctrl Pts',(-49.6338628664509,-84.3794254732619,
60.3434563880282));
#209740=CARTESIAN_POINT('Ctrl Pts',(-49.5179823909209,-80.6973186374278,
60.6606599817841));
#209741=CARTESIAN_POINT('Ctrl Pts',(-49.4021019153909,-77.4317790082792,
62.3912031861476));
#209742=CARTESIAN_POINT('Ctrl Pts',(-49.2862214398709,-75.1018722171853,
65.2600118737984));
#209743=CARTESIAN_POINT('Ctrl Pts',(-49.1703409643409,-74.0779427618718,
68.8110817203492));
#209744=CARTESIAN_POINT('Ctrl Pts',(-49.0544604888109,-74.5227466829941,
72.4799615572945));
#209745=CARTESIAN_POINT('Ctrl Pts',(-48.9385800132809,-76.365581629465,
75.6834730465697));
#209746=CARTESIAN_POINT('Ctrl Pts',(-48.8226995377509,-79.3135231486161,
77.912412958451));
#209747=CARTESIAN_POINT('Ctrl Pts',(-48.7068190622209,-82.8979933102528,
78.8124750030432));
#209748=CARTESIAN_POINT('Ctrl Pts',(-48.5909385866909,-86.5492141392223,
78.2406322116708));
#209749=CARTESIAN_POINT('Ctrl Pts',(-48.4750581111709,-89.686880460583,
76.2876306508874));
#209750=CARTESIAN_POINT('Ctrl Pts',(-48.3978044608109,-91.103632261208,
74.2721860206966));
#209751=CARTESIAN_POINT('Ctrl Pts',(-48.3591776356409,-91.5871045987178,
73.1658451292715));
#209752=CARTESIAN_POINT('Ctrl Pts',(-55.5513999592359,-88.6830297228196,
77.3373946338934));
#209753=CARTESIAN_POINT('Ctrl Pts',(-55.5127731340599,-89.7246238799117,
76.6195970288649));
#209754=CARTESIAN_POINT('Ctrl Pts',(-55.4355194837069,-91.5152857987813,
74.760652612607));
#209755=CARTESIAN_POINT('Ctrl Pts',(-55.3196390081769,-92.8987181423976,
71.1440607355203));
#209756=CARTESIAN_POINT('Ctrl Pts',(-55.2037585326479,-92.7591637193615,
67.274522509035));
#209757=CARTESIAN_POINT('Ctrl Pts',(-55.0878780571179,-91.1189460531508,
63.7670134801353));
#209758=CARTESIAN_POINT('Ctrl Pts',(-54.9719975815889,-88.2387440360669,
61.179086960254));
#209759=CARTESIAN_POINT('Ctrl Pts',(-54.8561171060589,-84.5763830585068,
59.9220933234976));
#209760=CARTESIAN_POINT('Ctrl Pts',(-54.7402366305299,-80.7140017850856,
60.1958367009625));
#209761=CARTESIAN_POINT('Ctrl Pts',(-54.6243561549999,-77.2655360428094,
61.9568044017577));
#209762=CARTESIAN_POINT('Ctrl Pts',(-54.5084756794709,-74.7791278349758,
64.9250863686191));
#209763=CARTESIAN_POINT('Ctrl Pts',(-54.3925952039409,-73.6499979763262,
68.6288667717323));
#209764=CARTESIAN_POINT('Ctrl Pts',(-54.2767147284109,-74.0576244494326,
72.4794205229618));
#209765=CARTESIAN_POINT('Ctrl Pts',(-54.1608342528809,-75.9372140173222,
75.8646925335888));
#209766=CARTESIAN_POINT('Ctrl Pts',(-54.0449537773509,-78.9900012470032,
78.2465854069093));
#209767=CARTESIAN_POINT('Ctrl Pts',(-53.9290733018209,-82.7307380233984,
79.2464913522906));
#209768=CARTESIAN_POINT('Ctrl Pts',(-53.8131928262909,-86.5648249413073,
78.7054728353225));
#209769=CARTESIAN_POINT('Ctrl Pts',(-53.6973123507609,-89.8828243586779,
76.7095260935192));
#209770=CARTESIAN_POINT('Ctrl Pts',(-53.5814318752309,-92.1573320239741,
73.5759118207695));
#209771=CARTESIAN_POINT('Ctrl Pts',(-53.4655513997009,-93.026809292365,
69.8027257917525));
#209772=CARTESIAN_POINT('Ctrl Pts',(-53.3496709241709,-92.353050591669,
65.9897253009272));
#209773=CARTESIAN_POINT('Ctrl Pts',(-53.2337904486409,-90.2431515414503,
62.7429962503755));
#209774=CARTESIAN_POINT('Ctrl Pts',(-53.1179099731109,-87.0324858381458,
60.5786142897588));
#209775=CARTESIAN_POINT('Ctrl Pts',(-53.0020294975809,-83.2313967727705,
59.8406133095025));
#209776=CARTESIAN_POINT('Ctrl Pts',(-52.8861490220609,-79.4440768967273,
60.6463003991196));
#209777=CARTESIAN_POINT('Ctrl Pts',(-52.7702685465309,-76.2725301145905,
62.8676095938354));
#209778=CARTESIAN_POINT('Ctrl Pts',(-52.6543880710009,-74.2208816676457,
66.1514582779195));
#209779=CARTESIAN_POINT('Ctrl Pts',(-52.5385075954709,-73.6152461742155,
69.9758705437336));
#209780=CARTESIAN_POINT('Ctrl Pts',(-52.4226271199409,-74.5518909007893,
73.7329465591992));
#209781=CARTESIAN_POINT('Ctrl Pts',(-52.3067466444109,-76.8819338408192,
76.8254897565408));
#209782=CARTESIAN_POINT('Ctrl Pts',(-52.1908661688809,-80.2350088795841,
78.761932710572));
#209783=CARTESIAN_POINT('Ctrl Pts',(-52.0749856933509,-84.0781364083665,
79.234473002314));
#209784=CARTESIAN_POINT('Ctrl Pts',(-51.9591052178209,-87.8004417575374,
78.167999178288));
#209785=CARTESIAN_POINT('Ctrl Pts',(-51.8432247422909,-90.8102552431185,
75.7320299026639));
#209786=CARTESIAN_POINT('Ctrl Pts',(-51.7273442667609,-92.6291595331741,
72.3137685443966));
#209787=CARTESIAN_POINT('Ctrl Pts',(-51.6114637912309,-92.9680352714057,
68.4565562396562));
#209788=CARTESIAN_POINT('Ctrl Pts',(-51.4955833157009,-91.7730173172237,
64.7735064682078));
#209789=CARTESIAN_POINT('Ctrl Pts',(-51.3797028401709,-89.2340567436806,
61.8500491424068));
#209790=CARTESIAN_POINT('Ctrl Pts',(-51.2638223646409,-85.7547276424399,
60.1508750680323));
#209791=CARTESIAN_POINT('Ctrl Pts',(-51.1479418891109,-81.8880780191402,
59.9460721861074));
#209792=CARTESIAN_POINT('Ctrl Pts',(-51.0320614135809,-78.2487214387897,
61.2681944235775));
#209793=CARTESIAN_POINT('Ctrl Pts',(-50.9161809380509,-75.4151426724483,
63.9070871657534));
#209794=CARTESIAN_POINT('Ctrl Pts',(-50.8003004625309,-73.837746105554,
67.443291854472));
#209795=CARTESIAN_POINT('Ctrl Pts',(-50.6844199870009,-73.7672628417323,
71.3147199681372));
#209796=CARTESIAN_POINT('Ctrl Pts',(-50.5685395114709,-75.2148963708959,
74.9059983888393));
#209797=CARTESIAN_POINT('Ctrl Pts',(-50.4526590359409,-77.9505417466828,
77.6462844884434));
#209798=CARTESIAN_POINT('Ctrl Pts',(-50.3367785604109,-81.5393613394195,
79.1000029826967));
#209799=CARTESIAN_POINT('Ctrl Pts',(-50.2208980848809,-85.4109033577874,
79.0360817049178));
#209800=CARTESIAN_POINT('Ctrl Pts',(-50.1050176093509,-88.9497765784368,
77.4646811010361));
#209801=CARTESIAN_POINT('Ctrl Pts',(-49.9891371338209,-91.5934683099975,
74.6355792014604));
#209802=CARTESIAN_POINT('Ctrl Pts',(-49.8732566582909,-92.9217571830265,
70.9984687825244));
#209803=CARTESIAN_POINT('Ctrl Pts',(-49.7573761827609,-92.7235083807798,
67.1314775823677));
#209804=CARTESIAN_POINT('Ctrl Pts',(-49.6414957072309,-91.0302340429712,
63.6492734604498));
#209805=CARTESIAN_POINT('Ctrl Pts',(-49.5256152317109,-88.1110843328011,
61.105361414176));
#209806=CARTESIAN_POINT('Ctrl Pts',(-49.4097347561809,-84.4300653499657,
59.9041025837992));
#209807=CARTESIAN_POINT('Ctrl Pts',(-49.2938542806509,-80.5722842074503,
60.2364400462553));
#209808=CARTESIAN_POINT('Ctrl Pts',(-49.1779738051209,-77.1509448049911,
62.0495479319753));
#209809=CARTESIAN_POINT('Ctrl Pts',(-49.0620933295909,-74.7098775347402,
65.055228253093));
#209810=CARTESIAN_POINT('Ctrl Pts',(-48.9462128540609,-73.6370961299356,
68.7757205963565));
#209811=CARTESIAN_POINT('Ctrl Pts',(-48.8303323785309,-74.1031217656727,
72.6196436763183));
#209812=CARTESIAN_POINT('Ctrl Pts',(-48.7144519030009,-76.033878862693,
75.9759955596776));
#209813=CARTESIAN_POINT('Ctrl Pts',(-48.5985714274709,-79.1224674639693,
78.3112787937738));
#209814=CARTESIAN_POINT('Ctrl Pts',(-48.4826909519509,-82.8779536603277,
79.254283040401));
#209815=CARTESIAN_POINT('Ctrl Pts',(-48.3668104764209,-86.7033752162974,
78.6551574757721));
#209816=CARTESIAN_POINT('Ctrl Pts',(-48.2509300008909,-89.9907404410874,
76.6089776856617));
#209817=CARTESIAN_POINT('Ctrl Pts',(-48.1736763505409,-91.4750858508685,
74.4973756505227));
#209818=CARTESIAN_POINT('Ctrl Pts',(-48.1350495253609,-91.9816247835266,
73.3382509378444));
#209819=CARTESIAN_POINT('Ctrl Pts',(-55.3272718489599,-88.9273396238135,
77.6919120683441));
#209820=CARTESIAN_POINT('Ctrl Pts',(-55.2886450237839,-90.0163655362671,
76.9414276436266));
#209821=CARTESIAN_POINT('Ctrl Pts',(-55.2113913734309,-91.8885699997907,
74.9978312579016));
#209822=CARTESIAN_POINT('Ctrl Pts',(-55.0955108979009,-93.335000608173,
71.2165482676822));
#209823=CARTESIAN_POINT('Ctrl Pts',(-54.9796304223719,-93.1890912039718,
67.1708003444751));
#209824=CARTESIAN_POINT('Ctrl Pts',(-54.8637499468419,-91.4741818715764,
63.5035675795474));
#209825=CARTESIAN_POINT('Ctrl Pts',(-54.7478694713129,-88.4628222087298,
60.7977929546752));
#209826=CARTESIAN_POINT('Ctrl Pts',(-54.6319889957829,-84.6336859005426,
59.4835587753601));
#209827=CARTESIAN_POINT('Ctrl Pts',(-54.5161085202509,-80.5954208412564,
59.7697677843112));
#209828=CARTESIAN_POINT('Ctrl Pts',(-54.4002280447209,-76.9899200557673,
61.6109258247081));
#209829=CARTESIAN_POINT('Ctrl Pts',(-54.2843475691909,-74.3902866488067,
64.7143763916865));
#209830=CARTESIAN_POINT('Ctrl Pts',(-54.1684670936609,-73.2097388642188,
68.58681826895));
#209831=CARTESIAN_POINT('Ctrl Pts',(-54.0525866181309,-73.6359276910248,
72.6127172084169));
#209832=CARTESIAN_POINT('Ctrl Pts',(-53.9367061426009,-75.6011093601795,
76.152146567904));
#209833=CARTESIAN_POINT('Ctrl Pts',(-53.8208256670709,-78.7929133614815,
78.6425052571067));
#209834=CARTESIAN_POINT('Ctrl Pts',(-53.7049451915509,-82.7039945186047,
79.687944574445));
#209835=CARTESIAN_POINT('Ctrl Pts',(-53.5890647160209,-86.7126767637781,
79.1222893429069));
#209836=CARTESIAN_POINT('Ctrl Pts',(-53.4731842404909,-90.1817700938727,
77.035451866986));
#209837=CARTESIAN_POINT('Ctrl Pts',(-53.3573037649609,-92.5598535044851,
73.7591401486176));
#209838=CARTESIAN_POINT('Ctrl Pts',(-53.2414232894309,-93.4689247287331,
69.8141320760029));
#209839=CARTESIAN_POINT('Ctrl Pts',(-53.1255428139009,-92.764484636779,
65.8274964843525));
#209840=CARTESIAN_POINT('Ctrl Pts',(-53.0096623383709,-90.5585057315378,
62.4329190064618));
#209841=CARTESIAN_POINT('Ctrl Pts',(-52.8937818628409,-87.2016338411459,
60.1699761668685));
#209842=CARTESIAN_POINT('Ctrl Pts',(-52.7779013873109,-83.2274520933251,
59.3983683526049));
#209843=CARTESIAN_POINT('Ctrl Pts',(-52.6620209117809,-79.2676665514421,
60.2407445429474));
#209844=CARTESIAN_POINT('Ctrl Pts',(-52.5461404362509,-75.9516949661677,
62.5632069494066));
#209845=CARTESIAN_POINT('Ctrl Pts',(-52.4302599607209,-73.8066192600998,
65.9965944019082));
#209846=CARTESIAN_POINT('Ctrl Pts',(-52.3143794851909,-73.1734045465354,
69.9951614340195));
#209847=CARTESIAN_POINT('Ctrl Pts',(-52.1984990096609,-74.15270187753,73.9233258808396));
#209848=CARTESIAN_POINT('Ctrl Pts',(-52.0826185341309,-76.5888495090847,
77.1566962433291));
#209849=CARTESIAN_POINT('Ctrl Pts',(-51.9667380586009,-80.0946157221245,
79.1813202684909));
#209850=CARTESIAN_POINT('Ctrl Pts',(-51.8508575830709,-84.1127502663909,
79.6753789369893));
#209851=CARTESIAN_POINT('Ctrl Pts',(-51.7349771075409,-88.0045606723086,
78.5603403958907));
#209852=CARTESIAN_POINT('Ctrl Pts',(-51.6190966320109,-91.1514340059658,
76.0134427918171));
#209853=CARTESIAN_POINT('Ctrl Pts',(-51.5032161564809,-93.053166932025,
72.4395218271453));
#209854=CARTESIAN_POINT('Ctrl Pts',(-51.3873356809509,-93.4074742766868,
68.4066611192533));
#209855=CARTESIAN_POINT('Ctrl Pts',(-51.2714552054309,-92.1580380071747,
64.5558938980169));
#209856=CARTESIAN_POINT('Ctrl Pts',(-51.1555747299009,-89.5034591229898,
61.4993091811534));
#209857=CARTESIAN_POINT('Ctrl Pts',(-51.0396942543709,-85.8656895335373,
59.7227587040344));
#209858=CARTESIAN_POINT('Ctrl Pts',(-50.9238137788409,-81.8229617537302,
59.5086295791554));
#209859=CARTESIAN_POINT('Ctrl Pts',(-50.8079333033109,-78.0178774090514,
60.8909581629449));
#209860=CARTESIAN_POINT('Ctrl Pts',(-50.6920528277809,-75.0552641104844,
63.6500198923845));
#209861=CARTESIAN_POINT('Ctrl Pts',(-50.5761723522509,-73.4060366029682,
67.3472550501956));
#209862=CARTESIAN_POINT('Ctrl Pts',(-50.4602918767209,-73.3323436966194,
71.3949789216125));
#209863=CARTESIAN_POINT('Ctrl Pts',(-50.3444114011909,-74.8458990620047,
75.1497957399931));
#209864=CARTESIAN_POINT('Ctrl Pts',(-50.2285309256609,-77.7061193131001,
78.0148680425531));
#209865=CARTESIAN_POINT('Ctrl Pts',(-50.1126504501309,-81.4583653342733,
79.534785468025));
#209866=CARTESIAN_POINT('Ctrl Pts',(-49.9967699746009,-85.5062082973436,
79.4679533651301));
#209867=CARTESIAN_POINT('Ctrl Pts',(-49.8808894990709,-89.206233505757,
77.8249948626797));
#209868=CARTESIAN_POINT('Ctrl Pts',(-49.7650090235509,-91.9703127592713,
74.8670622968578));
#209869=CARTESIAN_POINT('Ctrl Pts',(-49.6491285480209,-93.3590887926927,
71.06432639851));
#209870=CARTESIAN_POINT('Ctrl Pts',(-49.5332480724909,-93.1518122048732,
67.0212414872382));
#209871=CARTESIAN_POINT('Ctrl Pts',(-49.4173675969609,-91.3814301244552,
63.3804659554293));
#209872=CARTESIAN_POINT('Ctrl Pts',(-49.3014871214309,-88.3293491819053,
60.7207101200916));
#209873=CARTESIAN_POINT('Ctrl Pts',(-49.1856066459009,-84.4807052266326,
59.4647487795594));
#209874=CARTESIAN_POINT('Ctrl Pts',(-49.0697261703709,-80.447249777423,
59.8122201107395));
#209875=CARTESIAN_POINT('Ctrl Pts',(-48.9538456948409,-76.8701106016706,
61.7078926778295));
#209876=CARTESIAN_POINT('Ctrl Pts',(-48.8379652193109,-74.3178828522775,
64.8504446324207));
#209877=CARTESIAN_POINT('Ctrl Pts',(-48.7220847437809,-73.1962494979973,
68.7403594723971));
#209878=CARTESIAN_POINT('Ctrl Pts',(-48.6062042682609,-73.6834968483605,
72.7593257953694));
#209879=CARTESIAN_POINT('Ctrl Pts',(-48.4903237927309,-75.7021760959367,
76.2685180728017));
#209880=CARTESIAN_POINT('Ctrl Pts',(-48.3744433172009,-78.9314117793381,
78.710144629103));
#209881=CARTESIAN_POINT('Ctrl Pts',(-48.2585628416709,-82.8579140104155,
79.6960910777588));
#209882=CARTESIAN_POINT('Ctrl Pts',(-48.1426823661409,-86.8575362933791,
79.0696827398739));
#209883=CARTESIAN_POINT('Ctrl Pts',(-48.0268018906109,-90.2946004215829,
76.9303247204407));
#209884=CARTESIAN_POINT('Ctrl Pts',(-47.9495482402609,-91.8465394405205,
74.7225652803544));
#209885=CARTESIAN_POINT('Ctrl Pts',(-47.9109214150809,-92.3761449683377,
73.5106567464228));
#209886=CARTESIAN_POINT('Ctrl Pts',(-55.1031437386839,-89.1716495247985,
78.0464295027995));
#209887=CARTESIAN_POINT('Ctrl Pts',(-55.0645169135079,-90.3081071926132,
77.2632582583921));
#209888=CARTESIAN_POINT('Ctrl Pts',(-54.9872632631549,-92.2618542008096,
75.2350099031932));
#209889=CARTESIAN_POINT('Ctrl Pts',(-54.8713827876249,-93.7712830739489,
71.289035799845));
#209890=CARTESIAN_POINT('Ctrl Pts',(-54.7555023120959,-93.6190186885821,
67.0670781799152));
#209891=CARTESIAN_POINT('Ctrl Pts',(-54.6396218365659,-91.8294176899935,
63.2401216789652));
#209892=CARTESIAN_POINT('Ctrl Pts',(-54.5237413610409,-88.686900381402,
60.4164989490926));
#209893=CARTESIAN_POINT('Ctrl Pts',(-54.4078608855109,-84.6909887425699,
59.0450242272283));
#209894=CARTESIAN_POINT('Ctrl Pts',(-54.2919804099809,-80.4768398974234,
59.3436988676507));
#209895=CARTESIAN_POINT('Ctrl Pts',(-54.1760999344509,-76.7143040687269,
61.2650472476524));
#209896=CARTESIAN_POINT('Ctrl Pts',(-54.0602194589209,-74.0014454626398,
64.5036664147486));
#209897=CARTESIAN_POINT('Ctrl Pts',(-53.9443389833909,-72.7694797521119,
68.5447697661598));
#209898=CARTESIAN_POINT('Ctrl Pts',(-53.8284585078609,-73.2142309326136,
72.746013893864));
#209899=CARTESIAN_POINT('Ctrl Pts',(-53.7125780323309,-75.2650047030302,
76.4396006022121));
#209900=CARTESIAN_POINT('Ctrl Pts',(-53.5966975568009,-78.5958254759494,
79.0384251072975));
#209901=CARTESIAN_POINT('Ctrl Pts',(-53.4808170812709,-82.6772510137972,
80.1293977965975));
#209902=CARTESIAN_POINT('Ctrl Pts',(-53.3649366057409,-86.8605285862284,
79.5391058504835));
#209903=CARTESIAN_POINT('Ctrl Pts',(-53.2490561302109,-90.4807158290425,
77.3613776404707));
#209904=CARTESIAN_POINT('Ctrl Pts',(-53.1331756546809,-92.9623749849825,
73.9423684764853));
#209905=CARTESIAN_POINT('Ctrl Pts',(-53.0172951791509,-93.9110401651089,
69.8255383602718));
#209906=CARTESIAN_POINT('Ctrl Pts',(-52.9014147036209,-93.1759186818892,
65.6652676678046));
#209907=CARTESIAN_POINT('Ctrl Pts',(-52.7855342280909,-90.8738599216446,
62.1228417625684));
#209908=CARTESIAN_POINT('Ctrl Pts',(-52.6696537525609,-87.3707818441818,
59.7613380439862));
#209909=CARTESIAN_POINT('Ctrl Pts',(-52.5537732770309,-83.2235074139119,
58.956123395707));
#209910=CARTESIAN_POINT('Ctrl Pts',(-52.4378928015009,-79.0912562061879,
59.8351886867613));
#209911=CARTESIAN_POINT('Ctrl Pts',(-52.3220123259709,-75.6308598177706,
62.258804304951));
#209912=CARTESIAN_POINT('Ctrl Pts',(-52.2061318504409,-73.3923568525672,
65.8417305258611));
#209913=CARTESIAN_POINT('Ctrl Pts',(-52.0902513749109,-72.7315629188536,
70.0144523242639));
#209914=CARTESIAN_POINT('Ctrl Pts',(-51.9743708993809,-73.7535128542524,
74.113705202441));
#209915=CARTESIAN_POINT('Ctrl Pts',(-51.8584904238609,-76.2957651773164,
77.487902730087));
#209916=CARTESIAN_POINT('Ctrl Pts',(-51.7426099483309,-79.9542225646198,
79.6007078263948));
#209917=CARTESIAN_POINT('Ctrl Pts',(-51.6267294728009,-84.1473641243655,
80.1162848716646));
#209918=CARTESIAN_POINT('Ctrl Pts',(-51.5108489972709,-88.2086795870379,
78.9526816135227));
#209919=CARTESIAN_POINT('Ctrl Pts',(-51.3949685217409,-91.4926127687853,
76.2948556810079));
#209920=CARTESIAN_POINT('Ctrl Pts',(-51.2790880462109,-93.477174330855,
72.5652751099481));
#209921=CARTESIAN_POINT('Ctrl Pts',(-51.1632075706809,-93.84691328197,68.3567659989079));
#209922=CARTESIAN_POINT('Ctrl Pts',(-51.0473270951509,-92.5430586971659,
64.338281327871));
#209923=CARTESIAN_POINT('Ctrl Pts',(-50.9314466196209,-89.7728615023466,
61.1485692199366));
#209924=CARTESIAN_POINT('Ctrl Pts',(-50.8155661440909,-85.9766514246951,
59.2946423400516));
#209925=CARTESIAN_POINT('Ctrl Pts',(-50.6996856685609,-81.7578454883824,
59.0711869721971));
#209926=CARTESIAN_POINT('Ctrl Pts',(-50.5838051930309,-77.7870333793684,
60.5137219022862));
#209927=CARTESIAN_POINT('Ctrl Pts',(-50.4679247175009,-74.6953855485565,
63.3929526189662));
#209928=CARTESIAN_POINT('Ctrl Pts',(-50.3520442419709,-72.9743271003957,
67.2512182458574));
#209929=CARTESIAN_POINT('Ctrl Pts',(-50.2361637664409,-72.8974245514948,
71.4752378750255));
#209930=CARTESIAN_POINT('Ctrl Pts',(-50.1202832909109,-74.4769017530788,
75.3935930910951));
#209931=CARTESIAN_POINT('Ctrl Pts',(-50.0044028153909,-77.4616968794652,
78.383451596628));
#209932=CARTESIAN_POINT('Ctrl Pts',(-49.8885223398609,-81.3773693290668,
79.9695679533435));
#209933=CARTESIAN_POINT('Ctrl Pts',(-49.7726418643309,-85.6015132368418,
79.8998250253565));
#209934=CARTESIAN_POINT('Ctrl Pts',(-49.6567613888009,-89.462690433018,
78.1853086243629));
#209935=CARTESIAN_POINT('Ctrl Pts',(-49.5408809132709,-92.3471572085029,
75.0985453923105));
#209936=CARTESIAN_POINT('Ctrl Pts',(-49.4250004377409,-93.7964204023591,
71.1301840145485));
#209937=CARTESIAN_POINT('Ctrl Pts',(-49.3091199622109,-93.5801160289695,
66.9110053921681));
#209938=CARTESIAN_POINT('Ctrl Pts',(-49.1932394866809,-91.7326262059582,
63.111658450455));
#209939=CARTESIAN_POINT('Ctrl Pts',(-49.0773590111509,-88.5476140310613,
60.3360588260279));
#209940=CARTESIAN_POINT('Ctrl Pts',(-48.9614785356209,-84.5313451033357,
59.0253949753285));
#209941=CARTESIAN_POINT('Ctrl Pts',(-48.8455980601009,-80.3222153474369,
59.3880001752185));
#209942=CARTESIAN_POINT('Ctrl Pts',(-48.7297175845709,-76.5892763983811,
61.3662374236589));
#209943=CARTESIAN_POINT('Ctrl Pts',(-48.6138371090409,-73.9258881698316,
64.6456610117156));
#209944=CARTESIAN_POINT('Ctrl Pts',(-48.4979566335109,-72.7554028660613,
68.7049983484054));
#209945=CARTESIAN_POINT('Ctrl Pts',(-48.3820761579809,-73.2638719310397,
72.8990079143937));
#209946=CARTESIAN_POINT('Ctrl Pts',(-48.2661956824509,-75.3704733291652,
76.5610405859094));
#209947=CARTESIAN_POINT('Ctrl Pts',(-48.1503152069209,-78.7403560946919,
79.1090104644245));
#209948=CARTESIAN_POINT('Ctrl Pts',(-48.0344347313909,-82.8378743604903,
80.1378991151166));
#209949=CARTESIAN_POINT('Ctrl Pts',(-47.9185542558709,-87.0116973704533,
79.4842080039733));
#209950=CARTESIAN_POINT('Ctrl Pts',(-47.8026737803409,-90.5984604020873,
77.251671755215));
#209951=CARTESIAN_POINT('Ctrl Pts',(-47.7254201299809,-92.2179930301717,
74.9477549101844));
#209952=CARTESIAN_POINT('Ctrl Pts',(-47.6867933048109,-92.7706651531469,
73.6830625549966));
#209953=CARTESIAN_POINT('',(-55.5975553638665,-91.4098880899276,73.6973239050991));
#209954=CARTESIAN_POINT('Ctrl Pts',(-62.9066342559309,-91.0821450451938,
74.1516175606607));
#209955=CARTESIAN_POINT('Ctrl Pts',(-62.8680074307549,-91.6975062893363,
73.1128364439599));
#209956=CARTESIAN_POINT('Ctrl Pts',(-62.7907537804019,-92.5053451055553,
70.7854776041952));
#209957=CARTESIAN_POINT('Ctrl Pts',(-62.6748733048729,-92.2570005774417,
67.098000141731));
#209958=CARTESIAN_POINT('Ctrl Pts',(-62.5589928293429,-90.5877173901553,
63.8007419836912));
#209959=CARTESIAN_POINT('Ctrl Pts',(-62.4431123538139,-87.7629155557435,
61.4176698865353));
#209960=CARTESIAN_POINT('Ctrl Pts',(-62.3272318782849,-84.2315820238582,
60.3276167603847));
#209961=CARTESIAN_POINT('Ctrl Pts',(-62.2113514027559,-80.5550370144063,
60.7038391619823));
#209962=CARTESIAN_POINT('Ctrl Pts',(-62.0954709272259,-77.3176748891168,
62.4865383110414));
#209963=CARTESIAN_POINT('Ctrl Pts',(-61.9795904516969,-75.0340828310024,
65.3923490235231));
#209964=CARTESIAN_POINT('Ctrl Pts',(-61.8637099761679,-74.0672433566291,
68.9593856609049));
#209965=CARTESIAN_POINT('Ctrl Pts',(-61.7478295006379,-74.570838033561,
72.620658834703));
#209966=CARTESIAN_POINT('Ctrl Pts',(-61.6319490251089,-76.4648192283687,
75.7942000908074));
#209967=CARTESIAN_POINT('Ctrl Pts',(-61.5160685495799,-79.4481339264209,
77.9755671576036));
#209968=CARTESIAN_POINT('Ctrl Pts',(-61.4001880740499,-83.0465768432993,
78.8180263208338));
#209969=CARTESIAN_POINT('Ctrl Pts',(-61.2843075985209,-86.6881665365578,
78.1876666029972));
#209970=CARTESIAN_POINT('Ctrl Pts',(-61.1684271229909,-89.7940632762463,
76.1846852475528));
#209971=CARTESIAN_POINT('Ctrl Pts',(-61.0525466474619,-91.8705770584431,
73.1274611176964));
#209972=CARTESIAN_POINT('Ctrl Pts',(-60.9366661719329,-92.5876408580107,
69.5019475850796));
#209973=CARTESIAN_POINT('Ctrl Pts',(-60.8207856964029,-91.8312756023416,
65.8844290339351));
#209974=CARTESIAN_POINT('Ctrl Pts',(-60.7049052208739,-89.7217074281312,
62.8499190263368));
#209975=CARTESIAN_POINT('Ctrl Pts',(-60.5890247453439,-86.5942574382841,
60.8807604677571));
#209976=CARTESIAN_POINT('Ctrl Pts',(-60.4731442698149,-82.9460415793733,
60.2899560038079));
#209977=CARTESIAN_POINT('Ctrl Pts',(-60.3572637942849,-79.3569528268042,
61.1714154719932));
#209978=CARTESIAN_POINT('Ctrl Pts',(-60.2413833187559,-76.3974857555292,
63.3850286996998));
#209979=CARTESIAN_POINT('Ctrl Pts',(-60.1255028432259,-74.5380550098396,
66.578936364274));
#209980=CARTESIAN_POINT('Ctrl Pts',(-60.0096223676969,-74.0742217268447,
70.2454589066055));
#209981=CARTESIAN_POINT('Ctrl Pts',(-59.8937418921669,-75.0797133593528,
73.8017934584711));
#209982=CARTESIAN_POINT('Ctrl Pts',(-59.7778614166379,-77.3947045140553,
76.682651806513));
#209983=CARTESIAN_POINT('Ctrl Pts',(-59.6619809411079,-80.65122159491,78.430114358312));
#209984=CARTESIAN_POINT('Ctrl Pts',(-59.5461004655789,-84.3316331205256,
78.7664175993805));
#209985=CARTESIAN_POINT('Ctrl Pts',(-59.4302199900499,-87.850928534276,
77.6381052939461));
#209986=CARTESIAN_POINT('Ctrl Pts',(-59.3143395145199,-90.6497070858334,
75.2245254864509));
#209987=CARTESIAN_POINT('Ctrl Pts',(-59.1984590389909,-92.283095970383,
71.9093226842531));
#209988=CARTESIAN_POINT('Ctrl Pts',(-59.0825785634609,-92.4914639662642,
68.2194566099759));
#209989=CARTESIAN_POINT('Ctrl Pts',(-58.9666980879319,-91.2416904628249,
64.7414406442362));
#209990=CARTESIAN_POINT('Ctrl Pts',(-58.8508176124019,-88.7324300637027,
62.0281140665388));
#209991=CARTESIAN_POINT('Ctrl Pts',(-58.7349371368729,-85.3625359440494,
60.5107668781401));
#209992=CARTESIAN_POINT('Ctrl Pts',(-58.6190566613429,-81.6676611472649,
60.4305851847562));
#209993=CARTESIAN_POINT('Ctrl Pts',(-58.5031761858139,-78.2351152028786,
61.8003140657713));
#209994=CARTESIAN_POINT('Ctrl Pts',(-58.3872957102849,-75.6105098175054,
64.4022317122195));
#209995=CARTESIAN_POINT('Ctrl Pts',(-58.2714152347549,-74.2110325384453,
67.822756849275));
#209996=CARTESIAN_POINT('Ctrl Pts',(-58.1555347592259,-74.259133756452,
71.5181885075058));
#209997=CARTESIAN_POINT('Ctrl Pts',(-58.0396542836959,-75.7471676634089,
74.901128642888));
#209998=CARTESIAN_POINT('Ctrl Pts',(-57.9237738081669,-78.4386075725234,
77.4338505153925));
#209999=CARTESIAN_POINT('Ctrl Pts',(-57.8078933326379,-81.9056424228852,
78.7137716903922));
#210000=CARTESIAN_POINT('Ctrl Pts',(-57.6920128571079,-85.5971784105718,
78.5374455169307));
#210001=CARTESIAN_POINT('Ctrl Pts',(-57.5761323815789,-88.9264367180665,
76.9328994783958));
#210002=CARTESIAN_POINT('Ctrl Pts',(-57.4602519060499,-91.3642234652816,
74.1551801543822));
#210003=CARTESIAN_POINT('Ctrl Pts',(-57.3443714305209,-92.523046391615,
70.6458129331831));
#210004=CARTESIAN_POINT('Ctrl Pts',(-57.2284909549909,-92.2187077136396,
66.9626204542406));
#210005=CARTESIAN_POINT('Ctrl Pts',(-57.1126104794619,-90.4995828203968,
63.6910553136321));
#210006=CARTESIAN_POINT('Ctrl Pts',(-56.9967300039329,-87.6389308851381,
61.3511409192107));
#210007=CARTESIAN_POINT('Ctrl Pts',(-56.8808495284039,-84.091459640771,
60.3148124779814));
#210008=CARTESIAN_POINT('Ctrl Pts',(-56.7649690528749,-80.4210484558933,
60.7467969703094));
#210009=CARTESIAN_POINT('Ctrl Pts',(-56.6490885773459,-77.2111183081457,
62.57842938896));
#210010=CARTESIAN_POINT('Ctrl Pts',(-56.5332081018169,-74.9718955700618,
65.5185672056337));
#210011=CARTESIAN_POINT('Ctrl Pts',(-56.4173276262869,-74.0593102599364,
69.0998682252855));
#210012=CARTESIAN_POINT('Ctrl Pts',(-56.3014471507579,-74.6184200790472,
72.7530756919932));
#210013=CARTESIAN_POINT('Ctrl Pts',(-56.1855666752289,-76.560353137091,
75.8975034275876));
#210014=CARTESIAN_POINT('Ctrl Pts',(-56.0696861997009,-79.5764343320587,
78.0333359882835));
#210015=CARTESIAN_POINT('Ctrl Pts',(-55.9538057241719,-83.18725012881,78.8210806253173));
#210016=CARTESIAN_POINT('Ctrl Pts',(-55.8379252486429,-86.8188521429654,
78.1355116392279));
#210017=CARTESIAN_POINT('Ctrl Pts',(-55.7220447731139,-89.8939891133529,
76.0856457086153));
#210018=CARTESIAN_POINT('Ctrl Pts',(-55.6061642975849,-91.9238570102634,
72.9971507091326));
#210019=CARTESIAN_POINT('Ctrl Pts',(-55.5289106472319,-92.3651629072477,
70.5734238624515));
#210020=CARTESIAN_POINT('Ctrl Pts',(-55.4902838220559,-92.3402865293407,
69.3663129168427));
#210021=CARTESIAN_POINT('Ctrl Pts',(-62.6825061456549,-91.452573473999,
74.371054836858));
#210022=CARTESIAN_POINT('Ctrl Pts',(-62.6438793204789,-92.0972937684766,
73.282713193911));
#210023=CARTESIAN_POINT('Ctrl Pts',(-62.5666256701259,-92.9436747917172,
70.8443154384341));
#210024=CARTESIAN_POINT('Ctrl Pts',(-62.4507451945969,-92.6834816794201,
66.9809074352464));
#210025=CARTESIAN_POINT('Ctrl Pts',(-62.3348647190669,-90.9345565426601,
63.5263362043601));
#210026=CARTESIAN_POINT('Ctrl Pts',(-62.2189842435379,-87.9749826535781,
61.0295670970088));
#210027=CARTESIAN_POINT('Ctrl Pts',(-62.1031037680089,-84.2751682498535,
59.8875072432627));
#210028=CARTESIAN_POINT('Ctrl Pts',(-61.9872232924799,-80.4232142899493,
60.2816793167476));
#210029=CARTESIAN_POINT('Ctrl Pts',(-61.8713428169499,-77.0313967476354,
62.1494315213011));
#210030=CARTESIAN_POINT('Ctrl Pts',(-61.7554623414209,-74.6388538987226,
65.1938792437981));
#210031=CARTESIAN_POINT('Ctrl Pts',(-61.6395818658919,-73.6258862531933,
68.9311001577751));
#210032=CARTESIAN_POINT('Ctrl Pts',(-61.5237013903619,-74.1535075675003,
72.7670536586458));
#210033=CARTESIAN_POINT('Ctrl Pts',(-61.4078209148329,-76.137851114111,
76.0920054209541));
#210034=CARTESIAN_POINT('Ctrl Pts',(-61.2919404393039,-79.26350055816,78.3774460967395));
#210035=CARTESIAN_POINT('Ctrl Pts',(-61.1760599637739,-83.0336261536677,
79.2600992130555));
#210036=CARTESIAN_POINT('Ctrl Pts',(-61.0601794882449,-86.8489570698533,
78.5996648636749));
#210037=CARTESIAN_POINT('Ctrl Pts',(-60.9442990127149,-90.1030369776855,
76.5011207294713));
#210038=CARTESIAN_POINT('Ctrl Pts',(-60.8284185371859,-92.2786217904858,
73.2980356147633));
#210039=CARTESIAN_POINT('Ctrl Pts',(-60.7125380616569,-93.0298968966431,
69.4995478571636));
#210040=CARTESIAN_POINT('Ctrl Pts',(-60.5966575861269,-92.2374452513553,
65.7094365237526));
#210041=CARTESIAN_POINT('Ctrl Pts',(-60.4807771105979,-90.0272290126208,
62.5301492281794));
#210042=CARTESIAN_POINT('Ctrl Pts',(-60.3648966350679,-86.7505675432666,
60.4670415855671));
#210043=CARTESIAN_POINT('Ctrl Pts',(-60.2490161595389,-82.9282943252811,
59.8480496818692));
#210044=CARTESIAN_POINT('Ctrl Pts',(-60.1331356840089,-79.1679691837779,
60.7715638181681));
#210045=CARTESIAN_POINT('Ctrl Pts',(-60.0172552084799,-76.0673051431882,
63.0907891278659));
#210046=CARTESIAN_POINT('Ctrl Pts',(-59.9013747329499,-74.1191604569068,
66.4370789854654));
#210047=CARTESIAN_POINT('Ctrl Pts',(-59.7854942574209,-73.6331975633271,
70.2785323036529));
#210048=CARTESIAN_POINT('Ctrl Pts',(-59.6696137818909,-74.6866614718425,
74.004540532737));
#210049=CARTESIAN_POINT('Ctrl Pts',(-59.5537333063619,-77.112101476679,
77.0228454067829));
#210050=CARTESIAN_POINT('Ctrl Pts',(-59.4378528308319,-80.5239878626353,
78.8536798665507));
#210051=CARTESIAN_POINT('Ctrl Pts',(-59.3219723553029,-84.3799928112316,
79.2060282256322));
#210052=CARTESIAN_POINT('Ctrl Pts',(-59.2060918797729,-88.0671947549688,
78.0238838368779));
#210053=CARTESIAN_POINT('Ctrl Pts',(-59.0902114042439,-90.9995037833793,
75.4951514881295));
#210054=CARTESIAN_POINT('Ctrl Pts',(-58.9743309287149,-92.7108220905774,
72.0217794692934));
#210055=CARTESIAN_POINT('Ctrl Pts',(-58.8584504531849,-92.9291313795479,
68.1558688929745));
#210056=CARTESIAN_POINT('Ctrl Pts',(-58.7425699776559,-91.6197308463801,
64.5119158508118));
#210057=CARTESIAN_POINT('Ctrl Pts',(-58.6266895021259,-88.9907529592742,
61.6691357328928));
#210058=CARTESIAN_POINT('Ctrl Pts',(-58.5108090265969,-85.4600802855175,
60.079395502359));
#210059=CARTESIAN_POINT('Ctrl Pts',(-58.3949285510669,-81.5889220192099,
59.9953883188284));
#210060=CARTESIAN_POINT('Ctrl Pts',(-58.2790480755379,-77.9926083853276,
61.4304673328671));
#210061=CARTESIAN_POINT('Ctrl Pts',(-58.1631676000089,-75.2427823716655,
64.1565231694806));
#210062=CARTESIAN_POINT('Ctrl Pts',(-58.0472871244789,-73.7765356555165,
67.7402424800745));
#210063=CARTESIAN_POINT('Ctrl Pts',(-57.9314066489499,-73.8269317955608,
71.6119841758515));
#210064=CARTESIAN_POINT('Ctrl Pts',(-57.8155261734199,-75.3859602001198,
75.1563252942432));
#210065=CARTESIAN_POINT('Ctrl Pts',(-57.6996456978909,-78.2058094306096,
77.8098840079436));
#210066=CARTESIAN_POINT('Ctrl Pts',(-57.5837652223619,-81.8382574454312,
79.1508705661768));
#210067=CARTESIAN_POINT('Ctrl Pts',(-57.4678847468319,-85.7059176071747,
78.9661318235942));
#210068=CARTESIAN_POINT('Ctrl Pts',(-57.3520042713029,-89.1940157232479,
77.2850324623463));
#210069=CARTESIAN_POINT('Ctrl Pts',(-57.2361237957739,-91.7481099313085,
74.3747874028884));
#210070=CARTESIAN_POINT('Ctrl Pts',(-57.1202433202449,-92.9622206108914,
70.6979873284379));
#210071=CARTESIAN_POINT('Ctrl Pts',(-57.0043628447149,-92.6433618528013,
66.8390687464838));
#210072=CARTESIAN_POINT('Ctrl Pts',(-56.8884823691859,-90.8422170489019,
63.4114163537942));
#210073=CARTESIAN_POINT('Ctrl Pts',(-56.7726018936569,-87.8450826410214,
60.9598640147741));
#210074=CARTESIAN_POINT('Ctrl Pts',(-56.6567214181279,-84.1283605902155,
59.8740920651051));
#210075=CARTESIAN_POINT('Ctrl Pts',(-56.5408409425989,-80.2828331013019,
60.3266866536539));
#210076=CARTESIAN_POINT('Ctrl Pts',(-56.4249604670699,-76.9197563235507,
62.2457067472406));
#210077=CARTESIAN_POINT('Ctrl Pts',(-56.3090799915409,-74.5736996668511,
65.326119329296));
#210078=CARTESIAN_POINT('Ctrl Pts',(-56.1931995160109,-73.6175746663254,
69.0782851830545));
#210079=CARTESIAN_POINT('Ctrl Pts',(-56.0773190404819,-74.2033597651636,
72.9057881597825));
#210080=CARTESIAN_POINT('Ctrl Pts',(-55.9614385649529,-76.2379429712918,
76.2002373876932));
#210081=CARTESIAN_POINT('Ctrl Pts',(-55.8455580894239,-79.3979222106296,
78.4379710938565));
#210082=CARTESIAN_POINT('Ctrl Pts',(-55.7296776138959,-83.1810109994356,
79.2632992392267));
#210083=CARTESIAN_POINT('Ctrl Pts',(-55.6137971383669,-86.9858777216637,
78.545021572567));
#210084=CARTESIAN_POINT('Ctrl Pts',(-55.4979166628379,-90.2077303033346,
76.3973559875148));
#210085=CARTESIAN_POINT('Ctrl Pts',(-55.3820361873089,-92.3344437431285,
73.1615080615852));
#210086=CARTESIAN_POINT('Ctrl Pts',(-55.3047825369559,-92.7968044630577,
70.6221445556835));
#210087=CARTESIAN_POINT('Ctrl Pts',(-55.2661557117799,-92.7707412264758,
69.357442022453));
#210088=CARTESIAN_POINT('Ctrl Pts',(-62.4583780353789,-91.8230019028041,
74.5904921130553));
#210089=CARTESIAN_POINT('Ctrl Pts',(-62.4197512102019,-92.4970812476076,
73.4525899438658));
#210090=CARTESIAN_POINT('Ctrl Pts',(-62.3424975598499,-93.3820044778794,
70.903153272674));
#210091=CARTESIAN_POINT('Ctrl Pts',(-62.2266170843209,-93.1099627814073,
66.863814728757));
#210092=CARTESIAN_POINT('Ctrl Pts',(-62.1107366087909,-91.2813956951746,
63.2519304250261));
#210093=CARTESIAN_POINT('Ctrl Pts',(-61.9948561332619,-88.1870497514119,
60.6414643074804));
#210094=CARTESIAN_POINT('Ctrl Pts',(-61.8789756577329,-84.3187544758582,
59.4473977261369));
#210095=CARTESIAN_POINT('Ctrl Pts',(-61.7630951822039,-80.2913915654904,
59.8595194715136));
#210096=CARTESIAN_POINT('Ctrl Pts',(-61.6472147066739,-76.7451186061521,
61.8123247315614));
#210097=CARTESIAN_POINT('Ctrl Pts',(-61.5313342311449,-74.2436249664418,
64.9954094640758));
#210098=CARTESIAN_POINT('Ctrl Pts',(-61.4154537556159,-73.1845291497573,
68.9028146546496));
#210099=CARTESIAN_POINT('Ctrl Pts',(-61.2995732800859,-73.7361771014411,
72.9134484825933));
#210100=CARTESIAN_POINT('Ctrl Pts',(-61.1836928045569,-75.8108829998573,
76.3898107511057));
#210101=CARTESIAN_POINT('Ctrl Pts',(-61.0678123290279,-79.0788671899051,
78.7793250358795));
#210102=CARTESIAN_POINT('Ctrl Pts',(-60.9519318534979,-83.0206754640438,
79.7021721052772));
#210103=CARTESIAN_POINT('Ctrl Pts',(-60.8360513779689,-87.0097476031586,
79.0116631243528));
#210104=CARTESIAN_POINT('Ctrl Pts',(-60.7201709024389,-90.4120106791324,
76.8175562113822));
#210105=CARTESIAN_POINT('Ctrl Pts',(-60.6042904269099,-92.6866665225346,
73.468610111819));
#210106=CARTESIAN_POINT('Ctrl Pts',(-60.4884099513809,-93.4721529352706,
69.4971481292357));
#210107=CARTESIAN_POINT('Ctrl Pts',(-60.3725294758509,-92.6436149003541,
65.5344440135603));
#210108=CARTESIAN_POINT('Ctrl Pts',(-60.2566490003219,-90.332750597095,
62.210379430011));
#210109=CARTESIAN_POINT('Ctrl Pts',(-60.1407685247919,-86.9068776482263,
60.0533227033745));
#210110=CARTESIAN_POINT('Ctrl Pts',(-60.0248880492629,-82.9105470711673,
59.4061433599308));
#210111=CARTESIAN_POINT('Ctrl Pts',(-59.9090075737329,-78.9789855407346,
60.3717121643543));
#210112=CARTESIAN_POINT('Ctrl Pts',(-59.7931270982039,-75.7371245308324,
62.796549556049));
#210113=CARTESIAN_POINT('Ctrl Pts',(-59.6772466226739,-73.7002659039675,
66.2952216066778));
#210114=CARTESIAN_POINT('Ctrl Pts',(-59.5613661471449,-73.192173399811,
70.3116057007245));
#210115=CARTESIAN_POINT('Ctrl Pts',(-59.4454856716149,-74.2936095843438,
74.2072876070263));
#210116=CARTESIAN_POINT('Ctrl Pts',(-59.3296051960859,-76.8294984393236,
77.3630390070701));
#210117=CARTESIAN_POINT('Ctrl Pts',(-59.2137247205559,-80.3967541303873,
79.277245374799));
#210118=CARTESIAN_POINT('Ctrl Pts',(-59.0978442450269,-84.4283525019679,
79.6456388518811));
#210119=CARTESIAN_POINT('Ctrl Pts',(-58.9819637694969,-88.2834609756893,
78.4096623797982));
#210120=CARTESIAN_POINT('Ctrl Pts',(-58.8660832939679,-91.3493004809464,
75.765777489781));
#210121=CARTESIAN_POINT('Ctrl Pts',(-58.7502028184379,-93.13854821078,72.1342362543011));
#210122=CARTESIAN_POINT('Ctrl Pts',(-58.6343223429089,-93.3667987928187,
68.0922811759415));
#210123=CARTESIAN_POINT('Ctrl Pts',(-58.5184418673799,-91.997771229922,
64.282391057355));
#210124=CARTESIAN_POINT('Ctrl Pts',(-58.4025613918499,-89.2490758548062,
61.3101573992296));
#210125=CARTESIAN_POINT('Ctrl Pts',(-58.2866809163209,-85.5576246269588,
59.6480241265653));
#210126=CARTESIAN_POINT('Ctrl Pts',(-58.1708004407909,-81.5101828911056,
59.5601914529124));
#210127=CARTESIAN_POINT('Ctrl Pts',(-58.0549199652619,-77.7501015677444,
61.0606205999848));
#210128=CARTESIAN_POINT('Ctrl Pts',(-57.9390394897319,-74.875054925804,
63.9108146267733));
#210129=CARTESIAN_POINT('Ctrl Pts',(-57.8231590142029,-73.3420387725811,
67.6577281109136));
#210130=CARTESIAN_POINT('Ctrl Pts',(-57.7072785386739,-73.3947298346776,
71.7057798442351));
#210131=CARTESIAN_POINT('Ctrl Pts',(-57.5913980631439,-75.0247527368537,
75.4115219456312));
#210132=CARTESIAN_POINT('Ctrl Pts',(-57.4755175876149,-77.9730112887291,
78.1859175005156));
#210133=CARTESIAN_POINT('Ctrl Pts',(-57.3596371120859,-81.7708724680175,
79.5879694419674));
#210134=CARTESIAN_POINT('Ctrl Pts',(-57.2437566365559,-85.8146568038154,
79.3948181302474));
#210135=CARTESIAN_POINT('Ctrl Pts',(-57.1278761610269,-89.4615947284621,
77.6371654462713));
#210136=CARTESIAN_POINT('Ctrl Pts',(-57.0119956854979,-92.1319963973636,
74.5943946513581));
#210137=CARTESIAN_POINT('Ctrl Pts',(-56.8961152099689,-93.4013948301736,
70.7501617236546));
#210138=CARTESIAN_POINT('Ctrl Pts',(-56.7802347344389,-93.0680159919581,
66.7155170386891));
#210139=CARTESIAN_POINT('Ctrl Pts',(-56.6643542589099,-91.1848512773756,
63.1317773939326));
#210140=CARTESIAN_POINT('Ctrl Pts',(-56.5484737833809,-88.0512343968762,
60.568587110321));
#210141=CARTESIAN_POINT('Ctrl Pts',(-56.4325933078519,-84.1652615396361,
59.4333716522234));
#210142=CARTESIAN_POINT('Ctrl Pts',(-56.3167128323229,-80.1446177466814,
59.9065763370039));
#210143=CARTESIAN_POINT('Ctrl Pts',(-56.2008323567939,-76.6283943389352,
61.9129841055395));
#210144=CARTESIAN_POINT('Ctrl Pts',(-56.0849518812639,-74.1755037636287,
65.1336714529826));
#210145=CARTESIAN_POINT('Ctrl Pts',(-55.9690714057349,-73.1758390727135,
69.0567021408465));
#210146=CARTESIAN_POINT('Ctrl Pts',(-55.8531909302059,-73.7882994512876,
73.0585006275909));
#210147=CARTESIAN_POINT('Ctrl Pts',(-55.7373104546769,-75.9155328055053,
76.5029713478119));
#210148=CARTESIAN_POINT('Ctrl Pts',(-55.6214299791479,-79.2194100892149,
78.8426061994354));
#210149=CARTESIAN_POINT('Ctrl Pts',(-55.5055495036199,-83.1747718700718,
79.705517853136));
#210150=CARTESIAN_POINT('Ctrl Pts',(-55.3896690280909,-87.1529033003677,
78.9545315059016));
#210151=CARTESIAN_POINT('Ctrl Pts',(-55.2737885525619,-90.5214714933247,
76.7090662664086));
#210152=CARTESIAN_POINT('Ctrl Pts',(-55.1579080770329,-92.7450304759939,
73.3258654140387));
#210153=CARTESIAN_POINT('Ctrl Pts',(-55.0806544266799,-93.2284460188592,
70.6708652489211));
#210154=CARTESIAN_POINT('Ctrl Pts',(-55.0420276015039,-93.2011959236129,
69.348571128068));
#210155=CARTESIAN_POINT('Ctrl Pts',(-62.2342499251029,-92.1934303316092,
74.8099293892526));
#210156=CARTESIAN_POINT('Ctrl Pts',(-62.1956230999259,-92.8968687267479,
73.6224666938168));
#210157=CARTESIAN_POINT('Ctrl Pts',(-62.1183694495739,-93.8203341640412,
70.961991106913));
#210158=CARTESIAN_POINT('Ctrl Pts',(-62.0024889740439,-93.5364438833945,
66.7467220222676));
#210159=CARTESIAN_POINT('Ctrl Pts',(-61.8866084985149,-91.6282348476794,
62.977524645695));
#210160=CARTESIAN_POINT('Ctrl Pts',(-61.7707280229859,-88.3991168492557,
60.25336151795));
#210161=CARTESIAN_POINT('Ctrl Pts',(-61.6548475474569,-84.3623407018535,
59.0072882090149));
#210162=CARTESIAN_POINT('Ctrl Pts',(-61.5389670719279,-80.1595688410345,
59.4373596262817));
#210163=CARTESIAN_POINT('Ctrl Pts',(-61.4230865963979,-76.4588404646688,
61.4752179418164));
#210164=CARTESIAN_POINT('Ctrl Pts',(-61.3072061208689,-73.8483960341625,
64.7969396843518));
#210165=CARTESIAN_POINT('Ctrl Pts',(-61.1913256453399,-72.7431720463215,
68.8745291515197));
#210166=CARTESIAN_POINT('Ctrl Pts',(-61.0754451698099,-73.3188466353806,
73.0598433065361));
#210167=CARTESIAN_POINT('Ctrl Pts',(-60.9595646942809,-75.4839148855997,
76.6876160812524));
#210168=CARTESIAN_POINT('Ctrl Pts',(-60.8436842187519,-78.8942338216446,
79.1812039750164));
#210169=CARTESIAN_POINT('Ctrl Pts',(-60.7278037432219,-83.0077247744123,
80.1442449974989));
#210170=CARTESIAN_POINT('Ctrl Pts',(-60.6119232676929,-87.1705381364528,
79.4236613850277));
#210171=CARTESIAN_POINT('Ctrl Pts',(-60.4960427921629,-90.7209843805715,
77.1339916933007));
#210172=CARTESIAN_POINT('Ctrl Pts',(-60.3801623166339,-93.0947112545776,
73.6391846088869));
#210173=CARTESIAN_POINT('Ctrl Pts',(-60.2642818411039,-93.9144089739031,
69.4947484013197));
#210174=CARTESIAN_POINT('Ctrl Pts',(-60.1484013655749,-93.0497845493678,
65.3594515033776));
#210175=CARTESIAN_POINT('Ctrl Pts',(-60.0325208900459,-90.638272181575,
61.8906096318565));
#210176=CARTESIAN_POINT('Ctrl Pts',(-59.9166404145159,-87.0631877532088,
59.6396038211845));
#210177=CARTESIAN_POINT('Ctrl Pts',(-59.8007599389869,-82.8927998170843,
58.9642370379884));
#210178=CARTESIAN_POINT('Ctrl Pts',(-59.6848794634569,-78.790001897706,
59.9718605105236));
#210179=CARTESIAN_POINT('Ctrl Pts',(-59.5689989879279,-75.4069439184913,
62.5023099842152));
#210180=CARTESIAN_POINT('Ctrl Pts',(-59.4531185123979,-73.2813713510347,
66.1533642278691));
#210181=CARTESIAN_POINT('Ctrl Pts',(-59.3372380368689,-72.7511492362934,
70.3446790977719));
#210182=CARTESIAN_POINT('Ctrl Pts',(-59.2213575613389,-73.9005576968343,
74.4100346812925));
#210183=CARTESIAN_POINT('Ctrl Pts',(-59.1054770858099,-76.5468954019475,
77.7032326073398));
#210184=CARTESIAN_POINT('Ctrl Pts',(-58.9895966102799,-80.2695203981129,
79.7008108830386));
#210185=CARTESIAN_POINT('Ctrl Pts',(-58.8737161347509,-84.4767121926759,
80.0852494781352));
#210186=CARTESIAN_POINT('Ctrl Pts',(-58.7578356592209,-88.4997271963806,
78.7954409227263));
#210187=CARTESIAN_POINT('Ctrl Pts',(-58.6419551836919,-91.6990971784923,
76.0364034914596));
#210188=CARTESIAN_POINT('Ctrl Pts',(-58.5260747081619,-93.566274330974,
72.2466930393405));
#210189=CARTESIAN_POINT('Ctrl Pts',(-58.4101942326329,-93.8044662060933,
68.0286934589439));
#210190=CARTESIAN_POINT('Ctrl Pts',(-58.2943137571039,-92.375811613486,
64.0528662639258));
#210191=CARTESIAN_POINT('Ctrl Pts',(-58.1784332815739,-89.5073987503684,
60.9511790655875));
#210192=CARTESIAN_POINT('Ctrl Pts',(-58.0625528060449,-85.6551689684265,
59.2166527507833));
#210193=CARTESIAN_POINT('Ctrl Pts',(-57.9466723305149,-81.4314437630425,
59.1249945869912));
#210194=CARTESIAN_POINT('Ctrl Pts',(-57.8307918549859,-77.5075947501924,
60.6907738670809));
#210195=CARTESIAN_POINT('Ctrl Pts',(-57.7149113794559,-74.5073274799646,
63.6651060840353));
#210196=CARTESIAN_POINT('Ctrl Pts',(-57.5990309039269,-72.9075418896531,
67.575213741715));
#210197=CARTESIAN_POINT('Ctrl Pts',(-57.4831504283979,-72.9625278737866,
71.7995755125808));
#210198=CARTESIAN_POINT('Ctrl Pts',(-57.3672699528679,-74.6635452735643,
75.6667185969865));
#210199=CARTESIAN_POINT('Ctrl Pts',(-57.2513894773389,-77.740213146816,
78.5619509930675));
#210200=CARTESIAN_POINT('Ctrl Pts',(-57.1355090018099,-81.7034874905648,
80.0250683177526));
#210201=CARTESIAN_POINT('Ctrl Pts',(-57.0196285262799,-85.923396000422,
79.8235044369147));
#210202=CARTESIAN_POINT('Ctrl Pts',(-56.9037480507509,-89.7291737336331,
77.9892984302229));
#210203=CARTESIAN_POINT('Ctrl Pts',(-56.7878675752219,-92.5158828633906,
74.8140018998643));
#210204=CARTESIAN_POINT('Ctrl Pts',(-56.6719870996929,-93.8405690494495,
70.8023361189084));
#210205=CARTESIAN_POINT('Ctrl Pts',(-56.5561066241629,-93.4926701311195,
66.5919653309314));
#210206=CARTESIAN_POINT('Ctrl Pts',(-56.4402261486339,-91.5274855058807,
62.8521384340946));
#210207=CARTESIAN_POINT('Ctrl Pts',(-56.3243456731049,-88.2573861527595,
60.1773102058844));
#210208=CARTESIAN_POINT('Ctrl Pts',(-56.2084651975759,-84.2021624890806,
58.992651239347));
#210209=CARTESIAN_POINT('Ctrl Pts',(-56.0925847220469,-80.0064023920941,
59.4864660203554));
#210210=CARTESIAN_POINT('Ctrl Pts',(-55.9767042465179,-76.3370323543386,
61.5802614638165));
#210211=CARTESIAN_POINT('Ctrl Pts',(-55.8608237709879,-73.7773078604179,
64.9412235766449));
#210212=CARTESIAN_POINT('Ctrl Pts',(-55.7449432954589,-72.7341034791027,
69.0351190986164));
#210213=CARTESIAN_POINT('Ctrl Pts',(-55.6290628199299,-73.3732391374036,
73.2112130953808));
#210214=CARTESIAN_POINT('Ctrl Pts',(-55.5131823444009,-75.5931226397066,
76.8057053079184));
#210215=CARTESIAN_POINT('Ctrl Pts',(-55.3973018688719,-79.0408979677858,
79.2472413050084));
#210216=CARTESIAN_POINT('Ctrl Pts',(-55.2814213933429,-83.1685327406974,
80.1477364670454));
#210217=CARTESIAN_POINT('Ctrl Pts',(-55.1655409178149,-87.3199288790655,
79.3640414392398));
#210218=CARTESIAN_POINT('Ctrl Pts',(-55.0496604422859,-90.8352126833059,
77.0207765453072));
#210219=CARTESIAN_POINT('Ctrl Pts',(-54.9337799667569,-93.155617208859,
73.4902227664913));
#210220=CARTESIAN_POINT('Ctrl Pts',(-54.8565263164039,-93.6600875746688,
70.7195859421521));
#210221=CARTESIAN_POINT('Ctrl Pts',(-54.8178994912279,-93.6316506207481,
69.3397002336783));
#210222=CARTESIAN_POINT('',(-62.7285891236391,-92.4023459513537,69.9231276410267));
#210223=CARTESIAN_POINT('Ctrl Pts',(-65.2384132905482,-92.5793602293726,
65.0087087433499));
#210224=CARTESIAN_POINT('Ctrl Pts',(-65.2029278919597,-92.020907624565,
63.8703843309197));
#210225=CARTESIAN_POINT('Ctrl Pts',(-65.1319570947826,-90.4796880229805,
61.8024113142918));
#210226=CARTESIAN_POINT('Ctrl Pts',(-65.0255008990171,-87.2049470387258,
59.7419494328986));
#210227=CARTESIAN_POINT('Ctrl Pts',(-64.9190447032515,-83.4077236954013,
59.0003860876845));
#210228=CARTESIAN_POINT('Ctrl Pts',(-64.8125885074859,-79.5984301452028,
59.6773007910861));
#210229=CARTESIAN_POINT('Ctrl Pts',(-64.7061323117203,-76.2891695109715,
61.6817243939745));
#210230=CARTESIAN_POINT('Ctrl Pts',(-64.5996761159548,-73.9248064731438,
64.7441915297996));
#210231=CARTESIAN_POINT('Ctrl Pts',(-64.4932199201892,-72.8231867097155,
68.4530125546885));
#210232=CARTESIAN_POINT('Ctrl Pts',(-64.3867637244237,-73.1324022343814,
72.3096048992952));
#210233=CARTESIAN_POINT('Ctrl Pts',(-64.2803075286581,-74.8108848414099,
75.7955215493427));
#210234=CARTESIAN_POINT('Ctrl Pts',(-64.1738513328926,-77.632993750829,
78.4421459656915));
#210235=CARTESIAN_POINT('Ctrl Pts',(-64.0673951371271,-81.2193488611975,
79.8936880956339));
#210236=CARTESIAN_POINT('Ctrl Pts',(-63.9609389413616,-85.0878315917651,
79.9550174392733));
#210237=CARTESIAN_POINT('Ctrl Pts',(-63.8544827455961,-88.7183957428313,
78.6178806428873));
#210238=CARTESIAN_POINT('Ctrl Pts',(-63.7480265498306,-91.6229818614739,
76.0620635928089));
#210239=CARTESIAN_POINT('Ctrl Pts',(-63.6415703540651,-93.41111347443,72.6310262841576));
#210240=CARTESIAN_POINT('Ctrl Pts',(-63.5705995568881,-93.6986662915826,
70.0679844126328));
#210241=CARTESIAN_POINT('Ctrl Pts',(-63.5351141582999,-93.6066243106656,
68.8033975024123));
#210242=CARTESIAN_POINT('Ctrl Pts',(-65.0142851802722,-92.1928244408197,
65.1983400256205));
#210243=CARTESIAN_POINT('Ctrl Pts',(-64.9787997816837,-91.6576796881873,
64.1075252799263));
#210244=CARTESIAN_POINT('Ctrl Pts',(-64.9078289845066,-90.1807851848182,
62.1258622007476));
#210245=CARTESIAN_POINT('Ctrl Pts',(-64.801372788741,-87.0427203985795,
60.1513967683751));
#210246=CARTESIAN_POINT('Ctrl Pts',(-64.6949165929754,-83.4039798336089,
59.4407836751363));
#210247=CARTESIAN_POINT('Ctrl Pts',(-64.5884603972099,-79.7536728298564,
60.0894463340284));
#210248=CARTESIAN_POINT('Ctrl Pts',(-64.4820042014443,-76.5825291227051,
62.0102123290093));
#210249=CARTESIAN_POINT('Ctrl Pts',(-64.3755480056787,-74.3168463018152,
64.9448628324088));
#210250=CARTESIAN_POINT('Ctrl Pts',(-64.2690918099132,-73.261204281863,
68.4988906815204));
#210251=CARTESIAN_POINT('Ctrl Pts',(-64.1626356141476,-73.5575142355291,
72.1945223939759));
#210252=CARTESIAN_POINT('Ctrl Pts',(-64.0561794183821,-75.1659428681317,
75.5349491147065));
#210253=CARTESIAN_POINT('Ctrl Pts',(-63.9497232226166,-77.8702668541082,
78.0711127145998));
#210254=CARTESIAN_POINT('Ctrl Pts',(-63.843267026851,-81.306940086253,79.4620725693219));
#210255=CARTESIAN_POINT('Ctrl Pts',(-63.7368108310855,-85.013965921681,
79.5208422413552));
#210256=CARTESIAN_POINT('Ctrl Pts',(-63.63035463532,-88.4930030642919,78.2395128430028));
#210257=CARTESIAN_POINT('Ctrl Pts',(-63.5238984395549,-91.2763619501754,
75.7903666285429));
#210258=CARTESIAN_POINT('Ctrl Pts',(-63.4174422437889,-92.989863223953,
72.5025287780578));
#210259=CARTESIAN_POINT('Ctrl Pts',(-63.3464714466119,-93.265414595499,
70.046459280852));
#210260=CARTESIAN_POINT('Ctrl Pts',(-63.3109860480239,-93.1772141238976,
68.834651790985));
#210261=CARTESIAN_POINT('Ctrl Pts',(-64.7901570699962,-91.8062886522624,
65.3879713079068));
#210262=CARTESIAN_POINT('Ctrl Pts',(-64.7546716714076,-91.2944517518238,
64.3446662289411));
#210263=CARTESIAN_POINT('Ctrl Pts',(-64.6837008742306,-89.8818823466701,
62.4493130872115));
#210264=CARTESIAN_POINT('Ctrl Pts',(-64.577244678465,-86.8804937584546,
60.5608441038513));
#210265=CARTESIAN_POINT('Ctrl Pts',(-64.4707884826994,-83.4002359718365,
59.8811812625842));
#210266=CARTESIAN_POINT('Ctrl Pts',(-64.3643322869338,-79.9089155145195,
60.5015918769625));
#210267=CARTESIAN_POINT('Ctrl Pts',(-64.2578760911682,-76.8758887344474,
62.3387002640362));
#210268=CARTESIAN_POINT('Ctrl Pts',(-64.1514198954027,-74.7088861304908,
65.1455341350097));
#210269=CARTESIAN_POINT('Ctrl Pts',(-64.0449636996371,-73.6992218540112,
68.5447688083423));
#210270=CARTESIAN_POINT('Ctrl Pts',(-63.9385075038716,-73.9826262366747,
72.0794398886478));
#210271=CARTESIAN_POINT('Ctrl Pts',(-63.832051308106,-75.5210008948488,
75.2743766800647));
#210272=CARTESIAN_POINT('Ctrl Pts',(-63.7255951123405,-78.1075399573813,
77.7000794635042));
#210273=CARTESIAN_POINT('Ctrl Pts',(-63.619138916575,-81.3945313113022,
79.0304570430103));
#210274=CARTESIAN_POINT('Ctrl Pts',(-63.5126827208099,-84.9401002515923,
79.086667043439));
#210275=CARTESIAN_POINT('Ctrl Pts',(-63.4062265250439,-88.2676103857406,
77.8611450431156));
#210276=CARTESIAN_POINT('Ctrl Pts',(-63.2997703292789,-90.9297420388772,
75.5186696642778));
#210277=CARTESIAN_POINT('Ctrl Pts',(-63.1933141335129,-92.5686129734675,
72.3740312719635));
#210278=CARTESIAN_POINT('Ctrl Pts',(-63.1223433363359,-92.8321628994063,
70.0249341490751));
#210279=CARTESIAN_POINT('Ctrl Pts',(-63.0868579377479,-92.7478039371384,
68.8659060795531));
#210280=CARTESIAN_POINT('Ctrl Pts',(-64.5660289597201,-91.4197528637094,
65.5776025901771));
#210281=CARTESIAN_POINT('Ctrl Pts',(-64.5305435611316,-90.9312238154461,
64.5818071779478));
#210282=CARTESIAN_POINT('Ctrl Pts',(-64.4595727639545,-89.5829795085174,
62.7727639736644));
#210283=CARTESIAN_POINT('Ctrl Pts',(-64.3531165681889,-86.7182671183082,
60.9702914393278));
#210284=CARTESIAN_POINT('Ctrl Pts',(-64.2466603724233,-83.3964921100534,
60.3215788500321));
#210285=CARTESIAN_POINT('Ctrl Pts',(-64.1402041766578,-80.0641581991723,
60.9137374199029));
#210286=CARTESIAN_POINT('Ctrl Pts',(-64.0337479808922,-77.1692483461807,
62.6671881990701));
#210287=CARTESIAN_POINT('Ctrl Pts',(-63.9272917851266,-75.1009259591622,
65.3462054376189));
#210288=CARTESIAN_POINT('Ctrl Pts',(-63.8208355893611,-74.1372394261586,
68.5906469351742));
#210289=CARTESIAN_POINT('Ctrl Pts',(-63.7143793935955,-74.4077382378226,
71.9643573833285));
#210290=CARTESIAN_POINT('Ctrl Pts',(-63.60792319783,-75.8760589215704,75.0138042454286));
#210291=CARTESIAN_POINT('Ctrl Pts',(-63.5014670020649,-78.3448130606606,
77.3290462124125));
#210292=CARTESIAN_POINT('Ctrl Pts',(-63.3950108062989,-81.4821225363578,
78.5988415166983));
#210293=CARTESIAN_POINT('Ctrl Pts',(-63.2885546105339,-84.8662345815091,
78.6524918455205));
#210294=CARTESIAN_POINT('Ctrl Pts',(-63.1820984147679,-88.0422177072,77.4827772432284));
#210295=CARTESIAN_POINT('Ctrl Pts',(-63.0756422190029,-90.5831221275879,
75.2469727000079));
#210296=CARTESIAN_POINT('Ctrl Pts',(-62.9691860232369,-92.1473627229813,
72.2455337658675));
#210297=CARTESIAN_POINT('Ctrl Pts',(-62.8982152260599,-92.3989112033227,
70.0034090172943));
#210298=CARTESIAN_POINT('Ctrl Pts',(-62.8627298274719,-92.3183937503701,
68.8971603681249));
#210299=CARTESIAN_POINT('Ctrl Pts',(-64.5675364832709,-89.3666802039723,
62.5540045030464));
#210300=CARTESIAN_POINT('Ctrl Pts',(-64.5675364832709,-89.6837232097609,
62.8628731621223));
#210301=CARTESIAN_POINT('Ctrl Pts',(-64.5675364832687,-89.9771780606084,
63.1936835736481));
#210302=CARTESIAN_POINT('Ctrl Pts',(-64.5675364832687,-90.5061924891354,
63.8842115791694));
#210303=CARTESIAN_POINT('Ctrl Pts',(-64.5675364832709,-90.7431890489746,
64.2429885299648));
#210304=CARTESIAN_POINT('Ctrl Pts',(-64.5675364832709,-90.9537820568252,
64.6166308207592));
#210305=CARTESIAN_POINT('Ctrl Pts',(-63.5337949169409,-93.5594912036319,
69.9703303450313));
#210306=CARTESIAN_POINT('Ctrl Pts',(-63.5394868426676,-93.551300696559,
70.1709662592206));
#210307=CARTESIAN_POINT('Ctrl Pts',(-63.5451666556007,-93.5372160945861,
70.3713185694425));
#210308=CARTESIAN_POINT('Ctrl Pts',(-63.5564167240733,-93.4975597846317,
70.7682868434331));
#210309=CARTESIAN_POINT('Ctrl Pts',(-63.561985078531,-93.4721513323048,
70.9648330212324));
#210310=CARTESIAN_POINT('Ctrl Pts',(-63.5675399484426,-93.4410622313485,
71.1605188170969));
#210311=CARTESIAN_POINT('Origin',(-49.5265537491909,-84.0265789317952,61.9560808081071));
#210312=CARTESIAN_POINT('',(-47.1840596451126,-83.4464714330094,62.1957559421789));
#210313=CARTESIAN_POINT('',(-39.7523422906826,-81.6060420553333,62.9561411445197));
#210314=CARTESIAN_POINT('',(-47.1840596451109,-83.4464714330093,62.1957559421787));
#210315=CARTESIAN_POINT('',(-47.119731784661,-80.7405384334922,63.3137295174306));
#210316=CARTESIAN_POINT('Origin',(-113.778845940191,-80.7405384334922,63.3137295174306));
#210317=CARTESIAN_POINT('Origin',(-113.778845940191,-80.7405384334922,63.3137295174306));
#210318=CARTESIAN_POINT('Origin',(27.1782499005891,-72.4225170988655,66.75037338561));
#210319=CARTESIAN_POINT('Origin',(27.1782499005891,-75.,72.98888938658));
#210320=CARTESIAN_POINT('Origin',(27.1782499005891,-75.,72.98888938658));
#210321=CARTESIAN_POINT('',(-39.7523422906826,-86.7610078576023,75.4331731464598));
#210322=CARTESIAN_POINT('Origin',(27.1782499005891,-77.5774829011345,79.2274053875501));
#210323=CARTESIAN_POINT('Ctrl Pts',(-39.7523422906848,-81.6060420553332,
62.9561411445199));
#210324=CARTESIAN_POINT('Ctrl Pts',(-39.7281387736131,-82.5738094980375,
63.4318987914185));
#210325=CARTESIAN_POINT('Ctrl Pts',(-39.7067753132048,-83.5053294334335,
64.0835294670284));
#210326=CARTESIAN_POINT('Ctrl Pts',(-39.6724659131911,-85.2832094673282,
65.8377960430231));
#210327=CARTESIAN_POINT('Ctrl Pts',(-39.6628533608352,-86.0573358731186,
67.0147663024293));
#210328=CARTESIAN_POINT('Ctrl Pts',(-39.6628533608352,-87.0495295570505,
69.4162628052949));
#210329=CARTESIAN_POINT('Ctrl Pts',(-39.6724659131911,-87.3318920083316,
70.7964084967982));
#210330=CARTESIAN_POINT('Ctrl Pts',(-39.7067753132048,-87.3106857783487,
73.2939791024836));
#210331=CARTESIAN_POINT('Ctrl Pts',(-39.7281387736131,-87.1107535098341,
74.4130765135442));
#210332=CARTESIAN_POINT('Ctrl Pts',(-39.7523422906848,-86.7610078576022,
75.4331731464597));
#210333=CARTESIAN_POINT('Origin',(-23.4378585958609,-75.,72.98888938658));
#210334=CARTESIAN_POINT('Ctrl Pts',(-23.3090332587941,-63.2240228732978,
77.8543002128611));
#210335=CARTESIAN_POINT('Ctrl Pts',(-23.3534781005806,-62.83121418956,77.0199591890652));
#210336=CARTESIAN_POINT('Ctrl Pts',(-23.3969857639789,-62.5315314215813,
76.148166123812));
#210337=CARTESIAN_POINT('Ctrl Pts',(-23.4821035727885,-62.1231202708912,
74.3427299956358));
#210338=CARTESIAN_POINT('Ctrl Pts',(-23.5241358609361,-62.0176287394905,
73.4125249276314));
#210339=CARTESIAN_POINT('Ctrl Pts',(-23.5675316904176,-62.0095472178182,
72.4907563613072));
#210340=CARTESIAN_POINT('Ctrl Pts',(-38.3758095864366,-79.7336577641993,
83.8196273194874));
#210341=CARTESIAN_POINT('Ctrl Pts',(-38.4258466097666,-77.8912456464383,
84.7194504420196));
#210342=CARTESIAN_POINT('Ctrl Pts',(-38.525920656419,-73.6862797614722,
85.5568522331397));
#210343=CARTESIAN_POINT('Ctrl Pts',(-38.6760317264166,-67.4554874534197,
83.4636401838067));
#210344=CARTESIAN_POINT('Ctrl Pts',(-38.826142796409,-63.0004712968532,
78.4421077647582));
#210345=CARTESIAN_POINT('Ctrl Pts',(-38.9262168430666,-62.0709193802797,
73.9710084799022));
#210346=CARTESIAN_POINT('Ctrl Pts',(-38.9762538663893,-62.2003708352002,
71.7442636422223));
#210347=CARTESIAN_POINT('Ctrl Pts',(-38.4975359461084,-79.7336577641993,
83.8196273194874));
#210348=CARTESIAN_POINT('Ctrl Pts',(-38.5475729694384,-77.8912456464383,
84.7194504420196));
#210349=CARTESIAN_POINT('Ctrl Pts',(-38.647647016096,-73.6862797614722,
85.5568522331397));
#210350=CARTESIAN_POINT('Ctrl Pts',(-38.7977580860884,-67.4554874534197,
83.4636401838067));
#210351=CARTESIAN_POINT('Ctrl Pts',(-38.947869156086,-63.0004712968532,
78.4421077647582));
#210352=CARTESIAN_POINT('Ctrl Pts',(-39.0479432027384,-62.0709193802797,
73.9710084799022));
#210353=CARTESIAN_POINT('Ctrl Pts',(-39.0979802260676,-62.2003708352002,
71.7442636422223));
#210354=CARTESIAN_POINT('Ctrl Pts',(-38.6192623057863,-79.7336577641993,
83.8196273194874));
#210355=CARTESIAN_POINT('Ctrl Pts',(-38.6692993291154,-77.8912456464383,
84.7194504420196));
#210356=CARTESIAN_POINT('Ctrl Pts',(-38.7693733757677,-73.6862797614722,
85.5568522331397));
#210357=CARTESIAN_POINT('Ctrl Pts',(-38.9194844457654,-67.4554874534197,
83.4636401838067));
#210358=CARTESIAN_POINT('Ctrl Pts',(-39.0695955157577,-63.0004712968532,
78.4421077647582));
#210359=CARTESIAN_POINT('Ctrl Pts',(-39.1696695624154,-62.0709193802797,
73.9710084799022));
#210360=CARTESIAN_POINT('Ctrl Pts',(-39.2197065857454,-62.2003708352002,
71.7442636422223));
#210361=CARTESIAN_POINT('Ctrl Pts',(-38.7409886654647,-79.7336577641993,
83.8196273194874));
#210362=CARTESIAN_POINT('Ctrl Pts',(-38.7910256887871,-77.8912456464383,
84.7194504420196));
#210363=CARTESIAN_POINT('Ctrl Pts',(-38.8910997354449,-73.6862797614722,
85.5568522331397));
#210364=CARTESIAN_POINT('Ctrl Pts',(-39.0412108054371,-67.4554874534197,
83.4636401838067));
#210365=CARTESIAN_POINT('Ctrl Pts',(-39.1913218754349,-63.0004712968532,
78.4421077647582));
#210366=CARTESIAN_POINT('Ctrl Pts',(-39.2913959220871,-62.0709193802797,
73.9710084799022));
#210367=CARTESIAN_POINT('Ctrl Pts',(-39.341432945417,-62.2003708352002,
71.7442636422223));
#210368=CARTESIAN_POINT('',(-38.9948861699879,-62.1810067989059,72.2582005417311));
#210369=CARTESIAN_POINT('Ctrl Pts',(-38.4175364832709,-79.3040007179705,
84.018699824741));
#210370=CARTESIAN_POINT('Ctrl Pts',(-38.4515840088404,-78.0242319180911,
84.580297006929));
#210371=CARTESIAN_POINT('Ctrl Pts',(-38.4856315344087,-76.6337365057753,
84.9164019235577));
#210372=CARTESIAN_POINT('Ctrl Pts',(-38.5196790599775,-75.2185063065921,
85.0027014193313));
#210373=CARTESIAN_POINT('Ctrl Pts',(-38.5318196218509,-74.7138678780693,
85.0334738279151));
#210374=CARTESIAN_POINT('Ctrl Pts',(-38.5439601837242,-74.2060847177368,
85.0324846379198));
#210375=CARTESIAN_POINT('Ctrl Pts',(-38.5561007455978,-73.6990558480383,
84.9986331104708));
#210376=CARTESIAN_POINT('Ctrl Pts',(-38.6061377689272,-71.6093489921214,
84.859114883362));
#210377=CARTESIAN_POINT('Ctrl Pts',(-38.6561747922594,-69.5324182227705,
84.1613775335844));
#210378=CARTESIAN_POINT('Ctrl Pts',(-38.7062118155911,-67.7514501453341,
82.9755867888541));
#210379=CARTESIAN_POINT('Ctrl Pts',(-38.7562488389227,-65.9704820678976,
81.7897960441239));
#210380=CARTESIAN_POINT('Ctrl Pts',(-38.8062858622539,-64.4854766823754,
80.115951904441));
#210381=CARTESIAN_POINT('Ctrl Pts',(-38.8563228855836,-63.5105860104709,
78.1612550133856));
#210382=CARTESIAN_POINT('Ctrl Pts',(-38.8900113257437,-62.8542211054953,
76.8452157116171));
#210383=CARTESIAN_POINT('Ctrl Pts',(-38.9236997659031,-62.4290840399959,
75.4018511432914));
#210384=CARTESIAN_POINT('Ctrl Pts',(-38.9573884811954,-62.2608540356083,
73.919597891675));
#210385=CARTESIAN_POINT('Ctrl Pts',(-38.9698878032445,-62.1984366657286,
73.3696463547994));
#210386=CARTESIAN_POINT('Ctrl Pts',(-38.9823871631681,-62.1713843280277,
72.8143415959309));
#210387=CARTESIAN_POINT('Ctrl Pts',(-38.9948865750186,-62.1810067178394,
72.2582005494316));
#210388=CARTESIAN_POINT('',(-39.2948856689521,-62.1810067177622,72.2582005309434));
#210389=CARTESIAN_POINT('',(-38.9948867524609,-62.1810067181578,72.2582005310305));
#210390=CARTESIAN_POINT('Ctrl Pts',(-38.7175257490599,-79.3043967631952,
84.0185260206292));
#210391=CARTESIAN_POINT('Ctrl Pts',(-38.7475365958835,-78.1763594241,84.5135891741795));
#210392=CARTESIAN_POINT('Ctrl Pts',(-38.7773577336901,-76.9698200260516,
84.8302771319025));
#210393=CARTESIAN_POINT('Ctrl Pts',(-38.8371612694423,-74.4971301206813,
85.0901078006421));
#210394=CARTESIAN_POINT('Ctrl Pts',(-38.8666805284219,-73.2491623894031,
85.0253215589554));
#210395=CARTESIAN_POINT('Ctrl Pts',(-38.9333423802022,-70.5016684508897,
84.4457335806271));
#210396=CARTESIAN_POINT('Ctrl Pts',(-38.9699089016275,-69.0435745979185,
83.8358955289173));
#210397=CARTESIAN_POINT('Ctrl Pts',(-39.0430464798089,-66.4403850004115,
82.1026671558932));
#210398=CARTESIAN_POINT('Ctrl Pts',(-39.0796009224146,-65.3002030898782,
80.9726262266062));
#210399=CARTESIAN_POINT('Ctrl Pts',(-39.1461000544407,-63.6601136043194,
78.5958132558447));
#210400=CARTESIAN_POINT('Ctrl Pts',(-39.1756663161435,-63.0966943303126,
77.4163792493374));
#210401=CARTESIAN_POINT('Ctrl Pts',(-39.2353970967561,-62.3417992295227,
74.9007486757214));
#210402=CARTESIAN_POINT('Ctrl Pts',(-39.2652280895187,-62.1581747903836,
73.5778073419933));
#210403=CARTESIAN_POINT('Ctrl Pts',(-39.2948856682995,-62.1810067181595,
72.2582005309356));
#210404=CARTESIAN_POINT('Ctrl Pts',(-22.1107451997509,-75.5739040289331,
84.8149721769878));
#210405=CARTESIAN_POINT('Ctrl Pts',(-22.1554803513709,-73.7414528439281,
84.9038985896114));
#210406=CARTESIAN_POINT('Ctrl Pts',(-22.2449506545909,-70.0361529743874,
84.2144079552725));
#210407=CARTESIAN_POINT('Ctrl Pts',(-22.3791561094309,-65.5303320257027,
80.7979303917428));
#210408=CARTESIAN_POINT('Ctrl Pts',(-22.5133615642709,-63.034536682417,
75.7241832750653));
#210409=CARTESIAN_POINT('Ctrl Pts',(-22.6475670191109,-63.0779852322991,
70.0699504067063));
#210410=CARTESIAN_POINT('Ctrl Pts',(-22.7817724739509,-65.6515761891153,
65.0351802123127));
#210411=CARTESIAN_POINT('Ctrl Pts',(-22.9159779287909,-70.2091042452636,
61.6883646725776));
#210412=CARTESIAN_POINT('Ctrl Pts',(-23.0501833836309,-75.7833689502356,
60.7397722098011));
#210413=CARTESIAN_POINT('Ctrl Pts',(-23.1843888384709,-81.1913848225435,
62.3907153943343));
#210414=CARTESIAN_POINT('Ctrl Pts',(-23.3185942933109,-85.2854509968364,
66.2908272630258));
#210415=CARTESIAN_POINT('Ctrl Pts',(-23.4527997481509,-87.1967152341949,
71.6124171753859));
#210416=CARTESIAN_POINT('Ctrl Pts',(-23.5870052029909,-86.5195647170419,
77.2261251637649));
#210417=CARTESIAN_POINT('Ctrl Pts',(-23.7212106578309,-83.3977058628873,
81.9405972979454));
#210418=CARTESIAN_POINT('Ctrl Pts',(-23.8554161126709,-78.4936666911383,
84.7553175337842));
#210419=CARTESIAN_POINT('Ctrl Pts',(-23.9896215675109,-72.8481935946092,
85.0729395141451));
#210420=CARTESIAN_POINT('Ctrl Pts',(-24.1238270223509,-67.6593817681323,
82.8260567769256));
#210421=CARTESIAN_POINT('Ctrl Pts',(-24.2580324771909,-64.0284127084992,
78.4915079084072));
#210422=CARTESIAN_POINT('Ctrl Pts',(-24.3922379320309,-62.7258589625622,
72.9891807694126));
#210423=CARTESIAN_POINT('Ctrl Pts',(-24.5264433868709,-64.0281514612617,
67.4867917924942));
#210424=CARTESIAN_POINT('Ctrl Pts',(-24.6606488417109,-67.6589147161704,
63.1520705335424));
#210425=CARTESIAN_POINT('Ctrl Pts',(-24.7948542965509,-72.8476198566583,
60.9049414386412));
#210426=CARTESIAN_POINT('Ctrl Pts',(-24.9290597513909,-78.4931080275489,
61.2222953760157));
#210427=CARTESIAN_POINT('Ctrl Pts',(-25.0632652062309,-83.3972808331134,
64.0367827707003));
#210428=CARTESIAN_POINT('Ctrl Pts',(-25.1974706610709,-86.5193635271416,
68.7511066704761));
#210429=CARTESIAN_POINT('Ctrl Pts',(-25.3316761159109,-87.1967805614843,
74.3647825240851));
#210430=CARTESIAN_POINT('Ctrl Pts',(-25.4658815707509,-85.2857690508221,
79.6864630932148));
#210431=CARTESIAN_POINT('Ctrl Pts',(-25.6000870255909,-81.1918878310654,
83.586769647843));
#210432=CARTESIAN_POINT('Ctrl Pts',(-25.7342924804309,-75.7839511863107,
85.2379684505081));
#210433=CARTESIAN_POINT('Ctrl Pts',(-25.8684979352709,-70.2096383289215,
84.2896449343191));
#210434=CARTESIAN_POINT('Ctrl Pts',(-26.0027033901109,-65.6519630192656,
80.9430297969228));
#210435=CARTESIAN_POINT('Ctrl Pts',(-26.1369088449509,-63.0780895580271,
75.9084414716367));
#210436=CARTESIAN_POINT('Ctrl Pts',(-26.2711142997909,-63.0345347478559,
70.2539879752973));
#210437=CARTESIAN_POINT('Ctrl Pts',(-26.3605846030209,-64.6978341565217,
66.8719649808208));
#210438=CARTESIAN_POINT('Ctrl Pts',(-26.4053197546309,-65.8649786513045,
65.456493688071));
#210439=CARTESIAN_POINT('Ctrl Pts',(-22.2602140739609,-75.5739040289331,
84.8149721769878));
#210440=CARTESIAN_POINT('Ctrl Pts',(-22.3049492255709,-73.7414528439281,
84.9038985896114));
#210441=CARTESIAN_POINT('Ctrl Pts',(-22.3944195288009,-70.0361529743874,
84.2144079552725));
#210442=CARTESIAN_POINT('Ctrl Pts',(-22.5286249836409,-65.5303320257027,
80.7979303917428));
#210443=CARTESIAN_POINT('Ctrl Pts',(-22.6628304384809,-63.034536682417,
75.7241832750653));
#210444=CARTESIAN_POINT('Ctrl Pts',(-22.7970358933209,-63.0779852322991,
70.0699504067063));
#210445=CARTESIAN_POINT('Ctrl Pts',(-22.9312413481609,-65.6515761891153,
65.0351802123127));
#210446=CARTESIAN_POINT('Ctrl Pts',(-23.0654468030009,-70.2091042452636,
61.6883646725776));
#210447=CARTESIAN_POINT('Ctrl Pts',(-23.1996522578409,-75.7833689502356,
60.7397722098011));
#210448=CARTESIAN_POINT('Ctrl Pts',(-23.3338577126809,-81.1913848225435,
62.3907153943343));
#210449=CARTESIAN_POINT('Ctrl Pts',(-23.4680631675209,-85.2854509968364,
66.2908272630258));
#210450=CARTESIAN_POINT('Ctrl Pts',(-23.6022686223609,-87.1967152341949,
71.6124171753859));
#210451=CARTESIAN_POINT('Ctrl Pts',(-23.7364740772009,-86.5195647170419,
77.2261251637649));
#210452=CARTESIAN_POINT('Ctrl Pts',(-23.8706795320409,-83.3977058628873,
81.9405972979454));
#210453=CARTESIAN_POINT('Ctrl Pts',(-24.0048849868809,-78.4936666911383,
84.7553175337842));
#210454=CARTESIAN_POINT('Ctrl Pts',(-24.1390904417209,-72.8481935946092,
85.0729395141451));
#210455=CARTESIAN_POINT('Ctrl Pts',(-24.2732958965609,-67.6593817681323,
82.8260567769256));
#210456=CARTESIAN_POINT('Ctrl Pts',(-24.4075013514009,-64.0284127084992,
78.4915079084072));
#210457=CARTESIAN_POINT('Ctrl Pts',(-24.5417068062409,-62.7258589625622,
72.9891807694126));
#210458=CARTESIAN_POINT('Ctrl Pts',(-24.6759122610809,-64.0281514612617,
67.4867917924942));
#210459=CARTESIAN_POINT('Ctrl Pts',(-24.8101177159209,-67.6589147161704,
63.1520705335424));
#210460=CARTESIAN_POINT('Ctrl Pts',(-24.9443231707609,-72.8476198566583,
60.9049414386412));
#210461=CARTESIAN_POINT('Ctrl Pts',(-25.0785286256009,-78.4931080275489,
61.2222953760157));
#210462=CARTESIAN_POINT('Ctrl Pts',(-25.2127340804409,-83.3972808331134,
64.0367827707003));
#210463=CARTESIAN_POINT('Ctrl Pts',(-25.3469395352809,-86.5193635271416,
68.7511066704761));
#210464=CARTESIAN_POINT('Ctrl Pts',(-25.4811449901209,-87.1967805614843,
74.3647825240851));
#210465=CARTESIAN_POINT('Ctrl Pts',(-25.6153504449609,-85.2857690508221,
79.6864630932148));
#210466=CARTESIAN_POINT('Ctrl Pts',(-25.7495558998009,-81.1918878310654,
83.586769647843));
#210467=CARTESIAN_POINT('Ctrl Pts',(-25.8837613546409,-75.7839511863107,
85.2379684505081));
#210468=CARTESIAN_POINT('Ctrl Pts',(-26.0179668094809,-70.2096383289215,
84.2896449343191));
#210469=CARTESIAN_POINT('Ctrl Pts',(-26.1521722643209,-65.6519630192656,
80.9430297969228));
#210470=CARTESIAN_POINT('Ctrl Pts',(-26.2863777191609,-63.0780895580271,
75.9084414716367));
#210471=CARTESIAN_POINT('Ctrl Pts',(-26.4205831740009,-63.0345347478559,
70.2539879752973));
#210472=CARTESIAN_POINT('Ctrl Pts',(-26.5100534772209,-64.6978341565217,
66.8719649808208));
#210473=CARTESIAN_POINT('Ctrl Pts',(-26.5547886288309,-65.8649786513045,
65.456493688071));
#210474=CARTESIAN_POINT('Ctrl Pts',(-22.4096829481609,-75.5739040289331,
84.8149721769878));
#210475=CARTESIAN_POINT('Ctrl Pts',(-22.4544180997809,-73.7414528439281,
84.9038985896114));
#210476=CARTESIAN_POINT('Ctrl Pts',(-22.5438884030009,-70.0361529743874,
84.2144079552725));
#210477=CARTESIAN_POINT('Ctrl Pts',(-22.6780938578409,-65.5303320257027,
80.7979303917428));
#210478=CARTESIAN_POINT('Ctrl Pts',(-22.8122993126809,-63.034536682417,
75.7241832750653));
#210479=CARTESIAN_POINT('Ctrl Pts',(-22.9465047675209,-63.0779852322991,
70.0699504067063));
#210480=CARTESIAN_POINT('Ctrl Pts',(-23.0807102223609,-65.6515761891153,
65.0351802123127));
#210481=CARTESIAN_POINT('Ctrl Pts',(-23.2149156772009,-70.2091042452636,
61.6883646725776));
#210482=CARTESIAN_POINT('Ctrl Pts',(-23.3491211320409,-75.7833689502356,
60.7397722098011));
#210483=CARTESIAN_POINT('Ctrl Pts',(-23.4833265868809,-81.1913848225435,
62.3907153943343));
#210484=CARTESIAN_POINT('Ctrl Pts',(-23.6175320417209,-85.2854509968364,
66.2908272630258));
#210485=CARTESIAN_POINT('Ctrl Pts',(-23.7517374965609,-87.1967152341949,
71.6124171753859));
#210486=CARTESIAN_POINT('Ctrl Pts',(-23.8859429514009,-86.5195647170419,
77.2261251637649));
#210487=CARTESIAN_POINT('Ctrl Pts',(-24.0201484062409,-83.3977058628873,
81.9405972979454));
#210488=CARTESIAN_POINT('Ctrl Pts',(-24.1543538610809,-78.4936666911383,
84.7553175337842));
#210489=CARTESIAN_POINT('Ctrl Pts',(-24.2885593159209,-72.8481935946092,
85.0729395141451));
#210490=CARTESIAN_POINT('Ctrl Pts',(-24.4227647707609,-67.6593817681323,
82.8260567769256));
#210491=CARTESIAN_POINT('Ctrl Pts',(-24.5569702256009,-64.0284127084992,
78.4915079084072));
#210492=CARTESIAN_POINT('Ctrl Pts',(-24.6911756804409,-62.7258589625622,
72.9891807694126));
#210493=CARTESIAN_POINT('Ctrl Pts',(-24.8253811352809,-64.0281514612617,
67.4867917924942));
#210494=CARTESIAN_POINT('Ctrl Pts',(-24.9595865901209,-67.6589147161704,
63.1520705335424));
#210495=CARTESIAN_POINT('Ctrl Pts',(-25.0937920449609,-72.8476198566583,
60.9049414386412));
#210496=CARTESIAN_POINT('Ctrl Pts',(-25.2279974998009,-78.4931080275489,
61.2222953760157));
#210497=CARTESIAN_POINT('Ctrl Pts',(-25.3622029546409,-83.3972808331134,
64.0367827707003));
#210498=CARTESIAN_POINT('Ctrl Pts',(-25.4964084094809,-86.5193635271416,
68.7511066704761));
#210499=CARTESIAN_POINT('Ctrl Pts',(-25.6306138643209,-87.1967805614843,
74.3647825240851));
#210500=CARTESIAN_POINT('Ctrl Pts',(-25.7648193191609,-85.2857690508221,
79.6864630932148));
#210501=CARTESIAN_POINT('Ctrl Pts',(-25.8990247740009,-81.1918878310654,
83.586769647843));
#210502=CARTESIAN_POINT('Ctrl Pts',(-26.0332302288409,-75.7839511863107,
85.2379684505081));
#210503=CARTESIAN_POINT('Ctrl Pts',(-26.1674356836809,-70.2096383289215,
84.2896449343191));
#210504=CARTESIAN_POINT('Ctrl Pts',(-26.3016411385209,-65.6519630192656,
80.9430297969228));
#210505=CARTESIAN_POINT('Ctrl Pts',(-26.4358465933609,-63.0780895580271,
75.9084414716367));
#210506=CARTESIAN_POINT('Ctrl Pts',(-26.5700520482009,-63.0345347478559,
70.2539879752973));
#210507=CARTESIAN_POINT('Ctrl Pts',(-26.6595223514309,-64.6978341565217,
66.8719649808208));
#210508=CARTESIAN_POINT('Ctrl Pts',(-26.7042575030409,-65.8649786513045,
65.456493688071));
#210509=CARTESIAN_POINT('Ctrl Pts',(-22.5591518223709,-75.5739040289331,
84.8149721769878));
#210510=CARTESIAN_POINT('Ctrl Pts',(-22.6038869739809,-73.7414528439281,
84.9038985896114));
#210511=CARTESIAN_POINT('Ctrl Pts',(-22.6933572772109,-70.0361529743874,
84.2144079552725));
#210512=CARTESIAN_POINT('Ctrl Pts',(-22.8275627320509,-65.5303320257027,
80.7979303917428));
#210513=CARTESIAN_POINT('Ctrl Pts',(-22.9617681868909,-63.034536682417,
75.7241832750653));
#210514=CARTESIAN_POINT('Ctrl Pts',(-23.0959736417309,-63.0779852322991,
70.0699504067063));
#210515=CARTESIAN_POINT('Ctrl Pts',(-23.2301790965709,-65.6515761891153,
65.0351802123127));
#210516=CARTESIAN_POINT('Ctrl Pts',(-23.3643845514109,-70.2091042452636,
61.6883646725776));
#210517=CARTESIAN_POINT('Ctrl Pts',(-23.4985900062509,-75.7833689502356,
60.7397722098011));
#210518=CARTESIAN_POINT('Ctrl Pts',(-23.6327954610909,-81.1913848225435,
62.3907153943343));
#210519=CARTESIAN_POINT('Ctrl Pts',(-23.7670009159309,-85.2854509968364,
66.2908272630258));
#210520=CARTESIAN_POINT('Ctrl Pts',(-23.9012063707709,-87.1967152341949,
71.6124171753859));
#210521=CARTESIAN_POINT('Ctrl Pts',(-24.0354118256109,-86.5195647170419,
77.2261251637649));
#210522=CARTESIAN_POINT('Ctrl Pts',(-24.1696172804509,-83.3977058628873,
81.9405972979454));
#210523=CARTESIAN_POINT('Ctrl Pts',(-24.3038227352909,-78.4936666911383,
84.7553175337842));
#210524=CARTESIAN_POINT('Ctrl Pts',(-24.4380281901309,-72.8481935946092,
85.0729395141451));
#210525=CARTESIAN_POINT('Ctrl Pts',(-24.5722336449709,-67.6593817681323,
82.8260567769256));
#210526=CARTESIAN_POINT('Ctrl Pts',(-24.7064390998109,-64.0284127084992,
78.4915079084072));
#210527=CARTESIAN_POINT('Ctrl Pts',(-24.8406445546509,-62.7258589625622,
72.9891807694126));
#210528=CARTESIAN_POINT('Ctrl Pts',(-24.9748500094909,-64.0281514612617,
67.4867917924942));
#210529=CARTESIAN_POINT('Ctrl Pts',(-25.1090554643309,-67.6589147161704,
63.1520705335424));
#210530=CARTESIAN_POINT('Ctrl Pts',(-25.2432609191709,-72.8476198566583,
60.9049414386412));
#210531=CARTESIAN_POINT('Ctrl Pts',(-25.3774663740109,-78.4931080275489,
61.2222953760157));
#210532=CARTESIAN_POINT('Ctrl Pts',(-25.5116718288509,-83.3972808331134,
64.0367827707003));
#210533=CARTESIAN_POINT('Ctrl Pts',(-25.6458772836909,-86.5193635271416,
68.7511066704761));
#210534=CARTESIAN_POINT('Ctrl Pts',(-25.7800827385309,-87.1967805614843,
74.3647825240851));
#210535=CARTESIAN_POINT('Ctrl Pts',(-25.9142881933709,-85.2857690508221,
79.6864630932148));
#210536=CARTESIAN_POINT('Ctrl Pts',(-26.0484936482109,-81.1918878310654,
83.586769647843));
#210537=CARTESIAN_POINT('Ctrl Pts',(-26.1826991030509,-75.7839511863107,
85.2379684505081));
#210538=CARTESIAN_POINT('Ctrl Pts',(-26.3169045578909,-70.2096383289215,
84.2896449343191));
#210539=CARTESIAN_POINT('Ctrl Pts',(-26.4511100127309,-65.6519630192656,
80.9430297969228));
#210540=CARTESIAN_POINT('Ctrl Pts',(-26.5853154675709,-63.0780895580271,
75.9084414716367));
#210541=CARTESIAN_POINT('Ctrl Pts',(-26.7195209224109,-63.0345347478559,
70.2539879752973));
#210542=CARTESIAN_POINT('Ctrl Pts',(-26.8089912256309,-64.6978341565217,
66.8719649808208));
#210543=CARTESIAN_POINT('Ctrl Pts',(-26.8537263772509,-65.8649786513045,
65.456493688071));
#210544=CARTESIAN_POINT('',(-22.5675364832709,-72.2044512501012,84.4927878836045));
#210545=CARTESIAN_POINT('Ctrl Pts',(-22.5675364832709,-72.2044512501012,
84.4927878836045));
#210546=CARTESIAN_POINT('Ctrl Pts',(-22.5702005749792,-72.101381045307,
84.467793838185));
#210547=CARTESIAN_POINT('Ctrl Pts',(-22.5728694662329,-71.9986439061689,
84.4414253512639));
#210548=CARTESIAN_POINT('Ctrl Pts',(-22.5892107893379,-71.3720639244154,
84.2716538950522));
#210549=CARTESIAN_POINT('Ctrl Pts',(-22.6029000964172,-70.857571028858,
84.0937531121258));
#210550=CARTESIAN_POINT('Ctrl Pts',(-22.6289955618953,-69.8696262372289,
83.6729279463958));
#210551=CARTESIAN_POINT('Ctrl Pts',(-22.6413046609066,-69.3967095048034,
83.4319232204433));
#210552=CARTESIAN_POINT('Ctrl Pts',(-22.6599801160594,-68.7147555205797,
83.0250434553367));
#210553=CARTESIAN_POINT('Ctrl Pts',(-22.6662554004773,-68.4915974755653,
82.8815572226386));
#210554=CARTESIAN_POINT('Ctrl Pts',(-22.6893343517786,-67.7056195601597,
82.3383815790085));
#210555=CARTESIAN_POINT('Ctrl Pts',(-22.7069178421115,-67.1716946281647,
81.8966499936456));
#210556=CARTESIAN_POINT('Ctrl Pts',(-22.7321799276305,-66.4561223902797,
81.191081357374));
#210557=CARTESIAN_POINT('Ctrl Pts',(-22.7400417610185,-66.2408487732195,
80.9612051372088));
#210558=CARTESIAN_POINT('Ctrl Pts',(-22.7616713767574,-65.6637270733977,
80.2927579163368));
#210559=CARTESIAN_POINT('Ctrl Pts',(-22.7748837672742,-65.3251316974417,
79.8367065697317));
#210560=CARTESIAN_POINT('Ctrl Pts',(-22.7947609375481,-64.8709906011954,
79.1240614124061));
#210561=CARTESIAN_POINT('Ctrl Pts',(-22.801362841351,-64.7292600705043,
78.8833334005035));
#210562=CARTESIAN_POINT('Ctrl Pts',(-22.8237826878125,-64.2863646376341,
78.066924839321));
#210563=CARTESIAN_POINT('Ctrl Pts',(-22.8402920915749,-64.0231454411833,
77.4705540397267));
#210564=CARTESIAN_POINT('Ctrl Pts',(-22.8648029152467,-63.7043957916297,
76.5509224533803));
#210565=CARTESIAN_POINT('Ctrl Pts',(-22.8729157189747,-63.6109150950584,
76.2407322943046));
#210566=CARTESIAN_POINT('Ctrl Pts',(-22.8959687353885,-63.3777242540699,
75.3320075975269));
#210567=CARTESIAN_POINT('Ctrl Pts',(-22.9102264149049,-63.272832382873,
74.7270547946618));
#210568=CARTESIAN_POINT('Ctrl Pts',(-22.9311662489802,-63.1886126135983,
73.8409316995098));
#210569=CARTESIAN_POINT('Ctrl Pts',(-22.9377614229422,-63.172002102898,
73.5625527585218));
#210570=CARTESIAN_POINT('Ctrl Pts',(-22.9606740564853,-63.1486501868713,
72.6142548128651));
#210571=CARTESIAN_POINT('Ctrl Pts',(-22.9777573547508,-63.1884849523521,
71.9430921224707));
#210572=CARTESIAN_POINT('Ctrl Pts',(-23.0022394040367,-63.3280072789211,
70.9807639026107));
#210573=CARTESIAN_POINT('Ctrl Pts',(-23.009809992206,-63.3828970341615,
70.6830316322857));
#210574=CARTESIAN_POINT('Ctrl Pts',(-23.0313765416433,-63.575741394923,
69.8254004003008));
#210575=CARTESIAN_POINT('Ctrl Pts',(-23.0447944938312,-63.7437455267563,
69.2740313357485));
#210576=CARTESIAN_POINT('Ctrl Pts',(-23.0652537324288,-64.0568737760211,
68.461953897769));
#210577=CARTESIAN_POINT('Ctrl Pts',(-23.072249157524,-64.1737923279692,
68.1895288572785));
#210578=CARTESIAN_POINT('Ctrl Pts',(-23.0965474361077,-64.6054951171437,
67.2786381453301));
#210579=CARTESIAN_POINT('Ctrl Pts',(-23.1147579084745,-64.967843830616,
66.6626023540414));
#210580=CARTESIAN_POINT('Ctrl Pts',(-23.1397715132475,-65.5471606574156,
65.8542689053473));
#210581=CARTESIAN_POINT('Ctrl Pts',(-23.1468311929961,-65.7201277877051,
65.6303568070702));
#210582=CARTESIAN_POINT('Ctrl Pts',(-23.1676747514321,-66.2648908086861,
64.9758232123873));
#210583=CARTESIAN_POINT('Ctrl Pts',(-23.180917910398,-66.6602300549298,
64.5661869645247));
#210584=CARTESIAN_POINT('Ctrl Pts',(-23.2013065948263,-67.3052464719053,
63.98684644309));
#210585=CARTESIAN_POINT('Ctrl Pts',(-23.2083909984657,-67.5358879433693,
63.7949330533718));
#210586=CARTESIAN_POINT('Ctrl Pts',(-23.2324629811764,-68.3265224511962,
63.1858849928527));
#210587=CARTESIAN_POINT('Ctrl Pts',(-23.2503290955488,-68.9170420587356,
62.8082314172963));
#210588=CARTESIAN_POINT('Ctrl Pts',(-23.2748842311724,-69.7822021340986,
62.3572729968318));
#210589=CARTESIAN_POINT('Ctrl Pts',(-23.2818169730817,-70.0327823351848,
62.2376943943266));
#210590=CARTESIAN_POINT('Ctrl Pts',(-23.3035186130697,-70.8455154209485,
61.8849216123275));
#210591=CARTESIAN_POINT('Ctrl Pts',(-23.3176588018285,-71.4219044077756,
61.6868980638871));
#210592=CARTESIAN_POINT('Ctrl Pts',(-23.3388664824507,-72.2933800065435,
61.4600378227875));
#210593=CARTESIAN_POINT('Ctrl Pts',(-23.3458199835052,-72.5801380471361,
61.3966045554723));
#210594=CARTESIAN_POINT('Ctrl Pts',(-23.3682626536341,-73.4930114596429,
61.2296514049232));
#210595=CARTESIAN_POINT('Ctrl Pts',(-23.3844526926435,-74.1263361552216,
61.1651917382816));
#210596=CARTESIAN_POINT('Ctrl Pts',(-23.407684371625,-75.0471740386811,
61.1458073048583));
#210597=CARTESIAN_POINT('Ctrl Pts',(-23.4148695247781,-75.3338716005414,
61.1502002309391));
#210598=CARTESIAN_POINT('Ctrl Pts',(-23.437206134341,-76.2411868293319,
61.1975982391152));
#210599=CARTESIAN_POINT('Ctrl Pts',(-23.4516854993175,-76.8584841699238,
61.2799207344907));
#210600=CARTESIAN_POINT('Ctrl Pts',(-23.4735337262852,-77.7658938973876,
61.4737526344256));
#210601=CARTESIAN_POINT('Ctrl Pts',(-23.4808192690104,-78.0644314250129,
61.5497313157693));
#210602=CARTESIAN_POINT('Ctrl Pts',(-23.5040385331769,-78.985976686343,
61.8225462972605));
#210603=CARTESIAN_POINT('Ctrl Pts',(-23.5207281916305,-79.5972182308479,
62.0593503041271));
#210604=CARTESIAN_POINT('Ctrl Pts',(-23.5441129061001,-80.4314026015402,
62.4648501692533));
#210605=CARTESIAN_POINT('Ctrl Pts',(-23.5509830628018,-80.673910896464,
62.5933714538943));
#210606=CARTESIAN_POINT('Ctrl Pts',(-23.5725188546082,-81.4338200893154,
63.0311669320082));
#210607=CARTESIAN_POINT('Ctrl Pts',(-23.5865887278414,-81.9320304656956,
63.3723514817783));
#210608=CARTESIAN_POINT('Ctrl Pts',(-23.6083405871127,-82.6525232096769,
63.9503037294639));
#210609=CARTESIAN_POINT('Ctrl Pts',(-23.6159578353334,-82.895558722176,
64.1620087200743));
#210610=CARTESIAN_POINT('Ctrl Pts',(-23.6398805770154,-83.6157764881116,
64.8424376056804));
#210611=CARTESIAN_POINT('Ctrl Pts',(-23.6569839558427,-84.0633982830332,
65.3425405823492));
#210612=CARTESIAN_POINT('Ctrl Pts',(-23.6804648193501,-84.6237728802768,
66.0871527080787));
#210613=CARTESIAN_POINT('Ctrl Pts',(-23.6870485851375,-84.7749847799005,
66.3027475337673));
#210614=CARTESIAN_POINT('Ctrl Pts',(-23.7082031998033,-85.2460366915907,
67.025357154534));
#210615=CARTESIAN_POINT('Ctrl Pts',(-23.7222219941297,-85.5344434917129,
67.5526944759278));
#210616=CARTESIAN_POINT('Ctrl Pts',(-23.7441210530633,-85.917699285489,
68.3991972044296));
#210617=CARTESIAN_POINT('Ctrl Pts',(-23.7519297485863,-86.041288304194,
68.7054045196352));
#210618=CARTESIAN_POINT('Ctrl Pts',(-23.7755298190367,-86.3691023964499,
69.6255567349058));
#210619=CARTESIAN_POINT('Ctrl Pts',(-23.7920487902638,-86.536744826011,
70.2525895074464));
#210620=CARTESIAN_POINT('Ctrl Pts',(-23.8151391213079,-86.6998527884554,
71.1537311340575));
#210621=CARTESIAN_POINT('Ctrl Pts',(-23.8218753913192,-86.7387036230601,
71.420093236262));
#210622=CARTESIAN_POINT('Ctrl Pts',(-23.8433555858714,-86.8349025507093,
72.2904016804811));
#210623=CARTESIAN_POINT('Ctrl Pts',(-23.8575579717939,-86.8543681848811,
72.8983416348768));
#210624=CARTESIAN_POINT('Ctrl Pts',(-23.8798554463617,-86.8126009199117,
73.8427727913579));
#210625=CARTESIAN_POINT('Ctrl Pts',(-23.8878816096207,-86.7831869848533,
74.1806799322738));
#210626=CARTESIAN_POINT('Ctrl Pts',(-23.9110847210234,-86.6594162642764,
75.1323771410212));
#210627=CARTESIAN_POINT('Ctrl Pts',(-23.9269053581022,-86.5313769103644,
75.7418298181749));
#210628=CARTESIAN_POINT('Ctrl Pts',(-23.9495459158712,-86.2782593381081,
76.6026846921188));
#210629=CARTESIAN_POINT('Ctrl Pts',(-23.9564812052765,-86.1908829611717,
76.8653374683523));
#210630=CARTESIAN_POINT('Ctrl Pts',(-23.978357349735,-85.87951350085,77.7003660271306));
#210631=CARTESIAN_POINT('Ctrl Pts',(-23.9927641337887,-85.6192994879538,
78.2589304827335));
#210632=CARTESIAN_POINT('Ctrl Pts',(-24.0155119050259,-85.1462650587442,
79.0984245577459));
#210633=CARTESIAN_POINT('Ctrl Pts',(-24.0237891876252,-84.9614493005972,
79.395151667052));
#210634=CARTESIAN_POINT('Ctrl Pts',(-24.0466112890863,-84.4281573134537,
80.1732424407857));
#210635=CARTESIAN_POINT('Ctrl Pts',(-24.0617134596371,-84.0557500977274,
80.6382476573784));
#210636=CARTESIAN_POINT('Ctrl Pts',(-24.0839137958733,-83.455843100956,
81.2812040167729));
#210637=CARTESIAN_POINT('Ctrl Pts',(-24.0910796733786,-83.2534875950334,
81.482882460786));
#210638=CARTESIAN_POINT('Ctrl Pts',(-24.114057595194,-82.5668987389516,
82.1183964911421));
#210639=CARTESIAN_POINT('Ctrl Pts',(-24.1292856506188,-82.0531629663279,
82.5197843027206));
#210640=CARTESIAN_POINT('Ctrl Pts',(-24.1528881185347,-81.2191982476438,
83.0682211280836));
#210641=CARTESIAN_POINT('Ctrl Pts',(-24.1611669801199,-80.9197306683576,
83.2468935918955));
#210642=CARTESIAN_POINT('Ctrl Pts',(-24.1827559596316,-80.1362205425358,
83.6690821495163));
#210643=CARTESIAN_POINT('Ctrl Pts',(-24.1964874148007,-79.6419118838925,
83.8935996769975));
#210644=CARTESIAN_POINT('Ctrl Pts',(-24.2174768257468,-78.8635400001464,
84.1843685432751));
#210645=CARTESIAN_POINT('Ctrl Pts',(-24.2247571552006,-78.5886510660862,
84.2756825250963));
#210646=CARTESIAN_POINT('Ctrl Pts',(-24.2483756982726,-77.6675515482579,
84.5438270605521));
#210647=CARTESIAN_POINT('Ctrl Pts',(-24.2640946299932,-77.0085486087368,
84.6754742522788));
#210648=CARTESIAN_POINT('Ctrl Pts',(-24.2884926428815,-75.9843843113636,
84.7918940227002));
#210649=CARTESIAN_POINT('Ctrl Pts',(-24.2970807599795,-75.6237028793401,
84.8163932788448));
#210650=CARTESIAN_POINT('Ctrl Pts',(-24.3182126869125,-74.753379085836,
84.8359863747897));
#210651=CARTESIAN_POINT('Ctrl Pts',(-24.331086847875,-74.2433492494284,
84.8148743652152));
#210652=CARTESIAN_POINT('Ctrl Pts',(-24.3515180034849,-73.4391621471866,
84.7292196212527));
#210653=CARTESIAN_POINT('Ctrl Pts',(-24.3590613604395,-73.1425132511634,
84.6861535064079));
#210654=CARTESIAN_POINT('Ctrl Pts',(-24.3815384824964,-72.2455386694007,
84.5202236828175));
#210655=CARTESIAN_POINT('Ctrl Pts',(-24.3960069964874,-71.6522821119051,
84.3613414335283));
#210656=CARTESIAN_POINT('Ctrl Pts',(-24.420087747924,-70.6927799935796,
84.0234693101138));
#210657=CARTESIAN_POINT('Ctrl Pts',(-24.4296875364308,-70.3176894943474,
83.8695157327615));
#210658=CARTESIAN_POINT('Ctrl Pts',(-24.4517726454239,-69.492170899461,
83.4806056486045));
#210659=CARTESIAN_POINT('Ctrl Pts',(-24.4645281627022,-69.0467282022266,
83.2349870119561));
#210660=CARTESIAN_POINT('Ctrl Pts',(-24.4851445577002,-68.3588257034976,
82.7956074273213));
#210661=CARTESIAN_POINT('Ctrl Pts',(-24.4929344656444,-68.1050651461329,
82.6191436156437));
#210662=CARTESIAN_POINT('Ctrl Pts',(-24.5153697889196,-67.3800154221781,
82.0707183485821));
#210663=CARTESIAN_POINT('Ctrl Pts',(-24.5295968633418,-66.9295782058471,
81.6718532422255));
#210664=CARTESIAN_POINT('Ctrl Pts',(-24.5540914658925,-66.2096628206234,
80.9304241509229));
#210665=CARTESIAN_POINT('Ctrl Pts',(-24.564365750269,-65.9246307267622,
80.6029215596546));
#210666=CARTESIAN_POINT('Ctrl Pts',(-24.5860905187512,-65.3728346095594,
79.894567924767));
#210667=CARTESIAN_POINT('Ctrl Pts',(-24.5976840511342,-65.1087963504241,
79.511541722129));
#210668=CARTESIAN_POINT('Ctrl Pts',(-24.6172620568231,-64.7068591408205,
78.8479458411513));
#210669=CARTESIAN_POINT('Ctrl Pts',(-24.6251367322929,-64.5560611690603,
78.5751882904969));
#210670=CARTESIAN_POINT('Ctrl Pts',(-24.6472317420048,-64.1564776850288,
77.778450069505));
#210671=CARTESIAN_POINT('Ctrl Pts',(-24.6610648696814,-63.9353368803934,
77.240709445703));
#210672=CARTESIAN_POINT('Ctrl Pts',(-24.6908945637497,-63.5435177201768,
76.0472767679771));
#210673=CARTESIAN_POINT('Ctrl Pts',(-24.7068825789407,-63.3872882704072,
75.3867366115899));
#210674=CARTESIAN_POINT('Ctrl Pts',(-24.7317749488675,-63.2391139871652,
74.3879117013547));
#210675=CARTESIAN_POINT('Ctrl Pts',(-24.7401923448886,-63.204033550018,
74.0559075222267));
#210676=CARTESIAN_POINT('Ctrl Pts',(-24.7610996526955,-63.1520046518361,
73.2283760432204));
#210677=CARTESIAN_POINT('Ctrl Pts',(-24.7733789330876,-63.1523239657399,
72.7345232328324));
#210678=CARTESIAN_POINT('Ctrl Pts',(-24.7975533204228,-63.2163039535267,
71.7369892425429));
#210679=CARTESIAN_POINT('Ctrl Pts',(-24.8094922231537,-63.2808630596704,
71.2360827207114));
#210680=CARTESIAN_POINT('Ctrl Pts',(-24.8351973708289,-63.4864194352961,
70.1752564221956));
#210681=CARTESIAN_POINT('Ctrl Pts',(-24.8489873208506,-63.6371013798287,
69.6171097101316));
#210682=CARTESIAN_POINT('Ctrl Pts',(-24.871569359364,-63.9377876836337,
68.7570415397288));
#210683=CARTESIAN_POINT('Ctrl Pts',(-24.8800360304053,-64.0615447344729,
68.4458729535586));
#210684=CARTESIAN_POINT('Ctrl Pts',(-24.9001649362169,-64.3887688614134,
67.7156793928846));
#210685=CARTESIAN_POINT('Ctrl Pts',(-24.9116058676399,-64.6036307349302,
67.304238822933));
#210686=CARTESIAN_POINT('Ctrl Pts',(-24.936773504184,-65.1398482256562,
66.4104777396577));
#210687=CARTESIAN_POINT('Ctrl Pts',(-24.9504401609289,-65.4735636386861,
65.9367826121286));
#210688=CARTESIAN_POINT('Ctrl Pts',(-24.9762719223671,-66.1587653668953,
65.099986780096));
#210689=CARTESIAN_POINT('Ctrl Pts',(-24.9884096401357,-66.5025277537145,
64.7304245665408));
#210690=CARTESIAN_POINT('Ctrl Pts',(-25.0096077839027,-67.1226339839138,
64.143431275759));
#210691=CARTESIAN_POINT('Ctrl Pts',(-25.0184772157891,-67.3876176298573,
63.9139452540245));
#210692=CARTESIAN_POINT('Ctrl Pts',(-25.0395422051437,-68.0467493322417,
63.3929967902548));
#210693=CARTESIAN_POINT('Ctrl Pts',(-25.051481480533,-68.4488671084499,
63.1146464292296));
#210694=CARTESIAN_POINT('Ctrl Pts',(-25.0840133009887,-69.605829643291,
62.4152363687055));
#210695=CARTESIAN_POINT('Ctrl Pts',(-25.104319479274,-70.3943111889634,
62.0491341885859));
#210696=CARTESIAN_POINT('Ctrl Pts',(-25.1367303308552,-71.6511389741192,
61.623800462803));
#210697=CARTESIAN_POINT('Ctrl Pts',(-25.1483805833471,-72.0982070991733,
61.5009928872146));
#210698=CARTESIAN_POINT('Ctrl Pts',(-25.1736387791001,-73.0833297619818,
61.2922240109905));
#210699=CARTESIAN_POINT('Ctrl Pts',(-25.18690328478,-73.6212370846174,61.2172565919412));
#210700=CARTESIAN_POINT('Ctrl Pts',(-25.2253780352521,-75.2159620477906,
61.1054031807067));
#210701=CARTESIAN_POINT('Ctrl Pts',(-25.2502026720849,-76.280546882193,
61.1724865348266));
#210702=CARTESIAN_POINT('Ctrl Pts',(-25.2868501328567,-77.724738435485,
61.4594462472879));
#210703=CARTESIAN_POINT('Ctrl Pts',(-25.2973866547898,-78.1284078048523,
61.5619808193849));
#210704=CARTESIAN_POINT('Ctrl Pts',(-25.3189006619814,-78.9588852174617,
61.8212918368161));
#210705=CARTESIAN_POINT('Ctrl Pts',(-25.3298740811697,-79.3836100045202,
61.9815962718169));
#210706=CARTESIAN_POINT('Ctrl Pts',(-25.3676607858402,-80.8209660344883,
62.620119032157));
#210707=CARTESIAN_POINT('Ctrl Pts',(-25.3942496696967,-81.7803037275957,
63.2194097958438));
#210708=CARTESIAN_POINT('Ctrl Pts',(-25.4315170012924,-82.9187865576204,
64.1789466500218));
#210709=CARTESIAN_POINT('Ctrl Pts',(-25.4407247650091,-83.1891272839219,
64.4295735366799));
#210710=CARTESIAN_POINT('Ctrl Pts',(-25.4634471275391,-83.8379068478192,
65.091061289566));
#210711=CARTESIAN_POINT('Ctrl Pts',(-25.4768210572136,-84.1994663576492,
65.5163497127943));
#210712=CARTESIAN_POINT('Ctrl Pts',(-25.5082872674835,-84.9777305813297,
66.5732280735895));
#210713=CARTESIAN_POINT('Ctrl Pts',(-25.5263741675259,-85.3681341316777,
67.2244202926804));
#210714=CARTESIAN_POINT('Ctrl Pts',(-25.5565118018322,-85.892517668506,
68.3253303899162));
#210715=CARTESIAN_POINT('Ctrl Pts',(-25.5682319358942,-86.0673700339834,
68.7558528469077));
#210716=CARTESIAN_POINT('Ctrl Pts',(-25.5936707871693,-86.3976332999429,
69.7340864108877));
#210717=CARTESIAN_POINT('Ctrl Pts',(-25.6073488507091,-86.5398957155988,
70.284393827016));
#210718=CARTESIAN_POINT('Ctrl Pts',(-25.6390902685798,-86.7786955465479,
71.5834051319908));
#210719=CARTESIAN_POINT('Ctrl Pts',(-25.6571261045347,-86.8447346260927,
72.3378995205217));
#210720=CARTESIAN_POINT('Ctrl Pts',(-25.6886429549223,-86.8346771541917,
73.6213929423741));
#210721=CARTESIAN_POINT('Ctrl Pts',(-25.7020061921809,-86.795000649475,
74.1509454828671));
#210722=CARTESIAN_POINT('Ctrl Pts',(-25.7309197773289,-86.6269076368682,
75.3136246984158));
#210723=CARTESIAN_POINT('Ctrl Pts',(-25.7464095591912,-86.4825368138157,
75.9421181765224));
#210724=CARTESIAN_POINT('Ctrl Pts',(-25.7802443466448,-86.058468686505,
77.2828736886994));
#210725=CARTESIAN_POINT('Ctrl Pts',(-25.7985939560829,-85.758370917871,
77.9889025693498));
#210726=CARTESIAN_POINT('Ctrl Pts',(-25.831032553874,-85.1291604331345,
79.1443949968908));
#210727=CARTESIAN_POINT('Ctrl Pts',(-25.844811107583,-84.8322918439808,
79.6085218961476));
#210728=CARTESIAN_POINT('Ctrl Pts',(-25.8792602330504,-83.990955503201,
80.7386112650431));
#210729=CARTESIAN_POINT('Ctrl Pts',(-25.8997594340109,-83.4048901794276,
81.3694771722443));
#210730=CARTESIAN_POINT('Ctrl Pts',(-25.9579490738006,-81.5877385699402,
82.9475470254536));
#210731=CARTESIAN_POINT('Ctrl Pts',(-25.9960369474434,-80.2388638266101,
83.7179044612192));
#210732=CARTESIAN_POINT('Ctrl Pts',(-26.0520110212422,-78.0417648515169,
84.4556003538643));
#210733=CARTESIAN_POINT('Ctrl Pts',(-26.0705765621172,-77.288612729029,
84.6300887618639));
#210734=CARTESIAN_POINT('Ctrl Pts',(-26.1000724134121,-76.0986710445967,
84.7856474129164));
#210735=CARTESIAN_POINT('Ctrl Pts',(-26.1107596449467,-75.6697395694068,
84.8178911491601));
#210736=CARTESIAN_POINT('Ctrl Pts',(-26.1480724884064,-74.1490259463417,
84.8475873904511));
#210737=CARTESIAN_POINT('Ctrl Pts',(-26.1742484856788,-73.0566099990662,
84.7171041053917));
#210738=CARTESIAN_POINT('Ctrl Pts',(-26.2193931213824,-71.2585880803683,
84.2478848991978));
#210739=CARTESIAN_POINT('Ctrl Pts',(-26.2384151825556,-70.5337737099665,
83.981778363005));
#210740=CARTESIAN_POINT('Ctrl Pts',(-26.2957251622276,-68.4292285265332,
82.9604600860379));
#210741=CARTESIAN_POINT('Ctrl Pts',(-26.3332502293259,-67.1567131535949,
81.9948919179989));
#210742=CARTESIAN_POINT('Ctrl Pts',(-26.3809156049555,-65.8740149622752,
80.5415543079316));
#210743=CARTESIAN_POINT('Ctrl Pts',(-26.3900399203341,-65.641478463133,
80.2509925078922));
#210744=CARTESIAN_POINT('Ctrl Pts',(-26.4361742047054,-64.5325293841572,
78.7228356001248));
#210745=CARTESIAN_POINT('Ctrl Pts',(-26.4727735230356,-63.8780065946758,
77.3230290806258));
#210746=CARTESIAN_POINT('Ctrl Pts',(-26.5412761300322,-63.2022949315233,
74.611776993663));
#210747=CARTESIAN_POINT('Ctrl Pts',(-26.5723193488738,-63.0981845490051,
73.3221947465108));
#210748=CARTESIAN_POINT('Ctrl Pts',(-26.6346898575196,-63.2994981574995,
70.7677501968342));
#210749=CARTESIAN_POINT('Ctrl Pts',(-26.6657005351421,-63.6077274104244,
69.5203338851136));
#210750=CARTESIAN_POINT('Ctrl Pts',(-26.6970005540986,-64.1119403475322,
68.3407908335599));
#210751=CARTESIAN_POINT('',(-22.5673849603904,-63.669040753613,76.420933693241));
#210752=CARTESIAN_POINT('Ctrl Pts',(-22.5675364832709,-63.6687702444235,
76.4210531081683));
#210753=CARTESIAN_POINT('Ctrl Pts',(-22.5675364832709,-63.7258038321112,
76.6088225515179));
#210754=CARTESIAN_POINT('Ctrl Pts',(-22.5675364832709,-63.7873203078865,
76.7945020356765));
#210755=CARTESIAN_POINT('Ctrl Pts',(-22.5675364832709,-63.8532188980627,
76.9781622505545));
#210756=CARTESIAN_POINT('Ctrl Pts',(-22.5675364832709,-63.9184088764334,
77.1598475552547));
#210757=CARTESIAN_POINT('Ctrl Pts',(-22.5675364832709,-63.9878875599488,
77.33955714555));
#210758=CARTESIAN_POINT('Ctrl Pts',(-22.5675364832709,-64.0616097872864,
77.5173473119477));
#210759=CARTESIAN_POINT('Ctrl Pts',(-22.5675364832709,-64.1355001969537,
77.6955430705995));
#210760=CARTESIAN_POINT('Ctrl Pts',(-22.5675364832709,-64.2136537188044,
77.8718110268248));
#210761=CARTESIAN_POINT('Ctrl Pts',(-22.5675364832709,-64.2960741558206,
78.0461899469697));
#210762=CARTESIAN_POINT('Ctrl Pts',(-22.5675364832709,-64.378330446047,
78.2202215777655));
#210763=CARTESIAN_POINT('Ctrl Pts',(-22.5675364832709,-64.4648368683367,
78.3923720715572));
#210764=CARTESIAN_POINT('Ctrl Pts',(-22.5675364832709,-64.5556433242083,
78.5626563900689));
#210765=CARTESIAN_POINT('Ctrl Pts',(-22.5675364832709,-64.6480925106386,
78.7360212302351));
#210766=CARTESIAN_POINT('Ctrl Pts',(-22.5675364832709,-64.7449987516446,
78.9074522896587));
#210767=CARTESIAN_POINT('Ctrl Pts',(-22.5675364832709,-64.8464610303325,
79.0769339040445));
#210768=CARTESIAN_POINT('Ctrl Pts',(-22.5675364832709,-64.8669864107892,
79.1112193021322));
#210769=CARTESIAN_POINT('Ctrl Pts',(-22.5675364832709,-64.8876983884462,
79.145424805595));
#210770=CARTESIAN_POINT('Ctrl Pts',(-22.5675364832709,-64.9085980057327,
79.1795501013398));
#210771=CARTESIAN_POINT('Ctrl Pts',(-22.5675364832709,-64.9174000338929,
79.1939222216519));
#210772=CARTESIAN_POINT('Ctrl Pts',(-22.5675364832709,-64.9262364572077,
79.2082819116383));
#210773=CARTESIAN_POINT('Ctrl Pts',(-22.5675364832709,-64.9351037869345,
79.222623373272));
#210774=CARTESIAN_POINT('Ctrl Pts',(-22.5675364832709,-65.0375475668251,
79.3883095024868));
#210775=CARTESIAN_POINT('Ctrl Pts',(-22.5675364832709,-65.1436663874556,
79.5508453779689));
#210776=CARTESIAN_POINT('Ctrl Pts',(-22.5675364832709,-65.2534263053612,
79.7102890247438));
#210777=CARTESIAN_POINT('Ctrl Pts',(-22.5675364832709,-65.3633010588936,
79.8698994884356));
#210778=CARTESIAN_POINT('Ctrl Pts',(-22.5675364832709,-65.4768247520306,
80.0264116215346));
#210779=CARTESIAN_POINT('Ctrl Pts',(-22.5675364832709,-65.5940096958059,
80.1798598398312));
#210780=CARTESIAN_POINT('Ctrl Pts',(-22.5675364832709,-65.6823624769175,
80.2955536858692));
#210781=CARTESIAN_POINT('Ctrl Pts',(-22.5675364832709,-65.7727974833994,
80.4095053827246));
#210782=CARTESIAN_POINT('Ctrl Pts',(-22.5675364832709,-65.8653362932692,
80.5217187995515));
#210783=CARTESIAN_POINT('Ctrl Pts',(-22.5675364832709,-65.987966895796,
80.6704218025018));
#210784=CARTESIAN_POINT('Ctrl Pts',(-22.5675364832709,-66.1142907375747,
80.8160736236853));
#210785=CARTESIAN_POINT('Ctrl Pts',(-22.5675364832709,-66.2443103813311,
80.9587217971806));
#210786=CARTESIAN_POINT('Ctrl Pts',(-22.5675364832709,-66.3745137755541,
81.1015715684322));
#210787=CARTESIAN_POINT('Ctrl Pts',(-22.5675364832709,-66.5084237436001,
81.2414094814956));
#210788=CARTESIAN_POINT('Ctrl Pts',(-22.5675364832709,-66.6460788550177,
81.3782455406439));
#210789=CARTESIAN_POINT('Ctrl Pts',(-22.5675364832709,-66.7103748553523,
81.4421589777416));
#210790=CARTESIAN_POINT('Ctrl Pts',(-22.5675364832709,-66.7754883930306,
81.5054169558065));
#210791=CARTESIAN_POINT('Ctrl Pts',(-22.5675364832709,-66.8414257863485,
81.5680174031831));
#210792=CARTESIAN_POINT('Ctrl Pts',(-22.5675364832709,-66.8594783064253,
81.5851563250637));
#210793=CARTESIAN_POINT('Ctrl Pts',(-22.5675364832709,-66.8775970561921,
81.6022500915462));
#210794=CARTESIAN_POINT('Ctrl Pts',(-22.5675364832709,-66.8957572266453,
81.619275372102));
#210795=CARTESIAN_POINT('Ctrl Pts',(-22.5675364832709,-67.0349336946461,
81.7497542363061));
#210796=CARTESIAN_POINT('Ctrl Pts',(-22.5675364832709,-67.1767618191788,
81.8764274620977));
#210797=CARTESIAN_POINT('Ctrl Pts',(-22.5675364832709,-67.3212106845732,
81.9993967091251));
#210798=CARTESIAN_POINT('Ctrl Pts',(-22.5675364832709,-67.4664417640186,
82.1230318545839));
#210799=CARTESIAN_POINT('Ctrl Pts',(-22.5675364832709,-67.6143223758131,
82.2429230597769));
#210800=CARTESIAN_POINT('Ctrl Pts',(-22.5675364832709,-67.7648596939825,
82.3591374576176));
#210801=CARTESIAN_POINT('Ctrl Pts',(-22.5675364832709,-67.9155872738129,
82.4754987369403));
#210802=CARTESIAN_POINT('Ctrl Pts',(-22.5675364832709,-68.0689786215426,
82.5881741648509));
#210803=CARTESIAN_POINT('Ctrl Pts',(-22.5675364832709,-68.2250744281003,
82.6971910903905));
#210804=CARTESIAN_POINT('Ctrl Pts',(-22.5675364832709,-68.3803784145739,
82.8056550107402));
#210805=CARTESIAN_POINT('Ctrl Pts',(-22.5675364832709,-68.538359844291,
82.9104976776817));
#210806=CARTESIAN_POINT('Ctrl Pts',(-22.5675364832709,-68.6990866879562,
83.0117028805195));
#210807=CARTESIAN_POINT('Ctrl Pts',(-22.5675364832709,-68.819631820705,
83.0876067826479));
#210808=CARTESIAN_POINT('Ctrl Pts',(-22.5675364832709,-68.9417218476887,
83.1614637579624));
#210809=CARTESIAN_POINT('Ctrl Pts',(-22.5675364832709,-69.0653940624834,
83.2332496878576));
#210810=CARTESIAN_POINT('Ctrl Pts',(-22.5675364832709,-69.119053375501,
83.2643964065358));
#210811=CARTESIAN_POINT('Ctrl Pts',(-22.5675364832709,-69.1730106287839,
83.2951530451425));
#210812=CARTESIAN_POINT('Ctrl Pts',(-22.5675364832709,-69.2272692395212,
83.3255167097264));
#210813=CARTESIAN_POINT('Ctrl Pts',(-22.5675364832709,-69.2590702189398,
83.3433128578286));
#210814=CARTESIAN_POINT('Ctrl Pts',(-22.5675364832709,-69.2909747226799,
83.3609740033855));
#210815=CARTESIAN_POINT('Ctrl Pts',(-22.5675364832709,-69.3229834710798,
83.3784994710574));
#210816=CARTESIAN_POINT('Ctrl Pts',(-22.5675364832709,-69.3427780357163,
83.389337414431));
#210817=CARTESIAN_POINT('Ctrl Pts',(-22.5675364832709,-69.362616341774,
83.4001255274541));
#210818=CARTESIAN_POINT('Ctrl Pts',(-22.5675364832709,-69.3824732041753,
83.4108500423031));
#210819=CARTESIAN_POINT('Ctrl Pts',(-22.5675364832709,-69.5606622039941,
83.5070883369465));
#210820=CARTESIAN_POINT('Ctrl Pts',(-22.5675364832709,-69.7407061600605,
83.5984099230677));
#210821=CARTESIAN_POINT('Ctrl Pts',(-22.5675364832709,-69.9225805595835,
83.684846614458));
#210822=CARTESIAN_POINT('Ctrl Pts',(-22.5675364832709,-70.0183813516282,
83.730376405999));
#210823=CARTESIAN_POINT('Ctrl Pts',(-22.5675364832709,-70.1146905431934,
83.7745501571491));
#210824=CARTESIAN_POINT('Ctrl Pts',(-22.5675364832709,-70.2115077836584,
83.8173676866023));
#210825=CARTESIAN_POINT('Ctrl Pts',(-22.5675364832709,-70.394853554888,
83.8984525525004));
#210826=CARTESIAN_POINT('Ctrl Pts',(-22.5675364832709,-70.5800199760405,
83.9746766474746));
#210827=CARTESIAN_POINT('Ctrl Pts',(-22.5675364832709,-70.7669764966094,
84.0461131619166));
#210828=CARTESIAN_POINT('Ctrl Pts',(-22.5675364832709,-70.9546509613198,
84.1178240044584));
#210829=CARTESIAN_POINT('Ctrl Pts',(-22.5675364832709,-71.1441297243915,
84.1847105346889));
#210830=CARTESIAN_POINT('Ctrl Pts',(-22.5675364832709,-71.3354013965792,
84.2467978873676));
#210831=CARTESIAN_POINT('Ctrl Pts',(-22.5675364832709,-71.5266286583088,
84.3088708242798));
#210832=CARTESIAN_POINT('Ctrl Pts',(-22.5675364832709,-71.7196484304936,
84.3661469096111));
#210833=CARTESIAN_POINT('Ctrl Pts',(-22.5675364832709,-71.91446234413,84.4186009739624));
#210834=CARTESIAN_POINT('Ctrl Pts',(-22.5675364832709,-72.0106871486104,
84.4445097090839));
#210835=CARTESIAN_POINT('Ctrl Pts',(-22.5675364832709,-72.1073498268638,
84.4692412399597));
#210836=CARTESIAN_POINT('Ctrl Pts',(-22.5675364832709,-72.2044512501012,
84.4927878836045));
#210837=CARTESIAN_POINT('',(-22.5675364837383,-63.6650775904626,76.4088722770809));
#210838=CARTESIAN_POINT('Ctrl Pts',(-22.5673829558621,-63.6690417381459,
76.4209333437237));
#210839=CARTESIAN_POINT('Ctrl Pts',(-22.5674341318949,-63.6677182296578,
76.4169137400222));
#210840=CARTESIAN_POINT('Ctrl Pts',(-22.5674853079278,-63.6663968467197,
76.4128933831604));
#210841=CARTESIAN_POINT('Ctrl Pts',(-22.5675364839606,-63.665077590315,
76.4088722753856));
#210842=CARTESIAN_POINT('Ctrl Pts',(-22.5675364837383,-63.6650775904626,
76.4088722770809));
#210843=CARTESIAN_POINT('Ctrl Pts',(-22.586268085323,-63.4407556184205,
75.6674670848505));
#210844=CARTESIAN_POINT('Ctrl Pts',(-22.6057724255717,-63.2917836040619,
74.9097552024768));
#210845=CARTESIAN_POINT('Ctrl Pts',(-22.6429310858971,-63.1457829357986,
73.4058157535817));
#210846=CARTESIAN_POINT('Ctrl Pts',(-22.6606405257089,-63.1430629241209,
72.6625676820767));
#210847=CARTESIAN_POINT('Ctrl Pts',(-22.6917079591697,-63.2582592579212,
71.3752055764282));
#210848=CARTESIAN_POINT('Ctrl Pts',(-22.7050393165102,-63.3458208703714,
70.8282257981593));
#210849=CARTESIAN_POINT('Ctrl Pts',(-22.7250377762266,-63.5307031732887,
70.0378179720608));
#210850=CARTESIAN_POINT('Ctrl Pts',(-22.7314888115041,-63.5980781301251,
69.7878453758935));
#210851=CARTESIAN_POINT('Ctrl Pts',(-22.7709634204641,-64.0624224972185,
68.2665105161733));
#210852=CARTESIAN_POINT('Ctrl Pts',(-22.8027640999297,-64.6679194849621,
67.0581888191365));
#210853=CARTESIAN_POINT('Ctrl Pts',(-22.8537481998866,-65.9071091201683,
65.3669320568941));
#210854=CARTESIAN_POINT('Ctrl Pts',(-22.8725290298921,-66.4156702435171,
64.7993630234648));
#210855=CARTESIAN_POINT('Ctrl Pts',(-22.9239292449122,-67.9619180596299,
63.3764671688569));
#210856=CARTESIAN_POINT('Ctrl Pts',(-22.9604267297465,-69.2359429638033,
62.5103550986164));
#210857=CARTESIAN_POINT('Ctrl Pts',(-23.0202928869868,-71.5293846545732,
61.6432305647962));
#210858=CARTESIAN_POINT('Ctrl Pts',(-23.0392730866334,-72.2792099810029,
61.441436526952));
#210859=CARTESIAN_POINT('Ctrl Pts',(-23.0930290504121,-74.445504175765,
61.0779603516231));
#210860=CARTESIAN_POINT('Ctrl Pts',(-23.1299594944171,-76.0198431470072,
61.0706562319354));
#210861=CARTESIAN_POINT('Ctrl Pts',(-23.1905021030074,-78.4129038273741,
61.628264893377));
#210862=CARTESIAN_POINT('Ctrl Pts',(-23.2090908068358,-79.130062116161,
61.8685784075949));
#210863=CARTESIAN_POINT('Ctrl Pts',(-23.2410740979783,-80.3384165870843,
62.4056935084503));
#210864=CARTESIAN_POINT('Ctrl Pts',(-23.2545074008345,-80.8422218529907,
62.6745433313161));
#210865=CARTESIAN_POINT('Ctrl Pts',(-23.2863973120796,-81.9507079764464,
63.3759610656578));
#210866=CARTESIAN_POINT('Ctrl Pts',(-23.3048480792465,-82.5381646861957,
63.8305898999235));
#210867=CARTESIAN_POINT('Ctrl Pts',(-23.3350930669854,-83.4322130684856,
64.6654052881871));
#210868=CARTESIAN_POINT('Ctrl Pts',(-23.3469809107225,-83.7657290843186,
65.0169928637771));
#210869=CARTESIAN_POINT('Ctrl Pts',(-23.36893902758,-84.3520862167886,65.7159828751825));
#210870=CARTESIAN_POINT('Ctrl Pts',(-23.3790075514594,-84.609791987786,
66.0593191549823));
#210871=CARTESIAN_POINT('Ctrl Pts',(-23.3969914175803,-85.0270869734603,
66.6842488965303));
#210872=CARTESIAN_POINT('Ctrl Pts',(-23.4048424767611,-85.1948254259029,
66.9596772122972));
#210873=CARTESIAN_POINT('Ctrl Pts',(-23.4296186292686,-85.6824443991078,
67.839468895149));
#210874=CARTESIAN_POINT('Ctrl Pts',(-23.4468326360181,-85.9619375557439,
68.4665319016512));
#210875=CARTESIAN_POINT('Ctrl Pts',(-23.4767056660226,-86.3583903479144,
69.6102254268307));
#210876=CARTESIAN_POINT('Ctrl Pts',(-23.489401765161,-86.4979883598872,
70.1191785115426));
#210877=CARTESIAN_POINT('Ctrl Pts',(-23.5097178004072,-86.6694129472462,
70.9606073814973));
#210878=CARTESIAN_POINT('Ctrl Pts',(-23.5175437050304,-86.7219987057389,
71.2888547719625));
#210879=CARTESIAN_POINT('Ctrl Pts',(-23.5372801291869,-86.8169868755348,
72.1037210969665));
#210880=CARTESIAN_POINT('Ctrl Pts',(-23.5494001670538,-86.8428986535457,
72.5918834219198));
#210881=CARTESIAN_POINT('Ctrl Pts',(-23.5734791553164,-86.8347310175825,
73.555385132888));
#210882=CARTESIAN_POINT('Ctrl Pts',(-23.5854383058721,-86.8020866465661,
74.0310234500652));
#210883=CARTESIAN_POINT('Ctrl Pts',(-23.6099759330426,-86.674778997216,
75.0188565090374));
#210884=CARTESIAN_POINT('Ctrl Pts',(-23.6223585606802,-86.5746198606898,
75.5304187723396));
#210885=CARTESIAN_POINT('Ctrl Pts',(-23.6423017686355,-86.3580165407987,
76.347259459777));
#210886=CARTESIAN_POINT('Ctrl Pts',(-23.64996574602,-86.261790108825,76.65790185941));
#210887=CARTESIAN_POINT('Ctrl Pts',(-23.6713796367493,-85.9633916480115,
77.4955707899585));
#210888=CARTESIAN_POINT('Ctrl Pts',(-23.6855188631017,-85.7356046736506,
78.0123852988445));
#210889=CARTESIAN_POINT('Ctrl Pts',(-23.7091552450762,-85.2958981914814,
78.8448886272851));
#210890=CARTESIAN_POINT('Ctrl Pts',(-23.7186618439811,-85.1029821930297,
79.1713809851606));
#210891=CARTESIAN_POINT('Ctrl Pts',(-23.7427639934682,-84.5651742002068,
79.9901439374166));
#210892=CARTESIAN_POINT('Ctrl Pts',(-23.7568771368581,-84.1974308613908,
80.4674901565153));
#210893=CARTESIAN_POINT('Ctrl Pts',(-23.7781528652288,-83.5953254237176,
81.1368390030137));
#210894=CARTESIAN_POINT('Ctrl Pts',(-23.7852645329272,-83.3865629699947,
81.3518844373689));
#210895=CARTESIAN_POINT('Ctrl Pts',(-23.8051161905733,-82.7938308006642,
81.9171206383192));
#210896=CARTESIAN_POINT('Ctrl Pts',(-23.8181956316299,-82.3943211869376,
82.2499055715468));
#210897=CARTESIAN_POINT('Ctrl Pts',(-23.8397098155051,-81.7028715992346,
82.7532298694108));
#210898=CARTESIAN_POINT('Ctrl Pts',(-23.8481703871649,-81.4220441131709,
82.9399204995204));
#210899=CARTESIAN_POINT('Ctrl Pts',(-23.8711970500663,-80.6219484498624,
83.4243581702032));
#210900=CARTESIAN_POINT('Ctrl Pts',(-23.8852778638192,-80.0867100406283,
83.6958827846338));
#210901=CARTESIAN_POINT('Ctrl Pts',(-23.9073163037075,-79.2263152444547,
84.053440516101));
#210902=CARTESIAN_POINT('Ctrl Pts',(-23.9152294424715,-78.913127485958,
84.1683613902867));
#210903=CARTESIAN_POINT('Ctrl Pts',(-23.9341886438323,-78.167825248394,
84.4061841008917));
#210904=CARTESIAN_POINT('Ctrl Pts',(-23.9454211520972,-77.733419580155,
84.5174767713367));
#210905=CARTESIAN_POINT('Ctrl Pts',(-23.9652782132137,-76.9595352927832,
84.6696729400019));
#210906=CARTESIAN_POINT('Ctrl Pts',(-23.9738842404027,-76.6217327526431,
84.7210490326955));
#210907=CARTESIAN_POINT('Ctrl Pts',(-23.9968051979934,-75.6997099389066,
84.8210702035748));
#210908=CARTESIAN_POINT('Ctrl Pts',(-24.0107033113079,-75.1123315013629,
84.8413692782653));
#210909=CARTESIAN_POINT('Ctrl Pts',(-24.0340122827486,-74.1297607022727,
84.8028056628773));
#210910=CARTESIAN_POINT('Ctrl Pts',(-24.0434324047584,-73.7335916800172,
84.7673381145636));
#210911=CARTESIAN_POINT('Ctrl Pts',(-24.0646309551327,-72.8665015294452,
84.6450363719954));
#210912=CARTESIAN_POINT('Ctrl Pts',(-24.0765713079443,-72.399014171567,
84.5493528448018));
#210913=CARTESIAN_POINT('Ctrl Pts',(-24.0997554081118,-71.5089793165134,
84.310313566701));
#210914=CARTESIAN_POINT('Ctrl Pts',(-24.1108807937167,-71.0858335697661,
84.1706526421816));
#210915=CARTESIAN_POINT('Ctrl Pts',(-24.138533227618,-70.0268835211385,
83.7543074460251));
#210916=CARTESIAN_POINT('Ctrl Pts',(-24.1548409783302,-69.4039225594739,
83.4445873667952));
#210917=CARTESIAN_POINT('Ctrl Pts',(-24.1798141076876,-68.5144527788177,
82.9004178078518));
#210918=CARTESIAN_POINT('Ctrl Pts',(-24.1882658800564,-68.2242060734541,
82.704657018762));
#210919=CARTESIAN_POINT('Ctrl Pts',(-24.2064651621954,-67.6319243272847,
82.2650889548629));
#210920=CARTESIAN_POINT('Ctrl Pts',(-24.2162594926797,-67.3322371454712,
82.0184893106432));
#210921=CARTESIAN_POINT('Ctrl Pts',(-24.2503354667518,-66.3240452924204,
81.1023758653165));
#210922=CARTESIAN_POINT('Ctrl Pts',(-24.2734890978267,-65.6834341645618,
80.3575421127117));
#210923=CARTESIAN_POINT('Ctrl Pts',(-24.3359484974999,-64.2389187654643,
78.1900043195484));
#210924=CARTESIAN_POINT('Ctrl Pts',(-24.3698713517956,-63.7839507079286,
76.9116039690688));
#210925=CARTESIAN_POINT('Ctrl Pts',(-24.4133074766064,-63.3381100240567,
75.1700668662164));
#210926=CARTESIAN_POINT('Ctrl Pts',(-24.4319587440239,-63.2185309075811,
74.3940693434518));
#210927=CARTESIAN_POINT('Ctrl Pts',(-24.4613547807653,-63.1540310279044,
73.1896082034826));
#210928=CARTESIAN_POINT('Ctrl Pts',(-24.471852603356,-63.1544389514483,
72.7660588280706));
#210929=CARTESIAN_POINT('Ctrl Pts',(-24.5046971488066,-63.2278786888342,
71.441152956426));
#210930=CARTESIAN_POINT('Ctrl Pts',(-24.5265462495199,-63.381491704234,
70.5461094578424));
#210931=CARTESIAN_POINT('Ctrl Pts',(-24.5670051429739,-63.848113738075,
68.940460524804));
#210932=CARTESIAN_POINT('Ctrl Pts',(-24.5856817309163,-64.1348934482634,
68.2206283273269));
#210933=CARTESIAN_POINT('Ctrl Pts',(-24.6232006790464,-64.8387020839017,
66.8653478737878));
#210934=CARTESIAN_POINT('Ctrl Pts',(-24.641661123262,-65.2512151410827,
66.2297978498682));
#210935=CARTESIAN_POINT('Ctrl Pts',(-24.688246890458,-66.4376319825064,
64.7326308652929));
#210936=CARTESIAN_POINT('Ctrl Pts',(-24.7260382386131,-67.5561267157986,
63.5847792685608));
#210937=CARTESIAN_POINT('Ctrl Pts',(-24.7917113773772,-69.8951100285009,
62.2801640674082));
#210938=CARTESIAN_POINT('Ctrl Pts',(-24.8105835909978,-70.6016469499005,
61.9711661347996));
#210939=CARTESIAN_POINT('Ctrl Pts',(-24.8476505405662,-72.0487458576382,
61.4982879163503));
#210940=CARTESIAN_POINT('Ctrl Pts',(-24.8656179042792,-72.7881859508202,
61.3322689755976));
#210941=CARTESIAN_POINT('Ctrl Pts',(-24.9052918234948,-74.4024570724264,
61.1330685277049));
#210942=CARTESIAN_POINT('Ctrl Pts',(-24.9268693700248,-75.2747719906355,
61.1221140290983));
#210943=CARTESIAN_POINT('Ctrl Pts',(-24.9577085382441,-76.5262184018719,
61.2424810283113));
#210944=CARTESIAN_POINT('Ctrl Pts',(-24.9672177195347,-76.9128067571203,
61.298875033784));
#210945=CARTESIAN_POINT('Ctrl Pts',(-24.9905520650339,-77.8648755091039,
61.4862146028854));
#210946=CARTESIAN_POINT('Ctrl Pts',(-25.0042103174987,-78.4242489456068,
61.6397751316609));
#210947=CARTESIAN_POINT('Ctrl Pts',(-25.033528821721,-79.5538256273119,
62.0429563473436));
#210948=CARTESIAN_POINT('Ctrl Pts',(-25.04892536006,-80.1189290269644,62.296315326189));
#210949=CARTESIAN_POINT('Ctrl Pts',(-25.0800666050373,-81.2227434998887,
62.8976245618864));
#210950=CARTESIAN_POINT('Ctrl Pts',(-25.0957726872482,-81.759935237262,
63.2487373897805));
#210951=CARTESIAN_POINT('Ctrl Pts',(-25.1193718523509,-82.5435011709395,
63.8566578124951));
#210952=CARTESIAN_POINT('Ctrl Pts',(-25.1276624343038,-82.8120640683606,
64.0849197521116));
#210953=CARTESIAN_POINT('Ctrl Pts',(-25.1454609563522,-83.3545132896373,
64.5900982370671));
#210954=CARTESIAN_POINT('Ctrl Pts',(-25.1550148296105,-83.625759296159,
64.869428342891));
#210955=CARTESIAN_POINT('Ctrl Pts',(-25.1821367707944,-84.3482342239114,
65.6906711368966));
#210956=CARTESIAN_POINT('Ctrl Pts',(-25.1999107406064,-84.7667054739517,
66.2617692430849));
#210957=CARTESIAN_POINT('Ctrl Pts',(-25.2283952223508,-85.3696652829342,
67.2584876520549));
#210958=CARTESIAN_POINT('Ctrl Pts',(-25.2393089263843,-85.5849431538456,
67.665653210413));
#210959=CARTESIAN_POINT('Ctrl Pts',(-25.2610572632069,-85.9669200722996,
68.5030414663968));
#210960=CARTESIAN_POINT('Ctrl Pts',(-25.2719955468722,-86.1331191980178,
68.9323993214247));
#210961=CARTESIAN_POINT('Ctrl Pts',(-25.2937880673866,-86.4034375703859,
69.7767493402283));
#210962=CARTESIAN_POINT('Ctrl Pts',(-25.3044379286781,-86.5109674922512,
70.1883156831867));
#210963=CARTESIAN_POINT('Ctrl Pts',(-25.3293736091068,-86.7108551138341,
71.1638320986707));
#210964=CARTESIAN_POINT('Ctrl Pts',(-25.343638785203,-86.7852594491684,
71.7315450267012));
#210965=CARTESIAN_POINT('Ctrl Pts',(-25.3658368888779,-86.8394224130096,
72.6541834421136));
#210966=CARTESIAN_POINT('Ctrl Pts',(-25.374145029744,-86.8444614999076,
73.0076890856007));
#210967=CARTESIAN_POINT('Ctrl Pts',(-25.3932547504683,-86.8197084010493,
73.8167754615253));
#210968=CARTESIAN_POINT('Ctrl Pts',(-25.4041146979202,-86.7793325444496,
74.2716084565836));
#210969=CARTESIAN_POINT('Ctrl Pts',(-25.424894620039,-86.6553428033959,
75.1053687246365));
#210970=CARTESIAN_POINT('Ctrl Pts',(-25.4345780693059,-86.5799035844431,
75.483491530525));
#210971=CARTESIAN_POINT('Ctrl Pts',(-25.4567619973944,-86.3652872626109,
76.3401422706028));
#210972=CARTESIAN_POINT('Ctrl Pts',(-25.4692500578771,-86.2138979984785,
76.8156577038014));
#210973=CARTESIAN_POINT('Ctrl Pts',(-25.4890094659494,-85.9180320095654,
77.5769828960217));
#210974=CARTESIAN_POINT('Ctrl Pts',(-25.4965644957774,-85.7906708954485,
77.8694937917343));
#210975=CARTESIAN_POINT('Ctrl Pts',(-25.5177272011171,-85.4002237205209,
78.675968320559));
#210976=CARTESIAN_POINT('Ctrl Pts',(-25.5313223378869,-85.1104844963385,
79.1778737046409));
#210977=CARTESIAN_POINT('Ctrl Pts',(-25.5539619675576,-84.5929121635644,
79.93673654874));
#210978=CARTESIAN_POINT('Ctrl Pts',(-25.5624776214518,-84.3898698056711,
80.2082748200738));
#210979=CARTESIAN_POINT('Ctrl Pts',(-25.583850319648,-83.8526286867851,
80.8660090615761));
#210980=CARTESIAN_POINT('Ctrl Pts',(-25.5966963903215,-83.5041146448396,
81.2405495882105));
#210981=CARTESIAN_POINT('Ctrl Pts',(-25.6174987374248,-82.8801328369273,
81.8305356652936));
#210982=CARTESIAN_POINT('Ctrl Pts',(-25.6257626286481,-82.6166528461616,
82.0587208875653));
#210983=CARTESIAN_POINT('Ctrl Pts',(-25.6481489502375,-81.8749389306029,
82.6461857161961));
#210984=CARTESIAN_POINT('Ctrl Pts',(-25.6622524342849,-81.3776042707483,
82.982588201651));
#210985=CARTESIAN_POINT('Ctrl Pts',(-25.6849535707228,-80.5776536122919,
83.4376350608617));
#210986=CARTESIAN_POINT('Ctrl Pts',(-25.6930171765533,-80.2925384126093,
83.5846073202146));
#210987=CARTESIAN_POINT('Ctrl Pts',(-25.7146507220582,-79.5134293397299,
83.9469660150489));
#210988=CARTESIAN_POINT('Ctrl Pts',(-25.7281391359254,-79.0093860434919,
84.1408019798079));
#210989=CARTESIAN_POINT('Ctrl Pts',(-25.7520876074811,-78.0611832160611,
84.4337245706684));
#210990=CARTESIAN_POINT('Ctrl Pts',(-25.7628108659822,-77.6200926928871,
84.5429585790474));
#210991=CARTESIAN_POINT('Ctrl Pts',(-25.7851622316925,-76.6949087349468,
84.7165901495161));
#210992=CARTESIAN_POINT('Ctrl Pts',(-25.7968063426044,-76.209853352635,
84.7770486933715));
#210993=CARTESIAN_POINT('Ctrl Pts',(-25.8166416512073,-75.4074932820353,
84.8260692378726));
#210994=CARTESIAN_POINT('Ctrl Pts',(-25.8245878850808,-75.0915856903094,
84.8324891107674));
#210995=CARTESIAN_POINT('Ctrl Pts',(-25.8461263984118,-74.2351689420447,
84.8155658720594));
#210996=CARTESIAN_POINT('Ctrl Pts',(-25.8595502609578,-73.6951265588063,
84.7677371052758));
#210997=CARTESIAN_POINT('Ctrl Pts',(-25.8870929365112,-72.5668908757251,
84.590167107365));
#210998=CARTESIAN_POINT('Ctrl Pts',(-25.9012958491269,-71.9799307868807,
84.4518600552353));
#210999=CARTESIAN_POINT('Ctrl Pts',(-25.9262597884433,-70.9876187870929,
84.1367233640308));
#211000=CARTESIAN_POINT('Ctrl Pts',(-25.9369484716105,-70.5754337900106,
83.9800739201598));
#211001=CARTESIAN_POINT('Ctrl Pts',(-25.9593084055028,-69.7555554483605,
83.6136503722819));
#211002=CARTESIAN_POINT('Ctrl Pts',(-25.9708645623636,-69.3496943959058,
83.4029204272594));
#211003=CARTESIAN_POINT('Ctrl Pts',(-25.993834366265,-68.5485247822595,
82.9265531223753));
#211004=CARTESIAN_POINT('Ctrl Pts',(-26.0053100341751,-68.1543368512848,
82.6589885236473));
#211005=CARTESIAN_POINT('Ctrl Pts',(-26.0343820127018,-67.1941352451247,
81.9199778940686));
#211006=CARTESIAN_POINT('Ctrl Pts',(-26.0518964723241,-66.6521974956702,
81.4170463576902));
#211007=CARTESIAN_POINT('Ctrl Pts',(-26.0820442935133,-65.834173220253,
80.5001478589804));
#211008=CARTESIAN_POINT('Ctrl Pts',(-26.0944271911147,-65.5306940758781,
80.1129252510169));
#211009=CARTESIAN_POINT('Ctrl Pts',(-26.1225191227804,-64.8854521730426,
79.1752815467207));
#211010=CARTESIAN_POINT('Ctrl Pts',(-26.1381663634804,-64.5620635789478,
78.6116580075701));
#211011=CARTESIAN_POINT('Ctrl Pts',(-26.1721088657882,-63.9623371723801,
77.3370325344058));
#211012=CARTESIAN_POINT('Ctrl Pts',(-26.1904008122124,-63.7041000312099,
76.6173315306627));
#211013=CARTESIAN_POINT('Ctrl Pts',(-26.2163069038114,-63.4471831016142,
75.5971963120756));
#211014=CARTESIAN_POINT('Ctrl Pts',(-26.2235318340176,-63.3868135706353,
75.3127304873911));
#211015=CARTESIAN_POINT('Ctrl Pts',(-26.2587554148368,-63.141968335338,
73.904777802475));
#211016=CARTESIAN_POINT('Ctrl Pts',(-26.2862238156631,-63.1094668467566,
72.754329610765));
#211017=CARTESIAN_POINT('Ctrl Pts',(-26.3415801754294,-63.3707065358412,
70.4878602924608));
#211018=CARTESIAN_POINT('Ctrl Pts',(-26.3693494802877,-63.6652819705078,
69.3856928759218));
#211019=CARTESIAN_POINT('Ctrl Pts',(-26.3971183084764,-64.1119392449378,
68.3407934129424));
#211020=CARTESIAN_POINT('Ctrl Pts',(-31.6489087198709,-79.9040287823937,
60.8783100640841));
#211021=CARTESIAN_POINT('Ctrl Pts',(-31.6814645153009,-81.2696674810732,
61.4313085050615));
#211022=CARTESIAN_POINT('Ctrl Pts',(-31.7465761061609,-83.811729992399,
63.0035716608669));
#211023=CARTESIAN_POINT('Ctrl Pts',(-31.8442434924509,-86.6262501677223,
66.49395799585));
#211024=CARTESIAN_POINT('Ctrl Pts',(-31.9419108787409,-88.1228094499778,
70.7205438274274));
#211025=CARTESIAN_POINT('Ctrl Pts',(-32.0395782650309,-88.1318596833692,
75.2042647157331));
#211026=CARTESIAN_POINT('Ctrl Pts',(-32.1372456513209,-86.6523499320974,
79.4368608152641));
#211027=CARTESIAN_POINT('Ctrl Pts',(-32.2349130376109,-83.8519959181997,
82.9385512545613));
#211028=CARTESIAN_POINT('Ctrl Pts',(-32.3325804239009,-80.0482284232973,
85.3124031224554));
#211029=CARTESIAN_POINT('Ctrl Pts',(-32.4302478101809,-75.6722218896999,
86.2893299487034));
#211030=CARTESIAN_POINT('Ctrl Pts',(-32.5279151964709,-71.2200159883432,
85.7585926810093));
#211031=CARTESIAN_POINT('Ctrl Pts',(-32.6255825827609,-67.1962880910714,
83.7803527627688));
#211032=CARTESIAN_POINT('Ctrl Pts',(-32.7232499690509,-64.0571456387238,
80.5788524819327));
#211033=CARTESIAN_POINT('Ctrl Pts',(-32.8209173553409,-62.1584243900869,
76.5169961329518));
#211034=CARTESIAN_POINT('Ctrl Pts',(-32.9185847416309,-61.7153528413655,
72.0552131952207));
#211035=CARTESIAN_POINT('Ctrl Pts',(-33.0162521279209,-62.7781551230735,
67.6992666057196));
#211036=CARTESIAN_POINT('Ctrl Pts',(-33.1139195142109,-65.2263578703911,
63.9429222806304));
#211037=CARTESIAN_POINT('Ctrl Pts',(-33.2115869005009,-68.7824464151142,
61.2119785531442));
#211038=CARTESIAN_POINT('Ctrl Pts',(-33.3092542867909,-73.0433223072712,
59.8160000388975));
#211039=CARTESIAN_POINT('Ctrl Pts',(-33.4069216730809,-77.5259963169692,
59.9132271101948));
#211040=CARTESIAN_POINT('Ctrl Pts',(-33.5045890593709,-81.7223374113863,
61.4926386461447));
#211041=CARTESIAN_POINT('Ctrl Pts',(-33.6022564456609,-85.1566716669334,
64.3752013257362));
#211042=CARTESIAN_POINT('Ctrl Pts',(-33.6999238319509,-87.43970202375,68.2341638508803));
#211043=CARTESIAN_POINT('Ctrl Pts',(-33.7975912182409,-88.3126368385637,
72.632095659094));
#211044=CARTESIAN_POINT('Ctrl Pts',(-33.8952586045309,-87.6765250683029,
77.0704716229308));
#211045=CARTESIAN_POINT('Ctrl Pts',(-33.9929259908209,-85.6034728108319,
81.0461820900503));
#211046=CARTESIAN_POINT('Ctrl Pts',(-34.0905933771109,-82.3284697580989,
84.1085625995896));
#211047=CARTESIAN_POINT('Ctrl Pts',(-34.1882607634009,-78.2227520696129,
85.9104787028144));
#211048=CARTESIAN_POINT('Ctrl Pts',(-34.2859281496909,-73.7517211029078,
86.2476751965479));
#211049=CARTESIAN_POINT('Ctrl Pts',(-34.3835955359809,-69.4221881001095,
85.0819293587689));
#211050=CARTESIAN_POINT('Ctrl Pts',(-34.4812629222709,-65.7249248799056,
82.545383664097));
#211051=CARTESIAN_POINT('Ctrl Pts',(-34.5789303085609,-63.0790326695276,
78.9255668466803));
#211052=CARTESIAN_POINT('Ctrl Pts',(-34.6765976948509,-61.7844351169188,
74.6328012395937));
#211053=CARTESIAN_POINT('Ctrl Pts',(-34.7742650811409,-61.9878806115566,
70.1536909137268));
#211054=CARTESIAN_POINT('Ctrl Pts',(-34.8719324674309,-63.666307701945,
65.995962942479));
#211055=CARTESIAN_POINT('Ctrl Pts',(-34.9695998537209,-66.6294592136506,
62.6309142802354));
#211056=CARTESIAN_POINT('Ctrl Pts',(-35.0672672400109,-70.5414487461066,
60.4399881567566));
#211057=CARTESIAN_POINT('Ctrl Pts',(-35.1649346263009,-74.9588348897375,
59.6715357908676));
#211058=CARTESIAN_POINT('Ctrl Pts',(-35.2626020125909,-79.3808872816728,
60.4126646754531));
#211059=CARTESIAN_POINT('Ctrl Pts',(-35.3602693988809,-83.3063466190444,
62.5793645557408));
#211060=CARTESIAN_POINT('Ctrl Pts',(-35.4579367851709,-86.2902446299875,
65.9260303652965));
#211061=CARTESIAN_POINT('Ctrl Pts',(-35.5556041714609,-87.994343206,70.0733026524509));
#211062=CARTESIAN_POINT('Ctrl Pts',(-35.6532715577509,-88.2254751955924,
74.5510696611245));
#211063=CARTESIAN_POINT('Ctrl Pts',(-35.7509389440409,-86.9574407599487,
78.8517565888795));
#211064=CARTESIAN_POINT('Ctrl Pts',(-35.8486063303309,-84.3339772411099,
82.4878614479098));
#211065=CARTESIAN_POINT('Ctrl Pts',(-35.9462737166209,-80.6524658951112,
85.0472155832));
#211066=CARTESIAN_POINT('Ctrl Pts',(-36.0439411029109,-76.3302224041847,
86.2397048224279));
#211067=CARTESIAN_POINT('Ctrl Pts',(-36.1416084892009,-71.857192288432,
85.9301552074926));
#211068=CARTESIAN_POINT('Ctrl Pts',(-36.2392758754909,-67.7404134024109,
84.1536555637811));
#211069=CARTESIAN_POINT('Ctrl Pts',(-36.3369432617809,-64.4465409395824,
81.1115800257429));
#211070=CARTESIAN_POINT('Ctrl Pts',(-36.4346106480709,-62.3489499909946,
77.1487613832986));
#211071=CARTESIAN_POINT('Ctrl Pts',(-36.5322780343609,-61.6854118183574,
72.7144027516668));
#211072=CARTESIAN_POINT('Ctrl Pts',(-36.6299454206509,-62.5311414241959,
68.3111584007035));
#211073=CARTESIAN_POINT('Ctrl Pts',(-36.7276128069509,-64.7902715968898,
64.4381556582015));
#211074=CARTESIAN_POINT('Ctrl Pts',(-36.8252801932409,-68.206719885141,
61.534416607706));
#211075=CARTESIAN_POINT('Ctrl Pts',(-36.9229475795309,-72.3932166837339,
59.9290929831488));
#211076=CARTESIAN_POINT('Ctrl Pts',(-37.0206149658209,-76.875203961106,
59.8041553558837));
#211077=CARTESIAN_POINT('Ctrl Pts',(-37.1182823521109,-81.1446285386002,
61.1737659619934));
#211078=CARTESIAN_POINT('Ctrl Pts',(-37.2159497384009,-84.7175321175373,
63.8826733471557));
#211079=CARTESIAN_POINT('Ctrl Pts',(-37.3136171246909,-87.1889103282383,
67.6238108193034));
#211080=CARTESIAN_POINT('Ctrl Pts',(-37.4112845109809,-88.2786209412064,
71.9731037866268));
#211081=CARTESIAN_POINT('Ctrl Pts',(-37.5089518972709,-87.8631423512599,
76.4375406365594));
#211082=CARTESIAN_POINT('Ctrl Pts',(-37.6066192835609,-85.9895636692369,
80.5110572786137));
#211083=CARTESIAN_POINT('Ctrl Pts',(-37.7042866698509,-82.8702903713335,
83.7319036844191));
#211084=CARTESIAN_POINT('Ctrl Pts',(-37.8019540561409,-78.8588051875596,
85.7349781226078));
#211085=CARTESIAN_POINT('Ctrl Pts',(-37.8670656470009,-75.8930709812184,
86.1071526244662));
#211086=CARTESIAN_POINT('Ctrl Pts',(-37.8996214424309,-74.4211620580609,
86.0418804791265));
#211087=CARTESIAN_POINT('Ctrl Pts',(-31.8730368301509,-79.7424307674282,
61.2773790062616));
#211088=CARTESIAN_POINT('Ctrl Pts',(-31.9055926255809,-81.0630688120212,
61.8121549909075));
#211089=CARTESIAN_POINT('Ctrl Pts',(-31.9707042164409,-83.5213650417874,
63.3326087841966));
#211090=CARTESIAN_POINT('Ctrl Pts',(-32.0683716027309,-86.2431408851346,
66.7079795823174));
#211091=CARTESIAN_POINT('Ctrl Pts',(-32.1660389890109,-87.6903854059918,
70.7952905623852));
#211092=CARTESIAN_POINT('Ctrl Pts',(-32.2637063753009,-87.6991374152512,
75.1312634607482));
#211093=CARTESIAN_POINT('Ctrl Pts',(-32.3613737615909,-86.2683806076395,
79.2243866578649));
#211094=CARTESIAN_POINT('Ctrl Pts',(-32.4590411478809,-83.5603041210376,
82.610689066389));
#211095=CARTESIAN_POINT('Ctrl Pts',(-32.5567085341709,-79.8818787282825,
84.9063175455787));
#211096=CARTESIAN_POINT('Ctrl Pts',(-32.6543759204609,-75.6500707711405,
85.8510525877097));
#211097=CARTESIAN_POINT('Ctrl Pts',(-32.7520433067509,-71.3445743749261,
85.3378042240803));
#211098=CARTESIAN_POINT('Ctrl Pts',(-32.8497106930409,-67.4534367355484,
83.4247514525908));
#211099=CARTESIAN_POINT('Ctrl Pts',(-32.9473780793309,-64.4177355988012,
80.3287473083499));
#211100=CARTESIAN_POINT('Ctrl Pts',(-33.0450454656209,-62.5815811902788,
76.400737629567));
#211101=CARTESIAN_POINT('Ctrl Pts',(-33.1427128519109,-62.1531097766604,
72.0859797803774));
#211102=CARTESIAN_POINT('Ctrl Pts',(-33.2403802382009,-63.1808904982033,
67.8735707501784));
#211103=CARTESIAN_POINT('Ctrl Pts',(-33.3380476244909,-65.5484198396858,
64.2410058345145));
#211104=CARTESIAN_POINT('Ctrl Pts',(-33.4357150107809,-68.9873278221854,
61.6000524200778));
#211105=CARTESIAN_POINT('Ctrl Pts',(-33.5333823970709,-73.1077989335492,
60.2500743203519));
#211106=CARTESIAN_POINT('Ctrl Pts',(-33.6310497833609,-77.4427594501453,
60.3440975560973));
#211107=CARTESIAN_POINT('Ctrl Pts',(-33.7287171696509,-81.5008223204608,
61.871464175445));
#211108=CARTESIAN_POINT('Ctrl Pts',(-33.8263845559409,-84.8219880725154,
64.6590403800946));
#211109=CARTESIAN_POINT('Ctrl Pts',(-33.9240519422309,-87.0297877995459,
68.390842011297));
#211110=CARTESIAN_POINT('Ctrl Pts',(-34.0217193285209,-87.8739575847217,
72.6438527593594));
#211111=CARTESIAN_POINT('Ctrl Pts',(-34.1193867148109,-87.2588070289994,
76.9359749434431));
#211112=CARTESIAN_POINT('Ctrl Pts',(-34.2170541010909,-85.2540661833469,
80.7806774275269));
#211113=CARTESIAN_POINT('Ctrl Pts',(-34.3147214873809,-82.0869813374197,
83.7421460881762));
#211114=CARTESIAN_POINT('Ctrl Pts',(-34.4123888736709,-78.1165556420916,
85.4846852834909));
#211115=CARTESIAN_POINT('Ctrl Pts',(-34.5100562599609,-73.7928545058452,
85.8107704468362));
#211116=CARTESIAN_POINT('Ctrl Pts',(-34.6077236462509,-69.6059886793678,
84.6834383749047));
#211117=CARTESIAN_POINT('Ctrl Pts',(-34.7053910325409,-66.0305580224903,
82.2304771711338));
#211118=CARTESIAN_POINT('Ctrl Pts',(-34.8030584188309,-63.4718534996216,
78.729940895939));
#211119=CARTESIAN_POINT('Ctrl Pts',(-34.9007258051209,-62.2199156466047,
74.5786309025152));
#211120=CARTESIAN_POINT('Ctrl Pts',(-34.9983931914109,-62.4166571862875,
70.2471166389011));
#211121=CARTESIAN_POINT('Ctrl Pts',(-35.0960605777009,-64.0397765902539,
66.2263945085208));
#211122=CARTESIAN_POINT('Ctrl Pts',(-35.1937279639909,-66.9052860562882,
62.9722312444263));
#211123=CARTESIAN_POINT('Ctrl Pts',(-35.2913953502809,-70.6883673438916,
60.8535007234066));
#211124=CARTESIAN_POINT('Ctrl Pts',(-35.3890627365809,-74.9601913662926,
60.1103704717333));
#211125=CARTESIAN_POINT('Ctrl Pts',(-35.4867301228709,-79.2365278743448,
60.8270776080123));
#211126=CARTESIAN_POINT('Ctrl Pts',(-35.5843975091609,-83.032635108598,
62.9223801912564));
#211127=CARTESIAN_POINT('Ctrl Pts',(-35.6820648954509,-85.9182074332976,
66.1587663561375));
#211128=CARTESIAN_POINT('Ctrl Pts',(-35.7797322817409,-87.566152393697,
70.1693773391154));
#211129=CARTESIAN_POINT('Ctrl Pts',(-35.8773996680309,-87.7896681003677,
74.4995925506423));
#211130=CARTESIAN_POINT('Ctrl Pts',(-35.9750670543209,-86.5634180540064,
78.6585628406411));
#211131=CARTESIAN_POINT('Ctrl Pts',(-36.0727344406109,-84.0264031503354,
82.1748504323777));
#211132=CARTESIAN_POINT('Ctrl Pts',(-36.1704018269009,-80.4662053104341,
84.6498684909032));
#211133=CARTESIAN_POINT('Ctrl Pts',(-36.2680692131909,-76.2863887911529,
85.8030627132264));
#211134=CARTESIAN_POINT('Ctrl Pts',(-36.3657365994809,-71.9607543820079,
85.5037134061586));
#211135=CARTESIAN_POINT('Ctrl Pts',(-36.4634039857709,-67.9796319787588,
83.7857531448031));
#211136=CARTESIAN_POINT('Ctrl Pts',(-36.5610713720609,-64.7942995092932,
80.8439203643351));
#211137=CARTESIAN_POINT('Ctrl Pts',(-36.6587387583509,-62.7658285737666,
77.0116848923228));
#211138=CARTESIAN_POINT('Ctrl Pts',(-36.7564061446409,-62.1241553730382,
72.723447660932));
#211139=CARTESIAN_POINT('Ctrl Pts',(-36.8540735309309,-62.9420164178251,
68.4652994295259));
#211140=CARTESIAN_POINT('Ctrl Pts',(-36.9517409172209,-65.126703521839,
64.7199202355243));
#211141=CARTESIAN_POINT('Ctrl Pts',(-37.0494083035109,-68.4305726866551,
61.9118654657189));
#211142=CARTESIAN_POINT('Ctrl Pts',(-37.1470756898009,-72.479115651301,
60.359440615331));
#211143=CARTESIAN_POINT('Ctrl Pts',(-37.2447430760909,-76.8134120648424,
60.238619944442));
#211144=CARTESIAN_POINT('Ctrl Pts',(-37.3424104623809,-80.9421501644669,
61.5630990137955));
#211145=CARTESIAN_POINT('Ctrl Pts',(-37.4400778486709,-84.397319090609,
64.1827422295159));
#211146=CARTESIAN_POINT('Ctrl Pts',(-37.5377452349609,-86.7872602154302,
67.8006013898866));
#211147=CARTESIAN_POINT('Ctrl Pts',(-37.6354126212509,-87.8410625823901,
72.0065760486924));
#211148=CARTESIAN_POINT('Ctrl Pts',(-37.7330800075509,-87.4392748817876,
76.3239003581206));
#211149=CARTESIAN_POINT('Ctrl Pts',(-37.8307473938409,-85.6274345396819,
80.2631860989099));
#211150=CARTESIAN_POINT('Ctrl Pts',(-37.9284147801309,-82.6109478271435,
83.3778988728008));
#211151=CARTESIAN_POINT('Ctrl Pts',(-38.0260821664209,-78.7316494782208,
85.3149678148182));
#211152=CARTESIAN_POINT('Ctrl Pts',(-38.0911937572809,-75.8636424227415,
85.6748783876891));
#211153=CARTESIAN_POINT('Ctrl Pts',(-38.1237495527109,-74.4402359800407,
85.6117570961772));
#211154=CARTESIAN_POINT('Ctrl Pts',(-32.0971649404209,-79.5808327524621,
61.6764479484404));
#211155=CARTESIAN_POINT('Ctrl Pts',(-32.1297207358509,-80.8564701429687,
62.1930014767526));
#211156=CARTESIAN_POINT('Ctrl Pts',(-32.1948323267109,-83.2310000911753,
63.6616459075254));
#211157=CARTESIAN_POINT('Ctrl Pts',(-32.2924997130009,-85.8600316025557,
66.9220011687801));
#211158=CARTESIAN_POINT('Ctrl Pts',(-32.3901670992909,-87.2579613620154,
70.8700372973401));
#211159=CARTESIAN_POINT('Ctrl Pts',(-32.4878344855809,-87.2664151471337,
75.0582622057642));
#211160=CARTESIAN_POINT('Ctrl Pts',(-32.5855018718709,-85.8844112831762,
79.0119125004583));
#211161=CARTESIAN_POINT('Ctrl Pts',(-32.6831692581609,-83.2686123238737,
82.2828268782174));
#211162=CARTESIAN_POINT('Ctrl Pts',(-32.7808366444509,-79.7155290332633,
84.5002319687039));
#211163=CARTESIAN_POINT('Ctrl Pts',(-32.8785040307409,-75.6279196525717,
85.412775226709));
#211164=CARTESIAN_POINT('Ctrl Pts',(-32.9761714170309,-71.4691327614987,
84.9170157671447));
#211165=CARTESIAN_POINT('Ctrl Pts',(-33.0738388033209,-67.7105853800127,
83.0691501424084));
#211166=CARTESIAN_POINT('Ctrl Pts',(-33.1715061896109,-64.7783255588649,
80.0786421347598));
#211167=CARTESIAN_POINT('Ctrl Pts',(-33.2691735759009,-63.0047379904651,
76.2844791261684));
#211168=CARTESIAN_POINT('Ctrl Pts',(-33.3668409621909,-62.5908667119491,
72.1167463655193));
#211169=CARTESIAN_POINT('Ctrl Pts',(-33.4645083484809,-63.5836258733412,
68.0478748946176));
#211170=CARTESIAN_POINT('Ctrl Pts',(-33.5621757347709,-65.8704818089924,
64.5390893883721));
#211171=CARTESIAN_POINT('Ctrl Pts',(-33.6598431210609,-69.1922092292778,
61.9881262869918));
#211172=CARTESIAN_POINT('Ctrl Pts',(-33.7575105073509,-73.1722755598568,
60.6841486018049));
#211173=CARTESIAN_POINT('Ctrl Pts',(-33.8551778936409,-77.3595225833569,
60.7749680020175));
#211174=CARTESIAN_POINT('Ctrl Pts',(-33.9528452799309,-81.2793072295691,
62.2502897047617));
#211175=CARTESIAN_POINT('Ctrl Pts',(-34.0505126662209,-84.4873044781106,
64.9428794344855));
#211176=CARTESIAN_POINT('Ctrl Pts',(-34.1481800525109,-86.6198735753575,
68.5475201717516));
#211177=CARTESIAN_POINT('Ctrl Pts',(-34.2458474388009,-87.4352783308858,
72.6556098596655));
#211178=CARTESIAN_POINT('Ctrl Pts',(-34.3435148250909,-86.8410889896759,
76.8014782640016));
#211179=CARTESIAN_POINT('Ctrl Pts',(-34.4411822113809,-84.9046595558289,
80.5151727650388));
#211180=CARTESIAN_POINT('Ctrl Pts',(-34.5388495976709,-81.8454929166992,
83.3757295768015));
#211181=CARTESIAN_POINT('Ctrl Pts',(-34.6365169839609,-78.0103592145147,
85.0588918641796));
#211182=CARTESIAN_POINT('Ctrl Pts',(-34.7341843702509,-73.8339879087212,
85.3738656971173));
#211183=CARTESIAN_POINT('Ctrl Pts',(-34.8318517565409,-69.7897892585688,
84.2849473910144));
#211184=CARTESIAN_POINT('Ctrl Pts',(-34.9295191428309,-66.3361911650335,
81.9155706781227));
#211185=CARTESIAN_POINT('Ctrl Pts',(-35.0271865291209,-63.8646743296805,
78.5343149451387));
#211186=CARTESIAN_POINT('Ctrl Pts',(-35.1248539154109,-62.6553961762831,
74.5244605653661));
#211187=CARTESIAN_POINT('Ctrl Pts',(-35.2225213017009,-62.8454337610229,
70.3405423640074));
#211188=CARTESIAN_POINT('Ctrl Pts',(-35.3201886879909,-64.4132454785962,
66.4568260744839));
#211189=CARTESIAN_POINT('Ctrl Pts',(-35.4178560742809,-67.181112898978,
63.3135482085524));
#211190=CARTESIAN_POINT('Ctrl Pts',(-35.5155234605709,-70.8352859417533,
61.2670132900357));
#211191=CARTESIAN_POINT('Ctrl Pts',(-35.6131908468609,-74.9615478429283,
60.5492051525981));
#211192=CARTESIAN_POINT('Ctrl Pts',(-35.7108582331509,-79.0921684670951,
61.2414905405986));
#211193=CARTESIAN_POINT('Ctrl Pts',(-35.8085256194409,-82.7589235982165,
63.2653958268243));
#211194=CARTESIAN_POINT('Ctrl Pts',(-35.9061930057309,-85.5461702366482,
66.3915023470505));
#211195=CARTESIAN_POINT('Ctrl Pts',(-36.0038603920209,-87.1379615814165,
70.2654520258604));
#211196=CARTESIAN_POINT('Ctrl Pts',(-36.1015277783109,-87.3538610051255,
74.4481154402485));
#211197=CARTESIAN_POINT('Ctrl Pts',(-36.1991951646009,-86.1693953480258,
78.4653690924801));
#211198=CARTESIAN_POINT('Ctrl Pts',(-36.2968625508909,-83.7188290595022,
81.8618394169131));
#211199=CARTESIAN_POINT('Ctrl Pts',(-36.3945299371809,-80.2799447256819,
84.2525213986484));
#211200=CARTESIAN_POINT('Ctrl Pts',(-36.4921973234709,-76.2425551780386,
85.3664206040374));
#211201=CARTESIAN_POINT('Ctrl Pts',(-36.5898647097609,-72.064316475499,
85.0772716047946));
#211202=CARTESIAN_POINT('Ctrl Pts',(-36.6875320960509,-68.2188505550257,
83.4178507257861));
#211203=CARTESIAN_POINT('Ctrl Pts',(-36.7851994823409,-65.1420580789654,
80.57626070286));
#211204=CARTESIAN_POINT('Ctrl Pts',(-36.8828668686309,-63.1827071565181,
76.8746084012712));
#211205=CARTESIAN_POINT('Ctrl Pts',(-36.9805342549209,-62.5628989277203,
72.7324925701221));
#211206=CARTESIAN_POINT('Ctrl Pts',(-37.0782016412109,-63.3528914114806,
68.6194404582811));
#211207=CARTESIAN_POINT('Ctrl Pts',(-37.1758690275009,-65.4631354468294,
65.0016848127869));
#211208=CARTESIAN_POINT('Ctrl Pts',(-37.2735364137909,-68.6544254882255,
62.2893143236977));
#211209=CARTESIAN_POINT('Ctrl Pts',(-37.3712038000809,-72.5650146189264,
60.7897882474999));
#211210=CARTESIAN_POINT('Ctrl Pts',(-37.4688711863709,-76.7516201686318,
60.673084533));
#211211=CARTESIAN_POINT('Ctrl Pts',(-37.5665385726609,-80.7396717903781,
61.9524320656214));
#211212=CARTESIAN_POINT('Ctrl Pts',(-37.6642059589509,-84.0771060637059,
64.482811111911));
#211213=CARTESIAN_POINT('Ctrl Pts',(-37.7618733452409,-86.3856101026459,
67.9773919605015));
#211214=CARTESIAN_POINT('Ctrl Pts',(-37.8595407315309,-87.4035042235849,
72.0400483107849));
#211215=CARTESIAN_POINT('Ctrl Pts',(-37.9572081178209,-87.0154074123175,
76.2102600797002));
#211216=CARTESIAN_POINT('Ctrl Pts',(-38.0548755041109,-85.265305410114,
80.0153149192114));
#211217=CARTESIAN_POINT('Ctrl Pts',(-38.1525428904009,-82.351605282947,
83.0238940611852));
#211218=CARTESIAN_POINT('Ctrl Pts',(-38.2502102766909,-78.60449376888,84.8949575070187));
#211219=CARTESIAN_POINT('Ctrl Pts',(-38.3153218675509,-75.8342138642759,
85.2426041509182));
#211220=CARTESIAN_POINT('Ctrl Pts',(-38.3478776629809,-74.4593099020373,
85.1816337132426));
#211221=CARTESIAN_POINT('Ctrl Pts',(-32.3212930507009,-79.4192347374965,
62.0755168906179));
#211222=CARTESIAN_POINT('Ctrl Pts',(-32.3538488461309,-80.6498714739172,
62.5738479625973));
#211223=CARTESIAN_POINT('Ctrl Pts',(-32.4189604369909,-82.9406351405637,
63.9906830308551));
#211224=CARTESIAN_POINT('Ctrl Pts',(-32.5166278232809,-85.4769223199675,
67.1360227552467));
#211225=CARTESIAN_POINT('Ctrl Pts',(-32.6142952095709,-86.8255373180291,
70.944784032297));
#211226=CARTESIAN_POINT('Ctrl Pts',(-32.7119625958609,-86.8336928790153,
74.9852609507784));
#211227=CARTESIAN_POINT('Ctrl Pts',(-32.8096299821509,-85.5004419587156,
78.7994383430527));
#211228=CARTESIAN_POINT('Ctrl Pts',(-32.9072973684309,-82.9769205267125,
81.9549646900448));
#211229=CARTESIAN_POINT('Ctrl Pts',(-33.0049647547209,-79.5491793382486,
84.0941463918273));
#211230=CARTESIAN_POINT('Ctrl Pts',(-33.1026321410109,-75.6057685340114,
84.9744978657157));
#211231=CARTESIAN_POINT('Ctrl Pts',(-33.2002995273009,-71.5936911480816,
84.4962273102156));
#211232=CARTESIAN_POINT('Ctrl Pts',(-33.2979669135909,-67.9677340244805,
82.7135488322342));
#211233=CARTESIAN_POINT('Ctrl Pts',(-33.3956342998809,-65.1389155189428,
79.8285369611779));
#211234=CARTESIAN_POINT('Ctrl Pts',(-33.4933016861709,-63.4278947906478,
76.1682206227875));
#211235=CARTESIAN_POINT('Ctrl Pts',(-33.5909690724609,-63.0286236472347,
72.1475129506798));
#211236=CARTESIAN_POINT('Ctrl Pts',(-33.6886364587509,-63.9863612484711,
68.2221790390764));
#211237=CARTESIAN_POINT('Ctrl Pts',(-33.7863038450409,-66.1925437782824,
64.8371729422473));
#211238=CARTESIAN_POINT('Ctrl Pts',(-33.8839712313309,-69.397090636349,
62.3762001539254));
#211239=CARTESIAN_POINT('Ctrl Pts',(-33.9816386176209,-73.2367521861339,
61.1182228832598));
#211240=CARTESIAN_POINT('Ctrl Pts',(-34.0793060039109,-77.2762857165359,
61.2058384479296));
#211241=CARTESIAN_POINT('Ctrl Pts',(-34.1769733902009,-81.0577921386458,
62.6291152340621));
#211242=CARTESIAN_POINT('Ctrl Pts',(-34.2746407764909,-84.1526208836926,
65.2267184888439));
#211243=CARTESIAN_POINT('Ctrl Pts',(-34.3723081627809,-86.2099593511533,
68.7041983321678));
#211244=CARTESIAN_POINT('Ctrl Pts',(-34.4699755490709,-86.9965990770434,
72.6673669599299));
#211245=CARTESIAN_POINT('Ctrl Pts',(-34.5676429353609,-86.4233709503677,
76.6669815845159));
#211246=CARTESIAN_POINT('Ctrl Pts',(-34.6653103216509,-84.5552529283401,
80.2496681025061));
#211247=CARTESIAN_POINT('Ctrl Pts',(-34.7629777079409,-81.6040044960209,
83.0093130653876));
#211248=CARTESIAN_POINT('Ctrl Pts',(-34.8606450942309,-77.9041627869953,
84.6330984448553));
#211249=CARTESIAN_POINT('Ctrl Pts',(-34.9583124805209,-73.8751213116633,
84.9369609474145));
#211250=CARTESIAN_POINT('Ctrl Pts',(-35.0559798668109,-69.9735898378284,
83.8864564071507));
#211251=CARTESIAN_POINT('Ctrl Pts',(-35.1536472531009,-66.6418243076185,
81.6006641851604));
#211252=CARTESIAN_POINT('Ctrl Pts',(-35.2513146393909,-64.2574951597656,
78.338688994402));
#211253=CARTESIAN_POINT('Ctrl Pts',(-35.3489820256809,-63.090876705969,
74.4702902282876));
#211254=CARTESIAN_POINT('Ctrl Pts',(-35.4466494119709,-63.2742103357459,
70.433968089186));
#211255=CARTESIAN_POINT('Ctrl Pts',(-35.5443167982609,-64.7867143669015,
66.6872576405196));
#211256=CARTESIAN_POINT('Ctrl Pts',(-35.6419841845509,-67.4569397416147,
63.6548651727437));
#211257=CARTESIAN_POINT('Ctrl Pts',(-35.7396515708509,-70.9822045395409,
61.6805258566954));
#211258=CARTESIAN_POINT('Ctrl Pts',(-35.8373189571409,-74.9629043194786,
60.9880398334549));
#211259=CARTESIAN_POINT('Ctrl Pts',(-35.9349863434309,-78.9478090597658,
61.6559034731573));
#211260=CARTESIAN_POINT('Ctrl Pts',(-36.0326537297209,-82.485212087779,
63.6084114623351));
#211261=CARTESIAN_POINT('Ctrl Pts',(-36.1303211160109,-85.1741330399482,
66.6242383378935));
#211262=CARTESIAN_POINT('Ctrl Pts',(-36.2279885023009,-86.7097707691124,
70.3615267125221));
#211263=CARTESIAN_POINT('Ctrl Pts',(-36.3256558885909,-86.9180539098912,
74.3966383297691));
#211264=CARTESIAN_POINT('Ctrl Pts',(-36.4233232748809,-85.7753726420844,
78.2721753442413));
#211265=CARTESIAN_POINT('Ctrl Pts',(-36.5209906611709,-83.4112549687333,
81.5488284013896));
#211266=CARTESIAN_POINT('Ctrl Pts',(-36.6186580474609,-80.0936841410099,
83.8551743063604));
#211267=CARTESIAN_POINT('Ctrl Pts',(-36.7163254337509,-76.1987215650125,
84.9297784948444));
#211268=CARTESIAN_POINT('Ctrl Pts',(-36.8139928200409,-72.1678785690723,
84.6508298034518));
#211269=CARTESIAN_POINT('Ctrl Pts',(-36.9116602063309,-68.4580691313762,
83.0499483068092));
#211270=CARTESIAN_POINT('Ctrl Pts',(-37.0093275926209,-65.489816648677,
80.3086010414542));
#211271=CARTESIAN_POINT('Ctrl Pts',(-37.1069949789109,-63.5995857392998,
76.7375319102927));
#211272=CARTESIAN_POINT('Ctrl Pts',(-37.2046623652009,-63.0016424824015,
72.7415374793882));
#211273=CARTESIAN_POINT('Ctrl Pts',(-37.3023297514909,-63.7637664051097,
68.7735814871057));
#211274=CARTESIAN_POINT('Ctrl Pts',(-37.3999971377809,-65.7995673717778,
65.2834493901101));
#211275=CARTESIAN_POINT('Ctrl Pts',(-37.4976645240709,-68.8782782897348,
62.6667631817017));
#211276=CARTESIAN_POINT('Ctrl Pts',(-37.5953319103609,-72.6509135864917,
61.2201358796829));
#211277=CARTESIAN_POINT('Ctrl Pts',(-37.6929992966509,-76.6898282723673,
61.1075491215586));
#211278=CARTESIAN_POINT('Ctrl Pts',(-37.7906666829409,-80.5371934162449,
62.3417651174235));
#211279=CARTESIAN_POINT('Ctrl Pts',(-37.8883340692309,-83.7568930367679,
64.7828799942741));
#211280=CARTESIAN_POINT('Ctrl Pts',(-37.9860014555209,-85.9839599898376,
68.1541825310842));
#211281=CARTESIAN_POINT('Ctrl Pts',(-38.0836688418109,-86.9659458647775,
72.0735205728459));
#211282=CARTESIAN_POINT('Ctrl Pts',(-38.1813362281009,-86.5915399428526,
76.0966198012583));
#211283=CARTESIAN_POINT('Ctrl Pts',(-38.2790036143909,-84.9031762805598,
79.7674437395071));
#211284=CARTESIAN_POINT('Ctrl Pts',(-38.3766710006809,-82.092262738757,
82.669889249567));
#211285=CARTESIAN_POINT('Ctrl Pts',(-38.4743383869709,-78.4773380595411,
84.4749471992291));
#211286=CARTESIAN_POINT('Ctrl Pts',(-38.5394499778309,-75.804785305799,
84.8103299141412));
#211287=CARTESIAN_POINT('Ctrl Pts',(-38.5720057732609,-74.4783838240209,
84.7515103303026));
#211288=CARTESIAN_POINT('',(-37.8135594354587,-79.7260345616507,85.0994033094111));
#211289=CARTESIAN_POINT('Ctrl Pts',(-37.8135412566022,-79.7265008243874,
85.0992154535007));
#211290=CARTESIAN_POINT('Ctrl Pts',(-37.9141945917161,-79.656190438583,
84.9191034084108));
#211291=CARTESIAN_POINT('Ctrl Pts',(-38.0148480643992,-79.5858805128641,
84.7389909011183));
#211292=CARTESIAN_POINT('Ctrl Pts',(-38.2164814622351,-79.4450337333417,
84.3781812915445));
#211293=CARTESIAN_POINT('Ctrl Pts',(-38.3174616202436,-79.3744967204846,
84.1974837711852));
#211294=CARTESIAN_POINT('Ctrl Pts',(-38.4184416307607,-79.3039603665244,
84.0167862995282));
#211295=CARTESIAN_POINT('',(-31.8032830015106,-84.3356921461145,63.942145982536));
#211296=CARTESIAN_POINT('Ctrl Pts',(-36.4473639743914,-62.9850802944281,
77.9529305295057));
#211297=CARTESIAN_POINT('Ctrl Pts',(-36.4543241802223,-62.8662959481017,
77.665425985869));
#211298=CARTESIAN_POINT('Ctrl Pts',(-36.4612900402069,-62.7578055866838,
77.3735961326477));
#211299=CARTESIAN_POINT('Ctrl Pts',(-36.485117930428,-62.4205173636423,
76.355723017862));
#211300=CARTESIAN_POINT('Ctrl Pts',(-36.5017296931877,-62.2450550777804,
75.6138349173405));
#211301=CARTESIAN_POINT('Ctrl Pts',(-36.5357274612721,-62.0247013039446,
74.0995341640204));
#211302=CARTESIAN_POINT('Ctrl Pts',(-36.5530476473795,-61.981718828881,
73.329864494191));
#211303=CARTESIAN_POINT('Ctrl Pts',(-36.5916197209741,-62.0390359146387,
71.5897218188896));
#211304=CARTESIAN_POINT('Ctrl Pts',(-36.6128801976632,-62.1798186416409,
70.6251596328269));
#211305=CARTESIAN_POINT('Ctrl Pts',(-36.6439294954884,-62.5328099313688,
69.281688088584));
#211306=CARTESIAN_POINT('Ctrl Pts',(-36.6532881833061,-62.6582388994359,
68.8833927198607));
#211307=CARTESIAN_POINT('Ctrl Pts',(-36.6809267326242,-63.0881923767221,
67.7172302332754));
#211308=CARTESIAN_POINT('Ctrl Pts',(-36.6989314919195,-63.4469139763311,
66.9716008860826));
#211309=CARTESIAN_POINT('Ctrl Pts',(-36.7364395657127,-64.3189605283735,
65.5286083221384));
#211310=CARTESIAN_POINT('Ctrl Pts',(-36.7557782652972,-64.8360286904484,
64.8381780403023));
#211311=CARTESIAN_POINT('Ctrl Pts',(-36.7839612892329,-65.6992197482852,
63.8966248022828));
#211312=CARTESIAN_POINT('Ctrl Pts',(-36.7931293056665,-65.9955511341076,
63.6030655527872));
#211313=CARTESIAN_POINT('Ctrl Pts',(-36.8208453918513,-66.9263589877273,
62.7656896735039));
#211314=CARTESIAN_POINT('Ctrl Pts',(-36.8396120669197,-67.5996227911344,
62.2682600303921));
#211315=CARTESIAN_POINT('Ctrl Pts',(-36.8761230715828,-69.0081416355683,
61.4238997206659));
#211316=CARTESIAN_POINT('Ctrl Pts',(-36.8937294894461,-69.7374966540635,
61.074300943056));
#211317=CARTESIAN_POINT('Ctrl Pts',(-36.9308123211814,-71.3016845990245,
60.4963768345923));
#211318=CARTESIAN_POINT('Ctrl Pts',(-36.9501609036144,-72.1364439111921,
60.2790324585819));
#211319=CARTESIAN_POINT('Ctrl Pts',(-36.978330496994,-73.3974509651564,
60.0813397198586));
#211320=CARTESIAN_POINT('Ctrl Pts',(-36.9874757398909,-73.8112215024371,
60.0366769320551));
#211321=CARTESIAN_POINT('Ctrl Pts',(-37.0151974403007,-75.0617540677333,
59.9621303772785));
#211322=CARTESIAN_POINT('Ctrl Pts',(-37.033990966252,-75.8999419217079,
59.993107255278));
#211323=CARTESIAN_POINT('Ctrl Pts',(-37.0719276034909,-77.5900391620661,
60.2199469355597));
#211324=CARTESIAN_POINT('Ctrl Pts',(-37.0908557950954,-78.4370257822214,
60.4214292563707));
#211325=CARTESIAN_POINT('Ctrl Pts',(-37.1293461869287,-80.0703946238553,
60.9875916109183));
#211326=CARTESIAN_POINT('Ctrl Pts',(-37.1486534495965,-80.8532460091769,
61.3493201333601));
#211327=CARTESIAN_POINT('Ctrl Pts',(-37.176861062698,-81.9555297796532,
61.9981658508267));
#211328=CARTESIAN_POINT('Ctrl Pts',(-37.1860769038382,-82.305971777073,
62.2279333725017));
#211329=CARTESIAN_POINT('Ctrl Pts',(-37.2143986726791,-83.3398725112968,
62.9796324327799));
#211330=CARTESIAN_POINT('Ctrl Pts',(-37.2337467737194,-83.9831984350049,
63.5527441000205));
#211331=CARTESIAN_POINT('Ctrl Pts',(-37.2730206552509,-85.1829821911235,
64.8563039758477));
#211332=CARTESIAN_POINT('Ctrl Pts',(-37.2929574213215,-85.7283677887833,
65.5906324615143));
#211333=CARTESIAN_POINT('Ctrl Pts',(-37.3226165148976,-86.4041788015047,
66.7344460687353));
#211334=CARTESIAN_POINT('Ctrl Pts',(-37.331952372424,-86.5986311571669,
67.1028796803519));
#211335=CARTESIAN_POINT('Ctrl Pts',(-37.3691472807876,-87.3053212567826,
68.6134082064923));
#211336=CARTESIAN_POINT('Ctrl Pts',(-37.3963711391022,-87.6691654605218,
69.8174527414559));
#211337=CARTESIAN_POINT('Ctrl Pts',(-37.4337911968826,-87.9179781646002,
71.4712655513977));
#211338=CARTESIAN_POINT('Ctrl Pts',(-37.4432018905373,-87.9603582315639,
71.8904995638018));
#211339=CARTESIAN_POINT('Ctrl Pts',(-37.4666736267226,-88.0157060709946,
72.9505504624398));
#211340=CARTESIAN_POINT('Ctrl Pts',(-37.4807126142551,-88.0017984756817,
73.591643275133));
#211341=CARTESIAN_POINT('Ctrl Pts',(-37.5120280994412,-87.8673101327979,
74.9949391007185));
#211342=CARTESIAN_POINT('Ctrl Pts',(-37.5293477014922,-87.7260732777811,
75.7527569995565));
#211343=CARTESIAN_POINT('Ctrl Pts',(-37.5673950034065,-87.2631759441533,
77.4061926447705));
#211344=CARTESIAN_POINT('Ctrl Pts',(-37.5881189354855,-86.9086724029588,
78.2880952478141));
#211345=CARTESIAN_POINT('Ctrl Pts',(-37.6177617346494,-86.2825812137115,
79.457820072434));
#211346=CARTESIAN_POINT('Ctrl Pts',(-37.6262594874007,-86.0891590173064,
79.7840534963821));
#211347=CARTESIAN_POINT('Ctrl Pts',(-37.6615797474437,-85.2225597219804,
81.1099098905177));
#211348=CARTESIAN_POINT('Ctrl Pts',(-37.6877898088874,-84.4263406844536,
82.0219288772879));
#211349=CARTESIAN_POINT('Ctrl Pts',(-37.7230062828639,-83.2369419520325,
83.0531423108285));
#211350=CARTESIAN_POINT('Ctrl Pts',(-37.7312775772375,-82.9477112373158,
83.2830764354318));
#211351=CARTESIAN_POINT('Ctrl Pts',(-37.7642212958841,-81.7474044354274,
84.1565247586272));
#211352=CARTESIAN_POINT('Ctrl Pts',(-37.7885929278986,-80.7650329325693,
84.6939292153208));
#211353=CARTESIAN_POINT('Ctrl Pts',(-37.8135449901798,-79.7261875999371,
85.0993456443021));
#211354=CARTESIAN_POINT('Ctrl Pts',(-37.7678684231509,-80.2245721714987,
84.9428528583424));
#211355=CARTESIAN_POINT('Ctrl Pts',(-37.8179054464809,-78.1874891607719,
85.9277583999695));
#211356=CARTESIAN_POINT('Ctrl Pts',(-37.9179794931409,-73.5482212730369,
86.8316803850282));
#211357=CARTESIAN_POINT('Ctrl Pts',(-38.0680905631309,-66.7022463072535,
84.5014189876433));
#211358=CARTESIAN_POINT('Ctrl Pts',(-38.2182016331209,-61.8311972113564,
78.9684584806007));
#211359=CARTESIAN_POINT('Ctrl Pts',(-38.3182756797809,-60.8302931416496,
74.0638248418014));
#211360=CARTESIAN_POINT('Ctrl Pts',(-38.3683127031109,-60.9803062607213,
71.6256255348517));
#211361=CARTESIAN_POINT('Ctrl Pts',(-37.9919965334309,-80.0521476485986,
84.5483408522442));
#211362=CARTESIAN_POINT('Ctrl Pts',(-38.0420335567609,-78.0834391555961,
85.5033627821869));
#211363=CARTESIAN_POINT('Ctrl Pts',(-38.1421076034109,-73.5967117403114,
86.3839207906894));
#211364=CARTESIAN_POINT('Ctrl Pts',(-38.2922186734109,-66.9668082009882,
84.1369185523978));
#211365=CARTESIAN_POINT('Ctrl Pts',(-38.4423297434009,-62.2418829099991,
78.7835876157209));
#211366=CARTESIAN_POINT('Ctrl Pts',(-38.5424037900609,-61.2660399523217,
74.0312248270541));
#211367=CARTESIAN_POINT('Ctrl Pts',(-38.5924408133809,-61.4088311706314,
71.6672949557471));
#211368=CARTESIAN_POINT('Ctrl Pts',(-38.2161246437009,-79.8797231256986,
84.1538288461459));
#211369=CARTESIAN_POINT('Ctrl Pts',(-38.2661616670309,-77.9793891504164,
85.078967164395));
#211370=CARTESIAN_POINT('Ctrl Pts',(-38.3662357136909,-73.645202207582,
85.9361611963413));
#211371=CARTESIAN_POINT('Ctrl Pts',(-38.5163467836809,-67.2313700947256,
83.7724181171587));
#211372=CARTESIAN_POINT('Ctrl Pts',(-38.6664578536809,-62.652568608624,
78.5987167508506));
#211373=CARTESIAN_POINT('Ctrl Pts',(-38.7665319003309,-61.7017867629931,
73.998624812305));
#211374=CARTESIAN_POINT('Ctrl Pts',(-38.8165689236609,-61.8373560805414,
71.7089643766425));
#211375=CARTESIAN_POINT('Ctrl Pts',(-38.4402527539809,-79.7072986027986,
83.7593168400476));
#211376=CARTESIAN_POINT('Ctrl Pts',(-38.4902897773109,-77.8753391452405,
84.6545715466123));
#211377=CARTESIAN_POINT('Ctrl Pts',(-38.5903638239709,-73.6936926748527,
85.4884016019933));
#211378=CARTESIAN_POINT('Ctrl Pts',(-38.7404748939609,-67.49593198846,83.4079176819122));
#211379=CARTESIAN_POINT('Ctrl Pts',(-38.8905859639509,-63.0632543072575,
78.4138458859746));
#211380=CARTESIAN_POINT('Ctrl Pts',(-38.9906600106109,-62.1375335736656,
73.9660247975586));
#211381=CARTESIAN_POINT('Ctrl Pts',(-39.0406970339409,-62.2658809904518,
71.7506337975388));
#211382=CARTESIAN_POINT('Ctrl Pts',(-38.9114901698969,-62.0210675377945,
72.2490839199139));
#211383=CARTESIAN_POINT('Ctrl Pts',(-38.9253796493603,-62.0477053299784,
72.2506022870319));
#211384=CARTESIAN_POINT('Ctrl Pts',(-38.9392691288105,-62.0743431221692,
72.2521206541503));
#211385=CARTESIAN_POINT('Ctrl Pts',(-38.9670676750248,-62.1276562719404,
72.2551595296326));
#211386=CARTESIAN_POINT('Ctrl Pts',(-38.9809767417889,-62.1543316295209,
72.2566800379965));
#211387=CARTESIAN_POINT('Ctrl Pts',(-38.9948858085393,-62.1810069871086,
72.2582005463609));
#211388=CARTESIAN_POINT('Ctrl Pts',(-38.6651607695592,-62.9850797267618,
77.9529291555313));
#211389=CARTESIAN_POINT('Ctrl Pts',(-38.61247162501,-63.4651597069569,79.1149107179876));
#211390=CARTESIAN_POINT('Ctrl Pts',(-38.5579303068348,-64.1112609851083,
80.2010992341744));
#211391=CARTESIAN_POINT('Ctrl Pts',(-38.4509479952484,-65.7059259388704,
82.1673583393617));
#211392=CARTESIAN_POINT('Ctrl Pts',(-38.3992043907891,-66.6498484985761,
83.0337413163219));
#211393=CARTESIAN_POINT('Ctrl Pts',(-38.3094997884852,-68.3950020381939,
84.2169638927091));
#211394=CARTESIAN_POINT('Ctrl Pts',(-38.2735339351584,-69.1287945259406,
84.6175018705529));
#211395=CARTESIAN_POINT('Ctrl Pts',(-38.166422504845,-71.447408923872,85.6073284218056));
#211396=CARTESIAN_POINT('Ctrl Pts',(-38.0982006061265,-73.1130898711673,
85.9613759922044));
#211397=CARTESIAN_POINT('Ctrl Pts',(-37.9903150495058,-75.6328782495681,
86.0001753956267));
#211398=CARTESIAN_POINT('Ctrl Pts',(-37.9546993734579,-76.4652312027286,
85.9328938291295));
#211399=CARTESIAN_POINT('Ctrl Pts',(-37.8839532152002,-78.1193429154257,
85.6374986271243));
#211400=CARTESIAN_POINT('Ctrl Pts',(-37.8490190852945,-78.9367127274665,
85.4074198623626));
#211401=CARTESIAN_POINT('Ctrl Pts',(-37.8135657720877,-79.7258720358075,
85.0994687906041));
#211402=CARTESIAN_POINT('Origin',(-39.1448867524609,-61.0226881170831,72.1921758070624));
#211403=CARTESIAN_POINT('Ctrl Pts',(-39.2948856686008,-62.1810067175759,
72.2582005309974));
#211404=CARTESIAN_POINT('Ctrl Pts',(-39.3087857943346,-62.1543485130583,
72.2566810003664));
#211405=CARTESIAN_POINT('Ctrl Pts',(-39.3226859200676,-62.1276903085403,
72.2551614697354));
#211406=CARTESIAN_POINT('Ctrl Pts',(-39.3504844252439,-62.0743772486039,
72.2521225993737));
#211407=CARTESIAN_POINT('Ctrl Pts',(-39.3643828046871,-62.0477223931856,
72.250603259643));
#211408=CARTESIAN_POINT('Ctrl Pts',(-39.3782811841296,-62.0210675377669,
72.2490839199123));
#211409=CARTESIAN_POINT('Ctrl Pts',(-38.6717262017909,-79.7072986027985,
83.7593168400477));
#211410=CARTESIAN_POINT('Ctrl Pts',(-38.7217632251209,-77.8753391452405,
84.6545715466123));
#211411=CARTESIAN_POINT('Ctrl Pts',(-38.8218372717809,-73.6936926748527,
85.4884016019933));
#211412=CARTESIAN_POINT('Ctrl Pts',(-38.9719483417709,-67.49593198846,83.4079176819122));
#211413=CARTESIAN_POINT('Ctrl Pts',(-39.1220594117609,-63.0632543072574,
78.4138458859745));
#211414=CARTESIAN_POINT('Ctrl Pts',(-39.2221334584209,-62.1375335736652,
73.9660247975577));
#211415=CARTESIAN_POINT('Ctrl Pts',(-39.2721704817509,-62.2658809904518,
71.7506337975388));
#211416=CARTESIAN_POINT('Ctrl Pts',(-38.8958543120709,-79.8797231256985,
84.153828846146));
#211417=CARTESIAN_POINT('Ctrl Pts',(-38.9458913354009,-77.9793891504164,
85.078967164395));
#211418=CARTESIAN_POINT('Ctrl Pts',(-39.0459653820509,-73.645202207582,
85.9361611963413));
#211419=CARTESIAN_POINT('Ctrl Pts',(-39.1960764520509,-67.2313700947253,
83.7724181171577));
#211420=CARTESIAN_POINT('Ctrl Pts',(-39.3461875220409,-62.652568608624,
78.5987167508506));
#211421=CARTESIAN_POINT('Ctrl Pts',(-39.4462615687009,-61.7017867629931,
73.998624812305));
#211422=CARTESIAN_POINT('Ctrl Pts',(-39.4962985920209,-61.8373560805414,
71.7089643766425));
#211423=CARTESIAN_POINT('Ctrl Pts',(-39.1199824223409,-80.0521476485985,
84.5483408522443));
#211424=CARTESIAN_POINT('Ctrl Pts',(-39.1700194456709,-78.0834391555961,
85.5033627821869));
#211425=CARTESIAN_POINT('Ctrl Pts',(-39.2700934923309,-73.5967117403114,
86.3839207906894));
#211426=CARTESIAN_POINT('Ctrl Pts',(-39.4202045623209,-66.9668082009882,
84.1369185523978));
#211427=CARTESIAN_POINT('Ctrl Pts',(-39.5703156323209,-62.241882909999,
78.7835876157208));
#211428=CARTESIAN_POINT('Ctrl Pts',(-39.6703896789709,-61.2660399523217,
74.0312248270541));
#211429=CARTESIAN_POINT('Ctrl Pts',(-39.7204267023009,-61.4088311706314,
71.6672949557471));
#211430=CARTESIAN_POINT('Ctrl Pts',(-39.3441105326209,-80.2245721714985,
84.9428528583425));
#211431=CARTESIAN_POINT('Ctrl Pts',(-39.3941475559509,-78.1874891607719,
85.9277583999695));
#211432=CARTESIAN_POINT('Ctrl Pts',(-39.4942216026109,-73.5482212730369,
86.8316803850282));
#211433=CARTESIAN_POINT('Ctrl Pts',(-39.6443326726009,-66.7022463072535,
84.5014189876433));
#211434=CARTESIAN_POINT('Ctrl Pts',(-39.7944437425909,-61.8311972113564,
78.9684584806006));
#211435=CARTESIAN_POINT('Ctrl Pts',(-39.8945177892509,-60.8302931416493,
74.0638248418005));
#211436=CARTESIAN_POINT('Ctrl Pts',(-39.9445548125809,-60.9803062607213,
71.6256255348517));
#211437=CARTESIAN_POINT('Ctrl Pts',(-38.7166027955228,-79.3038821947565,
84.0168244534335));
#211438=CARTESIAN_POINT('Ctrl Pts',(-38.8175042526392,-79.3743616523911,
84.1973833874513));
#211439=CARTESIAN_POINT('Ctrl Pts',(-38.918405870868,-79.4448417742437,
84.3779423951187));
#211440=CARTESIAN_POINT('Ctrl Pts',(-39.1200383310617,-79.5856838366802,
84.7387543832486));
#211441=CARTESIAN_POINT('Ctrl Pts',(-39.220769502857,-79.6560460057835,
84.9190079546549));
#211442=CARTESIAN_POINT('Ctrl Pts',(-39.3215005357773,-79.7264086317985,
85.0992610619778));
#211443=CARTESIAN_POINT('Ctrl Pts',(-32.5527664985109,-79.4192347374965,
62.0755168906179));
#211444=CARTESIAN_POINT('Ctrl Pts',(-32.5853222939409,-80.6498714739172,
62.5738479625973));
#211445=CARTESIAN_POINT('Ctrl Pts',(-32.6504338848009,-82.9406351405637,
63.9906830308551));
#211446=CARTESIAN_POINT('Ctrl Pts',(-32.7481012710909,-85.4769223199675,
67.1360227552467));
#211447=CARTESIAN_POINT('Ctrl Pts',(-32.8457686573809,-86.8255373180291,
70.944784032297));
#211448=CARTESIAN_POINT('Ctrl Pts',(-32.9434360436709,-86.8336928790153,
74.9852609507784));
#211449=CARTESIAN_POINT('Ctrl Pts',(-33.0411034299609,-85.5004419587156,
78.7994383430527));
#211450=CARTESIAN_POINT('Ctrl Pts',(-33.1387708162509,-82.9769205267125,
81.9549646900448));
#211451=CARTESIAN_POINT('Ctrl Pts',(-33.2364382025409,-79.5491793382486,
84.0941463918273));
#211452=CARTESIAN_POINT('Ctrl Pts',(-33.3341055888209,-75.6057685340114,
84.9744978657157));
#211453=CARTESIAN_POINT('Ctrl Pts',(-33.4317729751109,-71.5936911480816,
84.4962273102156));
#211454=CARTESIAN_POINT('Ctrl Pts',(-33.5294403614009,-67.9677340244805,
82.7135488322342));
#211455=CARTESIAN_POINT('Ctrl Pts',(-33.6271077476909,-65.1389155189428,
79.8285369611779));
#211456=CARTESIAN_POINT('Ctrl Pts',(-33.7247751339809,-63.4278947906478,
76.1682206227875));
#211457=CARTESIAN_POINT('Ctrl Pts',(-33.8224425202709,-63.0286236472347,
72.1475129506798));
#211458=CARTESIAN_POINT('Ctrl Pts',(-33.9201099065609,-63.9863612484711,
68.2221790390764));
#211459=CARTESIAN_POINT('Ctrl Pts',(-34.0177772928509,-66.1925437782824,
64.8371729422473));
#211460=CARTESIAN_POINT('Ctrl Pts',(-34.1154446791409,-69.397090636349,
62.3762001539254));
#211461=CARTESIAN_POINT('Ctrl Pts',(-34.2131120654309,-73.2367521861339,
61.1182228832598));
#211462=CARTESIAN_POINT('Ctrl Pts',(-34.3107794517209,-77.2762857165359,
61.2058384479296));
#211463=CARTESIAN_POINT('Ctrl Pts',(-34.4084468380109,-81.0577921386454,
62.6291152340612));
#211464=CARTESIAN_POINT('Ctrl Pts',(-34.5061142243009,-84.1526208836926,
65.2267184888439));
#211465=CARTESIAN_POINT('Ctrl Pts',(-34.6037816105909,-86.2099593511533,
68.7041983321678));
#211466=CARTESIAN_POINT('Ctrl Pts',(-34.7014489968809,-86.9965990770434,
72.6673669599299));
#211467=CARTESIAN_POINT('Ctrl Pts',(-34.7991163831709,-86.4233709503677,
76.6669815845159));
#211468=CARTESIAN_POINT('Ctrl Pts',(-34.8967837694509,-84.5552529283401,
80.2496681025061));
#211469=CARTESIAN_POINT('Ctrl Pts',(-34.9944511557409,-81.6040044960209,
83.0093130653876));
#211470=CARTESIAN_POINT('Ctrl Pts',(-35.0921185420309,-77.9041627869953,
84.6330984448553));
#211471=CARTESIAN_POINT('Ctrl Pts',(-35.1897859283209,-73.8751213116633,
84.9369609474145));
#211472=CARTESIAN_POINT('Ctrl Pts',(-35.2874533146109,-69.9735898378284,
83.8864564071507));
#211473=CARTESIAN_POINT('Ctrl Pts',(-35.3851207009009,-66.6418243076185,
81.6006641851604));
#211474=CARTESIAN_POINT('Ctrl Pts',(-35.4827880871909,-64.2574951597656,
78.3386889944021));
#211475=CARTESIAN_POINT('Ctrl Pts',(-35.5804554734809,-63.090876705969,
74.4702902282876));
#211476=CARTESIAN_POINT('Ctrl Pts',(-35.6781228597709,-63.2742103357459,
70.433968089186));
#211477=CARTESIAN_POINT('Ctrl Pts',(-35.7757902460609,-64.7867143669015,
66.6872576405196));
#211478=CARTESIAN_POINT('Ctrl Pts',(-35.8734576323509,-67.4569397416147,
63.6548651727437));
#211479=CARTESIAN_POINT('Ctrl Pts',(-35.9711250186409,-70.982204539541,
61.6805258566954));
#211480=CARTESIAN_POINT('Ctrl Pts',(-36.0687924049309,-74.9629043194786,
60.9880398334549));
#211481=CARTESIAN_POINT('Ctrl Pts',(-36.1664597912209,-78.9478090597658,
61.6559034731573));
#211482=CARTESIAN_POINT('Ctrl Pts',(-36.2641271775109,-82.485212087779,
63.6084114623351));
#211483=CARTESIAN_POINT('Ctrl Pts',(-36.3617945638009,-85.1741330399482,
66.6242383378935));
#211484=CARTESIAN_POINT('Ctrl Pts',(-36.4594619500909,-86.7097707691124,
70.3615267125221));
#211485=CARTESIAN_POINT('Ctrl Pts',(-36.5571293363809,-86.9180539098912,
74.3966383297691));
#211486=CARTESIAN_POINT('Ctrl Pts',(-36.6547967226709,-85.7753726420844,
78.2721753442413));
#211487=CARTESIAN_POINT('Ctrl Pts',(-36.7524641089609,-83.4112549687333,
81.5488284013896));
#211488=CARTESIAN_POINT('Ctrl Pts',(-36.8501314952509,-80.0936841410099,
83.8551743063604));
#211489=CARTESIAN_POINT('Ctrl Pts',(-36.9477988815409,-76.1987215650125,
84.9297784948444));
#211490=CARTESIAN_POINT('Ctrl Pts',(-37.0454662678409,-72.1678785690723,
84.6508298034518));
#211491=CARTESIAN_POINT('Ctrl Pts',(-37.1431336541309,-68.4580691313762,
83.0499483068092));
#211492=CARTESIAN_POINT('Ctrl Pts',(-37.2408010404209,-65.489816648677,
80.3086010414542));
#211493=CARTESIAN_POINT('Ctrl Pts',(-37.3384684267109,-63.5995857392998,
76.7375319102927));
#211494=CARTESIAN_POINT('Ctrl Pts',(-37.4361358130009,-63.0016424824015,
72.7415374793882));
#211495=CARTESIAN_POINT('Ctrl Pts',(-37.5338031992909,-63.7637664051097,
68.7735814871057));
#211496=CARTESIAN_POINT('Ctrl Pts',(-37.6314705855809,-65.7995673717778,
65.2834493901101));
#211497=CARTESIAN_POINT('Ctrl Pts',(-37.7291379718709,-68.8782782897348,
62.6667631817017));
#211498=CARTESIAN_POINT('Ctrl Pts',(-37.8268053581609,-72.6509135864917,
61.2201358796829));
#211499=CARTESIAN_POINT('Ctrl Pts',(-37.9244727444509,-76.6898282723673,
61.1075491215586));
#211500=CARTESIAN_POINT('Ctrl Pts',(-38.0221401307409,-80.5371934162449,
62.3417651174235));
#211501=CARTESIAN_POINT('Ctrl Pts',(-38.1198075170309,-83.7568930367679,
64.7828799942741));
#211502=CARTESIAN_POINT('Ctrl Pts',(-38.2174749033309,-85.9839599898376,
68.1541825310842));
#211503=CARTESIAN_POINT('Ctrl Pts',(-38.3151422896209,-86.9659458647775,
72.0735205728459));
#211504=CARTESIAN_POINT('Ctrl Pts',(-38.4128096759109,-86.5915399428526,
76.0966198012583));
#211505=CARTESIAN_POINT('Ctrl Pts',(-38.5104770622009,-84.9031762805598,
79.7674437395071));
#211506=CARTESIAN_POINT('Ctrl Pts',(-38.6081444484909,-82.092262738757,
82.669889249567));
#211507=CARTESIAN_POINT('Ctrl Pts',(-38.7058118347809,-78.4773380595411,
84.4749471992291));
#211508=CARTESIAN_POINT('Ctrl Pts',(-38.7709234256409,-75.804785305799,
84.8103299141412));
#211509=CARTESIAN_POINT('Ctrl Pts',(-38.8034792210709,-74.4783838240209,
84.7515103303026));
#211510=CARTESIAN_POINT('Ctrl Pts',(-32.7768946087909,-79.5808327524621,
61.6764479484404));
#211511=CARTESIAN_POINT('Ctrl Pts',(-32.8094504042209,-80.8564701429687,
62.1930014767526));
#211512=CARTESIAN_POINT('Ctrl Pts',(-32.8745619950809,-83.2310000911753,
63.6616459075254));
#211513=CARTESIAN_POINT('Ctrl Pts',(-32.9722293813709,-85.8600316025557,
66.9220011687801));
#211514=CARTESIAN_POINT('Ctrl Pts',(-33.0698967676509,-87.2579613620154,
70.8700372973401));
#211515=CARTESIAN_POINT('Ctrl Pts',(-33.1675641539409,-87.2664151471337,
75.0582622057642));
#211516=CARTESIAN_POINT('Ctrl Pts',(-33.2652315402309,-85.8844112831762,
79.0119125004583));
#211517=CARTESIAN_POINT('Ctrl Pts',(-33.3628989265209,-83.2686123238737,
82.2828268782174));
#211518=CARTESIAN_POINT('Ctrl Pts',(-33.4605663128109,-79.7155290332633,
84.5002319687039));
#211519=CARTESIAN_POINT('Ctrl Pts',(-33.5582336991009,-75.6279196525717,
85.412775226709));
#211520=CARTESIAN_POINT('Ctrl Pts',(-33.6559010853909,-71.4691327614987,
84.9170157671447));
#211521=CARTESIAN_POINT('Ctrl Pts',(-33.7535684716809,-67.7105853800127,
83.0691501424084));
#211522=CARTESIAN_POINT('Ctrl Pts',(-33.8512358579709,-64.7783255588649,
80.0786421347598));
#211523=CARTESIAN_POINT('Ctrl Pts',(-33.9489032442609,-63.0047379904651,
76.2844791261684));
#211524=CARTESIAN_POINT('Ctrl Pts',(-34.0465706305509,-62.5908667119491,
72.1167463655193));
#211525=CARTESIAN_POINT('Ctrl Pts',(-34.1442380168409,-63.5836258733412,
68.0478748946176));
#211526=CARTESIAN_POINT('Ctrl Pts',(-34.2419054031309,-65.8704818089924,
64.5390893883721));
#211527=CARTESIAN_POINT('Ctrl Pts',(-34.3395727894109,-69.1922092292778,
61.9881262869918));
#211528=CARTESIAN_POINT('Ctrl Pts',(-34.4372401757009,-73.1722755598568,
60.6841486018049));
#211529=CARTESIAN_POINT('Ctrl Pts',(-34.5349075619909,-77.3595225833569,
60.7749680020175));
#211530=CARTESIAN_POINT('Ctrl Pts',(-34.6325749482809,-81.2793072295691,
62.2502897047617));
#211531=CARTESIAN_POINT('Ctrl Pts',(-34.7302423345709,-84.4873044781106,
64.9428794344855));
#211532=CARTESIAN_POINT('Ctrl Pts',(-34.8279097208609,-86.6198735753576,
68.5475201717517));
#211533=CARTESIAN_POINT('Ctrl Pts',(-34.9255771071509,-87.4352783308858,
72.6556098596655));
#211534=CARTESIAN_POINT('Ctrl Pts',(-35.0232444934409,-86.8410889896759,
76.8014782640016));
#211535=CARTESIAN_POINT('Ctrl Pts',(-35.1209118797309,-84.9046595558289,
80.5151727650388));
#211536=CARTESIAN_POINT('Ctrl Pts',(-35.2185792660209,-81.8454929166992,
83.3757295768015));
#211537=CARTESIAN_POINT('Ctrl Pts',(-35.3162466523109,-78.0103592145147,
85.0588918641796));
#211538=CARTESIAN_POINT('Ctrl Pts',(-35.4139140386009,-73.8339879087212,
85.3738656971173));
#211539=CARTESIAN_POINT('Ctrl Pts',(-35.5115814248909,-69.7897892585688,
84.2849473910144));
#211540=CARTESIAN_POINT('Ctrl Pts',(-35.6092488111809,-66.3361911650335,
81.9155706781227));
#211541=CARTESIAN_POINT('Ctrl Pts',(-35.7069161974709,-63.8646743296805,
78.5343149451387));
#211542=CARTESIAN_POINT('Ctrl Pts',(-35.8045835837609,-62.6553961762827,
74.5244605653652));
#211543=CARTESIAN_POINT('Ctrl Pts',(-35.9022509700509,-62.8454337610229,
70.3405423640074));
#211544=CARTESIAN_POINT('Ctrl Pts',(-35.9999183563409,-64.4132454785962,
66.4568260744839));
#211545=CARTESIAN_POINT('Ctrl Pts',(-36.0975857426309,-67.181112898978,
63.3135482085524));
#211546=CARTESIAN_POINT('Ctrl Pts',(-36.1952531289209,-70.8352859417533,
61.2670132900357));
#211547=CARTESIAN_POINT('Ctrl Pts',(-36.2929205152109,-74.9615478429283,
60.5492051525981));
#211548=CARTESIAN_POINT('Ctrl Pts',(-36.3905879015009,-79.0921684670951,
61.2414905405986));
#211549=CARTESIAN_POINT('Ctrl Pts',(-36.4882552877909,-82.7589235982165,
63.2653958268243));
#211550=CARTESIAN_POINT('Ctrl Pts',(-36.5859226740809,-85.5461702366482,
66.3915023470505));
#211551=CARTESIAN_POINT('Ctrl Pts',(-36.6835900603709,-87.1379615814165,
70.2654520258604));
#211552=CARTESIAN_POINT('Ctrl Pts',(-36.7812574466609,-87.3538610051255,
74.4481154402485));
#211553=CARTESIAN_POINT('Ctrl Pts',(-36.8789248329509,-86.1693953480258,
78.4653690924801));
#211554=CARTESIAN_POINT('Ctrl Pts',(-36.9765922192409,-83.7188290595022,
81.8618394169131));
#211555=CARTESIAN_POINT('Ctrl Pts',(-37.0742596055309,-80.2799447256819,
84.2525213986484));
#211556=CARTESIAN_POINT('Ctrl Pts',(-37.1719269918209,-76.2425551780386,
85.3664206040374));
#211557=CARTESIAN_POINT('Ctrl Pts',(-37.2695943781109,-72.064316475499,
85.0772716047946));
#211558=CARTESIAN_POINT('Ctrl Pts',(-37.3672617644009,-68.2188505550257,
83.4178507257861));
#211559=CARTESIAN_POINT('Ctrl Pts',(-37.4649291506909,-65.1420580789654,
80.57626070286));
#211560=CARTESIAN_POINT('Ctrl Pts',(-37.5625965369809,-63.1827071565181,
76.8746084012712));
#211561=CARTESIAN_POINT('Ctrl Pts',(-37.6602639232709,-62.5628989277203,
72.7324925701221));
#211562=CARTESIAN_POINT('Ctrl Pts',(-37.7579313095609,-63.3528914114806,
68.6194404582811));
#211563=CARTESIAN_POINT('Ctrl Pts',(-37.8555986958509,-65.4631354468294,
65.0016848127869));
#211564=CARTESIAN_POINT('Ctrl Pts',(-37.9532660821509,-68.6544254882255,
62.2893143236977));
#211565=CARTESIAN_POINT('Ctrl Pts',(-38.0509334684409,-72.5650146189264,
60.7897882474999));
#211566=CARTESIAN_POINT('Ctrl Pts',(-38.1486008547309,-76.7516201686318,
60.673084533));
#211567=CARTESIAN_POINT('Ctrl Pts',(-38.2462682410209,-80.7396717903781,
61.9524320656214));
#211568=CARTESIAN_POINT('Ctrl Pts',(-38.3439356273109,-84.0771060637059,
64.482811111911));
#211569=CARTESIAN_POINT('Ctrl Pts',(-38.4416030136009,-86.3856101026459,
67.9773919605015));
#211570=CARTESIAN_POINT('Ctrl Pts',(-38.5392703998909,-87.4035042235849,
72.0400483107849));
#211571=CARTESIAN_POINT('Ctrl Pts',(-38.6369377861809,-87.0154074123175,
76.2102600797002));
#211572=CARTESIAN_POINT('Ctrl Pts',(-38.7346051724709,-85.2653054101149,
80.015314919211));
#211573=CARTESIAN_POINT('Ctrl Pts',(-38.8322725587709,-82.351605282947,
83.0238940611852));
#211574=CARTESIAN_POINT('Ctrl Pts',(-38.9299399450609,-78.60449376888,84.8949575070187));
#211575=CARTESIAN_POINT('Ctrl Pts',(-38.9950515359209,-75.8342138642759,
85.2426041509182));
#211576=CARTESIAN_POINT('Ctrl Pts',(-39.0276073313509,-74.4593099020373,
85.1816337132426));
#211577=CARTESIAN_POINT('Ctrl Pts',(-33.0010227190609,-79.7424307674282,
61.2773790062616));
#211578=CARTESIAN_POINT('Ctrl Pts',(-33.0335785144909,-81.0630688120212,
61.8121549909075));
#211579=CARTESIAN_POINT('Ctrl Pts',(-33.0986901053509,-83.5213650417874,
63.3326087841966));
#211580=CARTESIAN_POINT('Ctrl Pts',(-33.1963574916409,-86.2431408851346,
66.7079795823174));
#211581=CARTESIAN_POINT('Ctrl Pts',(-33.2940248779309,-87.6903854059918,
70.7952905623852));
#211582=CARTESIAN_POINT('Ctrl Pts',(-33.3916922642209,-87.6991374152512,
75.1312634607482));
#211583=CARTESIAN_POINT('Ctrl Pts',(-33.4893596505109,-86.2683806076395,
79.2243866578649));
#211584=CARTESIAN_POINT('Ctrl Pts',(-33.5870270368009,-83.5603041210376,
82.610689066389));
#211585=CARTESIAN_POINT('Ctrl Pts',(-33.6846944230909,-79.8818787282825,
84.9063175455787));
#211586=CARTESIAN_POINT('Ctrl Pts',(-33.7823618093809,-75.6500707711405,
85.8510525877097));
#211587=CARTESIAN_POINT('Ctrl Pts',(-33.8800291956709,-71.3445743749261,
85.3378042240803));
#211588=CARTESIAN_POINT('Ctrl Pts',(-33.9776965819609,-67.4534367355484,
83.4247514525908));
#211589=CARTESIAN_POINT('Ctrl Pts',(-34.0753639682509,-64.4177355988012,
80.3287473083499));
#211590=CARTESIAN_POINT('Ctrl Pts',(-34.1730313545409,-62.5815811902788,
76.400737629567));
#211591=CARTESIAN_POINT('Ctrl Pts',(-34.2706987408209,-62.1531097766604,
72.0859797803774));
#211592=CARTESIAN_POINT('Ctrl Pts',(-34.3683661271109,-63.1808904982033,
67.8735707501784));
#211593=CARTESIAN_POINT('Ctrl Pts',(-34.4660335134009,-65.5484198396858,
64.2410058345145));
#211594=CARTESIAN_POINT('Ctrl Pts',(-34.5637008996909,-68.9873278221854,
61.6000524200778));
#211595=CARTESIAN_POINT('Ctrl Pts',(-34.6613682859809,-73.1077989335492,
60.2500743203519));
#211596=CARTESIAN_POINT('Ctrl Pts',(-34.7590356722709,-77.4427594501453,
60.3440975560973));
#211597=CARTESIAN_POINT('Ctrl Pts',(-34.8567030585609,-81.5008223204608,
61.871464175445));
#211598=CARTESIAN_POINT('Ctrl Pts',(-34.9543704448509,-84.8219880725154,
64.6590403800946));
#211599=CARTESIAN_POINT('Ctrl Pts',(-35.0520378311409,-87.0297877995459,
68.390842011297));
#211600=CARTESIAN_POINT('Ctrl Pts',(-35.1497052174309,-87.8739575847217,
72.6438527593594));
#211601=CARTESIAN_POINT('Ctrl Pts',(-35.2473726037209,-87.2588070289994,
76.9359749434431));
#211602=CARTESIAN_POINT('Ctrl Pts',(-35.3450399900109,-85.2540661833469,
80.7806774275269));
#211603=CARTESIAN_POINT('Ctrl Pts',(-35.4427073763009,-82.0869813374197,
83.7421460881762));
#211604=CARTESIAN_POINT('Ctrl Pts',(-35.5403747625909,-78.1165556420916,
85.4846852834909));
#211605=CARTESIAN_POINT('Ctrl Pts',(-35.6380421488809,-73.7928545058452,
85.8107704468362));
#211606=CARTESIAN_POINT('Ctrl Pts',(-35.7357095351709,-69.6059886793678,
84.6834383749047));
#211607=CARTESIAN_POINT('Ctrl Pts',(-35.8333769214609,-66.0305580224903,
82.2304771711338));
#211608=CARTESIAN_POINT('Ctrl Pts',(-35.9310443077509,-63.4718534996216,
78.729940895939));
#211609=CARTESIAN_POINT('Ctrl Pts',(-36.0287116940409,-62.2199156466047,
74.5786309025152));
#211610=CARTESIAN_POINT('Ctrl Pts',(-36.1263790803309,-62.4166571862875,
70.2471166389011));
#211611=CARTESIAN_POINT('Ctrl Pts',(-36.2240464666209,-64.0397765902539,
66.2263945085208));
#211612=CARTESIAN_POINT('Ctrl Pts',(-36.3217138529109,-66.9052860562882,
62.9722312444263));
#211613=CARTESIAN_POINT('Ctrl Pts',(-36.4193812392009,-70.6883673438916,
60.8535007234066));
#211614=CARTESIAN_POINT('Ctrl Pts',(-36.5170486254909,-74.9601913662926,
60.1103704717333));
#211615=CARTESIAN_POINT('Ctrl Pts',(-36.6147160117809,-79.2365278743448,
60.8270776080123));
#211616=CARTESIAN_POINT('Ctrl Pts',(-36.7123833980709,-83.032635108598,
62.9223801912564));
#211617=CARTESIAN_POINT('Ctrl Pts',(-36.8100507843609,-85.9182074332976,
66.1587663561375));
#211618=CARTESIAN_POINT('Ctrl Pts',(-36.9077181706509,-87.566152393697,
70.1693773391154));
#211619=CARTESIAN_POINT('Ctrl Pts',(-37.0053855569409,-87.7896681003677,
74.4995925506423));
#211620=CARTESIAN_POINT('Ctrl Pts',(-37.1030529432309,-86.5634180540064,
78.6585628406411));
#211621=CARTESIAN_POINT('Ctrl Pts',(-37.2007203295209,-84.0264031503354,
82.1748504323777));
#211622=CARTESIAN_POINT('Ctrl Pts',(-37.2983877158209,-80.4662053104341,
84.6498684909032));
#211623=CARTESIAN_POINT('Ctrl Pts',(-37.3960551021109,-76.2863887911529,
85.8030627132264));
#211624=CARTESIAN_POINT('Ctrl Pts',(-37.4937224884009,-71.9607543820079,
85.5037134061586));
#211625=CARTESIAN_POINT('Ctrl Pts',(-37.5913898746909,-67.9796319787588,
83.7857531448031));
#211626=CARTESIAN_POINT('Ctrl Pts',(-37.6890572609809,-64.7942995092932,
80.8439203643351));
#211627=CARTESIAN_POINT('Ctrl Pts',(-37.7867246472709,-62.7658285737666,
77.0116848923228));
#211628=CARTESIAN_POINT('Ctrl Pts',(-37.8843920335609,-62.1241553730382,
72.723447660932));
#211629=CARTESIAN_POINT('Ctrl Pts',(-37.9820594198509,-62.9420164178251,
68.4652994295259));
#211630=CARTESIAN_POINT('Ctrl Pts',(-38.0797268061409,-65.126703521839,
64.7199202355243));
#211631=CARTESIAN_POINT('Ctrl Pts',(-38.1773941924309,-68.4305726866551,
61.9118654657189));
#211632=CARTESIAN_POINT('Ctrl Pts',(-38.2750615787209,-72.479115651301,
60.359440615331));
#211633=CARTESIAN_POINT('Ctrl Pts',(-38.3727289650109,-76.8134120648424,
60.238619944442));
#211634=CARTESIAN_POINT('Ctrl Pts',(-38.4703963513009,-80.9421501644669,
61.5630990137955));
#211635=CARTESIAN_POINT('Ctrl Pts',(-38.5680637375909,-84.397319090609,
64.1827422295159));
#211636=CARTESIAN_POINT('Ctrl Pts',(-38.6657311238809,-86.7872602154302,
67.8006013898866));
#211637=CARTESIAN_POINT('Ctrl Pts',(-38.7633985101709,-87.8410625823901,
72.0065760486924));
#211638=CARTESIAN_POINT('Ctrl Pts',(-38.8610658964609,-87.4392748817876,
76.3239003581206));
#211639=CARTESIAN_POINT('Ctrl Pts',(-38.9587332827509,-85.6274345396819,
80.2631860989099));
#211640=CARTESIAN_POINT('Ctrl Pts',(-39.0564006690409,-82.6109478271435,
83.3778988728008));
#211641=CARTESIAN_POINT('Ctrl Pts',(-39.1540680553309,-78.7316494782208,
85.3149678148182));
#211642=CARTESIAN_POINT('Ctrl Pts',(-39.2191796461909,-75.8636424227415,
85.6748783876891));
#211643=CARTESIAN_POINT('Ctrl Pts',(-39.2517354416209,-74.4402359800407,
85.6117570961772));
#211644=CARTESIAN_POINT('Ctrl Pts',(-33.2251508293409,-79.9040287823937,
60.8783100640841));
#211645=CARTESIAN_POINT('Ctrl Pts',(-33.2577066247709,-81.2696674810732,
61.4313085050615));
#211646=CARTESIAN_POINT('Ctrl Pts',(-33.3228182156309,-83.811729992399,
63.0035716608669));
#211647=CARTESIAN_POINT('Ctrl Pts',(-33.4204856019209,-86.6262501677223,
66.49395799585));
#211648=CARTESIAN_POINT('Ctrl Pts',(-33.5181529882109,-88.1228094499778,
70.7205438274274));
#211649=CARTESIAN_POINT('Ctrl Pts',(-33.6158203745009,-88.1318596833692,
75.2042647157331));
#211650=CARTESIAN_POINT('Ctrl Pts',(-33.7134877607909,-86.6523499320974,
79.4368608152641));
#211651=CARTESIAN_POINT('Ctrl Pts',(-33.8111551470709,-83.8519959181997,
82.9385512545613));
#211652=CARTESIAN_POINT('Ctrl Pts',(-33.9088225333609,-80.0482284232973,
85.3124031224554));
#211653=CARTESIAN_POINT('Ctrl Pts',(-34.0064899196509,-75.6722218896999,
86.2893299487034));
#211654=CARTESIAN_POINT('Ctrl Pts',(-34.1041573059409,-71.2200159883432,
85.7585926810093));
#211655=CARTESIAN_POINT('Ctrl Pts',(-34.2018246922309,-67.1962880910714,
83.7803527627688));
#211656=CARTESIAN_POINT('Ctrl Pts',(-34.2994920785209,-64.0571456387238,
80.5788524819327));
#211657=CARTESIAN_POINT('Ctrl Pts',(-34.3971594648109,-62.1584243900869,
76.5169961329518));
#211658=CARTESIAN_POINT('Ctrl Pts',(-34.4948268511009,-61.7153528413655,
72.0552131952207));
#211659=CARTESIAN_POINT('Ctrl Pts',(-34.5924942373909,-62.7781551230735,
67.6992666057196));
#211660=CARTESIAN_POINT('Ctrl Pts',(-34.6901616236809,-65.2263578703911,
63.9429222806304));
#211661=CARTESIAN_POINT('Ctrl Pts',(-34.7878290099709,-68.7824464151142,
61.2119785531442));
#211662=CARTESIAN_POINT('Ctrl Pts',(-34.8854963962609,-73.0433223072712,
59.8160000388975));
#211663=CARTESIAN_POINT('Ctrl Pts',(-34.9831637825509,-77.5259963169692,
59.9132271101948));
#211664=CARTESIAN_POINT('Ctrl Pts',(-35.0808311688409,-81.7223374113863,
61.4926386461447));
#211665=CARTESIAN_POINT('Ctrl Pts',(-35.1784985551309,-85.1566716669334,
64.3752013257362));
#211666=CARTESIAN_POINT('Ctrl Pts',(-35.2761659414209,-87.43970202375,68.2341638508803));
#211667=CARTESIAN_POINT('Ctrl Pts',(-35.3738333277109,-88.3126368385637,
72.632095659094));
#211668=CARTESIAN_POINT('Ctrl Pts',(-35.4715007140009,-87.6765250683029,
77.0704716229308));
#211669=CARTESIAN_POINT('Ctrl Pts',(-35.5691681002909,-85.6034728108319,
81.0461820900503));
#211670=CARTESIAN_POINT('Ctrl Pts',(-35.6668354865809,-82.3284697580989,
84.1085625995896));
#211671=CARTESIAN_POINT('Ctrl Pts',(-35.7645028728709,-78.2227520696129,
85.9104787028144));
#211672=CARTESIAN_POINT('Ctrl Pts',(-35.8621702591609,-73.7517211029078,
86.2476751965479));
#211673=CARTESIAN_POINT('Ctrl Pts',(-35.9598376454509,-69.4221881001095,
85.0819293587689));
#211674=CARTESIAN_POINT('Ctrl Pts',(-36.0575050317409,-65.7249248799056,
82.545383664097));
#211675=CARTESIAN_POINT('Ctrl Pts',(-36.1551724180309,-63.0790326695276,
78.9255668466803));
#211676=CARTESIAN_POINT('Ctrl Pts',(-36.2528398043209,-61.7844351169188,
74.6328012395937));
#211677=CARTESIAN_POINT('Ctrl Pts',(-36.3505071906109,-61.9878806115566,
70.1536909137268));
#211678=CARTESIAN_POINT('Ctrl Pts',(-36.4481745769009,-63.666307701945,
65.995962942479));
#211679=CARTESIAN_POINT('Ctrl Pts',(-36.5458419631909,-66.6294592136506,
62.6309142802354));
#211680=CARTESIAN_POINT('Ctrl Pts',(-36.6435093494809,-70.5414487461066,
60.4399881567566));
#211681=CARTESIAN_POINT('Ctrl Pts',(-36.7411767357709,-74.9588348897375,
59.6715357908676));
#211682=CARTESIAN_POINT('Ctrl Pts',(-36.8388441220609,-79.3808872816728,
60.4126646754531));
#211683=CARTESIAN_POINT('Ctrl Pts',(-36.9365115083509,-83.3063466190444,
62.5793645557408));
#211684=CARTESIAN_POINT('Ctrl Pts',(-37.0341788946409,-86.2902446299875,
65.9260303652965));
#211685=CARTESIAN_POINT('Ctrl Pts',(-37.1318462809309,-87.994343206,70.0733026524509));
#211686=CARTESIAN_POINT('Ctrl Pts',(-37.2295136672209,-88.2254751955924,
74.5510696611245));
#211687=CARTESIAN_POINT('Ctrl Pts',(-37.3271810535109,-86.9574407599487,
78.8517565888795));
#211688=CARTESIAN_POINT('Ctrl Pts',(-37.4248484398009,-84.3339772411099,
82.4878614479098));
#211689=CARTESIAN_POINT('Ctrl Pts',(-37.5225158260909,-80.6524658951112,
85.0472155832));
#211690=CARTESIAN_POINT('Ctrl Pts',(-37.6201832123809,-76.3302224041847,
86.2397048224279));
#211691=CARTESIAN_POINT('Ctrl Pts',(-37.7178505986709,-71.857192288432,
85.9301552074926));
#211692=CARTESIAN_POINT('Ctrl Pts',(-37.8155179849609,-67.7404134024109,
84.1536555637811));
#211693=CARTESIAN_POINT('Ctrl Pts',(-37.9131853712509,-64.4465409395824,
81.1115800257429));
#211694=CARTESIAN_POINT('Ctrl Pts',(-38.0108527575409,-62.3489499909946,
77.1487613832986));
#211695=CARTESIAN_POINT('Ctrl Pts',(-38.1085201438309,-61.6854118183574,
72.7144027516668));
#211696=CARTESIAN_POINT('Ctrl Pts',(-38.2061875301209,-62.5311414241959,
68.3111584007035));
#211697=CARTESIAN_POINT('Ctrl Pts',(-38.3038549164109,-64.7902715968898,
64.4381556582015));
#211698=CARTESIAN_POINT('Ctrl Pts',(-38.4015223027009,-68.206719885141,
61.534416607706));
#211699=CARTESIAN_POINT('Ctrl Pts',(-38.4991896889909,-72.3932166837339,
59.9290929831488));
#211700=CARTESIAN_POINT('Ctrl Pts',(-38.5968570752809,-76.875203961106,
59.8041553558837));
#211701=CARTESIAN_POINT('Ctrl Pts',(-38.6945244615809,-81.1446285386002,
61.1737659619934));
#211702=CARTESIAN_POINT('Ctrl Pts',(-38.7921918478709,-84.7175321175373,
63.8826733471557));
#211703=CARTESIAN_POINT('Ctrl Pts',(-38.8898592341609,-87.1889103282383,
67.6238108193033));
#211704=CARTESIAN_POINT('Ctrl Pts',(-38.9875266204509,-88.2786209412064,
71.9731037866268));
#211705=CARTESIAN_POINT('Ctrl Pts',(-39.0851940067409,-87.8631423512599,
76.4375406365594));
#211706=CARTESIAN_POINT('Ctrl Pts',(-39.1828613930309,-85.9895636692369,
80.5110572786137));
#211707=CARTESIAN_POINT('Ctrl Pts',(-39.2805287793209,-82.8702903713335,
83.7319036844191));
#211708=CARTESIAN_POINT('Ctrl Pts',(-39.3781961656109,-78.8588051875596,
85.7349781226078));
#211709=CARTESIAN_POINT('Ctrl Pts',(-39.4433077564709,-75.8930709812184,
86.1071526244662));
#211710=CARTESIAN_POINT('Ctrl Pts',(-39.4758635519009,-74.4211620580609,
86.0418804791265));
#211711=CARTESIAN_POINT('Ctrl Pts',(-37.9553013365568,-62.9850802944281,
77.9529305295057));
#211712=CARTESIAN_POINT('Ctrl Pts',(-37.9474201705531,-63.1216095490577,
78.2833846866343));
#211713=CARTESIAN_POINT('Ctrl Pts',(-37.9395319063314,-63.271795121894,
78.6082626989507));
#211714=CARTESIAN_POINT('Ctrl Pts',(-37.9145482658144,-63.7864029611045,
79.6105293665822));
#211715=CARTESIAN_POINT('Ctrl Pts',(-37.8972687988449,-64.1974606125135,
80.2618535031525));
#211716=CARTESIAN_POINT('Ctrl Pts',(-37.8610792187594,-65.1847264324815,
81.5561899246955));
#211717=CARTESIAN_POINT('Ctrl Pts',(-37.8423433620313,-65.7722569016136,
82.1860084574922));
#211718=CARTESIAN_POINT('Ctrl Pts',(-37.8109478109972,-66.8312005758723,
83.1167677105313));
#211719=CARTESIAN_POINT('Ctrl Pts',(-37.7985886876602,-67.2674656454352,
83.4536451729963));
#211720=CARTESIAN_POINT('Ctrl Pts',(-37.7691084875777,-68.3637012594982,
84.1940605472006));
#211721=CARTESIAN_POINT('Ctrl Pts',(-37.752260997049,-69.0408691600133,
84.5684007187656));
#211722=CARTESIAN_POINT('Ctrl Pts',(-37.7176829609665,-70.4665992089544,
85.1981775476462));
#211723=CARTESIAN_POINT('Ctrl Pts',(-37.6999872682034,-71.2133015775831,
85.4500028177778));
#211724=CARTESIAN_POINT('Ctrl Pts',(-37.6640147271937,-72.78986964161,85.8267949841164));
#211725=CARTESIAN_POINT('Ctrl Pts',(-37.6457906302058,-73.6183716817423,
85.9421750277991));
#211726=CARTESIAN_POINT('Ctrl Pts',(-37.6179084997543,-74.8690218240065,
85.9949223926247));
#211727=CARTESIAN_POINT('Ctrl Pts',(-37.608565090223,-75.2864483781191,
85.9924272170315));
#211728=CARTESIAN_POINT('Ctrl Pts',(-37.5800013565997,-76.5622250903209,
85.9233331417926));
#211729=CARTESIAN_POINT('Ctrl Pts',(-37.561208726608,-77.4146797158845,
85.791611988895));
#211730=CARTESIAN_POINT('Ctrl Pts',(-37.5247928902469,-79.005561520104,
85.3811380147145));
#211731=CARTESIAN_POINT('Ctrl Pts',(-37.5072055842918,-79.7440710258465,
85.1176208937734));
#211732=CARTESIAN_POINT('Ctrl Pts',(-37.4706991061669,-81.2343611254123,
84.4287793423801));
#211733=CARTESIAN_POINT('Ctrl Pts',(-37.4519642982971,-81.9766763907336,
83.9918133103111));
#211734=CARTESIAN_POINT('Ctrl Pts',(-37.4235240123576,-83.0079247368912,
83.2381757820445));
#211735=CARTESIAN_POINT('Ctrl Pts',(-37.4141646745884,-83.3333225848237,
82.9754034813127));
#211736=CARTESIAN_POINT('Ctrl Pts',(-37.3855784673059,-84.2880441829575,
82.1252187149311));
#211737=CARTESIAN_POINT('Ctrl Pts',(-37.3667761154245,-84.8722039841866,
81.4906462028291));
#211738=CARTESIAN_POINT('Ctrl Pts',(-37.3288884631521,-85.900057666322,
80.1240524272387));
#211739=CARTESIAN_POINT('Ctrl Pts',(-37.3097661738678,-86.3429472217326,
79.3966463528337));
#211740=CARTESIAN_POINT('Ctrl Pts',(-37.2723777773446,-87.0746795871862,
77.8778102789801));
#211741=CARTESIAN_POINT('Ctrl Pts',(-37.2541052672179,-87.3641153421296,
77.0910954575695));
#211742=CARTESIAN_POINT('Ctrl Pts',(-37.2261946318884,-87.6814127958953,
75.8793939520376));
#211743=CARTESIAN_POINT('Ctrl Pts',(-37.216870478266,-87.7674530863341,
75.4719092966888));
#211744=CARTESIAN_POINT('Ctrl Pts',(-37.188334955032,-87.9709508310614,
74.2115296624505));
#211745=CARTESIAN_POINT('Ctrl Pts',(-37.1695528444446,-88.0234260694818,
73.3505374940313));
#211746=CARTESIAN_POINT('Ctrl Pts',(-37.1324546555661,-87.9593077821367,
71.6786479533309));
#211747=CARTESIAN_POINT('Ctrl Pts',(-37.1141663205998,-87.8520911218072,
70.8713112465121));
#211748=CARTESIAN_POINT('Ctrl Pts',(-37.0776055093155,-87.4832538348699,
69.265165449192));
#211749=CARTESIAN_POINT('Ctrl Pts',(-37.0593609396572,-87.2182658519536,
68.4709546004865));
#211750=CARTESIAN_POINT('Ctrl Pts',(-37.028756307801,-86.6601778752232,
67.2156601142761));
#211751=CARTESIAN_POINT('Ctrl Pts',(-37.0166706348671,-86.4110793261731,
66.7377142091686));
#211752=CARTESIAN_POINT('Ctrl Pts',(-36.9874851340614,-85.7347609734185,
65.6159671225058));
#211753=CARTESIAN_POINT('Ctrl Pts',(-36.9706554515717,-85.2784462954607,
64.9921013330032));
#211754=CARTESIAN_POINT('Ctrl Pts',(-36.9368299445691,-84.2726486204961,
63.8463944526631));
#211755=CARTESIAN_POINT('Ctrl Pts',(-36.9198965764989,-83.7275327721831,
63.3246569542117));
#211756=CARTESIAN_POINT('Ctrl Pts',(-36.8938644165587,-82.8143090573121,
62.5912253381851));
#211757=CARTESIAN_POINT('Ctrl Pts',(-36.8846757283285,-82.4758480186136,
62.3452743352519));
#211758=CARTESIAN_POINT('Ctrl Pts',(-36.8533476314567,-81.2877080817444,
61.5665594157926));
#211759=CARTESIAN_POINT('Ctrl Pts',(-36.8309230422989,-80.3885391871815,
61.1158732010766));
#211760=CARTESIAN_POINT('Ctrl Pts',(-36.7894494876858,-78.6387021441159,
60.4789344798652));
#211761=CARTESIAN_POINT('Ctrl Pts',(-36.7707178990796,-77.8036529097714,
60.2657349567428));
#211762=CARTESIAN_POINT('Ctrl Pts',(-36.7386712591883,-76.3794260285354,
60.0492377442393));
#211763=CARTESIAN_POINT('Ctrl Pts',(-36.7256353124818,-75.7999574332354,
60.0005305292947));
#211764=CARTESIAN_POINT('Ctrl Pts',(-36.6954200028567,-74.4448263249971,
59.9776797137621));
#211765=CARTESIAN_POINT('Ctrl Pts',(-36.6785226408525,-73.6708544423597,
60.033845272356));
#211766=CARTESIAN_POINT('Ctrl Pts',(-36.6444393144521,-72.1542417281374,
60.2813083751712));
#211767=CARTESIAN_POINT('Ctrl Pts',(-36.6273040887924,-71.4142410833303,
60.4699725635176));
#211768=CARTESIAN_POINT('Ctrl Pts',(-36.5912629985515,-69.8843497244514,
61.0068902560186));
#211769=CARTESIAN_POINT('Ctrl Pts',(-36.5725265787893,-69.1038501365627,
61.3710752108196));
#211770=CARTESIAN_POINT('Ctrl Pts',(-36.5440917128776,-68.0058455111706,
62.0227490315051));
#211771=CARTESIAN_POINT('Ctrl Pts',(-36.5347393239218,-67.6571704750053,
62.2530948298418));
#211772=CARTESIAN_POINT('Ctrl Pts',(-36.5061627867718,-66.6259532144554,
63.0081240836906));
#211773=CARTESIAN_POINT('Ctrl Pts',(-36.487364783741,-65.9838937259926,
63.5840945896985));
#211774=CARTESIAN_POINT('Ctrl Pts',(-36.4508287270761,-64.8716835789756,
64.8011777568565));
#211775=CARTESIAN_POINT('Ctrl Pts',(-36.4331132215708,-64.3939415100505,
65.4302567804368));
#211776=CARTESIAN_POINT('Ctrl Pts',(-36.3984301762417,-63.5673059184115,
66.7528247588843));
#211777=CARTESIAN_POINT('Ctrl Pts',(-36.3815971455736,-63.2175024656728,
67.4420206215753));
#211778=CARTESIAN_POINT('Ctrl Pts',(-36.3484649018998,-62.6632765516673,
68.8267002319811));
#211779=CARTESIAN_POINT('Ctrl Pts',(-36.3322686753649,-62.4516988960482,
69.5163260240136));
#211780=CARTESIAN_POINT('Ctrl Pts',(-36.3002569422527,-62.1447056281685,
70.9245458454321));
#211781=CARTESIAN_POINT('Ctrl Pts',(-36.2845007616004,-62.0499953695942,
71.6407444006773));
#211782=CARTESIAN_POINT('Ctrl Pts',(-36.2513677547303,-61.9779183273901,
73.1315272034695));
#211783=CARTESIAN_POINT('Ctrl Pts',(-36.2340081542753,-62.0093114894252,
73.903746883324));
#211784=CARTESIAN_POINT('Ctrl Pts',(-36.1994040444446,-62.2108802467661,
75.4506851127403));
#211785=CARTESIAN_POINT('Ctrl Pts',(-36.1821713308395,-62.3837445293686,
76.2218644194105));
#211786=CARTESIAN_POINT('Ctrl Pts',(-36.1568663165771,-62.7321991006185,
77.304263693113));
#211787=CARTESIAN_POINT('Ctrl Pts',(-36.1490816133291,-62.8521945973888,
77.6312952057894));
#211788=CARTESIAN_POINT('Ctrl Pts',(-36.1412950695185,-62.9850802944281,
77.9529305295057));
#211789=CARTESIAN_POINT('',(-32.7070373297029,-83.5022665033036,64.749780674319));
#211790=CARTESIAN_POINT('Ctrl Pts',(-26.5424658037409,-63.226796009855,
73.1405558201252));
#211791=CARTESIAN_POINT('Ctrl Pts',(-26.5750215991709,-63.2096934794613,
71.8129609505269));
#211792=CARTESIAN_POINT('Ctrl Pts',(-26.6401331900309,-63.6289072208686,
69.1522693813868));
#211793=CARTESIAN_POINT('Ctrl Pts',(-26.7378005763209,-65.5466883188414,
65.595862444819));
#211794=CARTESIAN_POINT('Ctrl Pts',(-26.8354679626109,-68.5360452568475,
62.8775596699701));
#211795=CARTESIAN_POINT('Ctrl Pts',(-26.9331353489009,-72.2581199618507,
61.3054018749864));
#211796=CARTESIAN_POINT('Ctrl Pts',(-27.0308027351909,-76.2909990282318,
61.0576244908063));
#211797=CARTESIAN_POINT('Ctrl Pts',(-27.1284701214809,-80.1775375961095,
62.1623076602056));
#211798=CARTESIAN_POINT('Ctrl Pts',(-27.2261375077709,-83.4771792584479,
64.4942323820704));
#211799=CARTESIAN_POINT('Ctrl Pts',(-27.3238048940609,-85.8158949537486,
67.789064150928));
#211800=CARTESIAN_POINT('Ctrl Pts',(-27.4214722803509,-86.9285808596196,
71.6733192596676));
#211801=CARTESIAN_POINT('Ctrl Pts',(-27.5191396666409,-86.6891090802536,
75.7067000853347));
#211802=CARTESIAN_POINT('Ctrl Pts',(-27.6168070529309,-85.1246248068445,
79.4320049844843));
#211803=CARTESIAN_POINT('Ctrl Pts',(-27.7144744392209,-82.4124692887962,
82.4269540784775));
#211804=CARTESIAN_POINT('Ctrl Pts',(-27.8121418255109,-78.860077414659,
84.3520565700369));
#211805=CARTESIAN_POINT('Ctrl Pts',(-27.9098092118009,-74.870128600351,
84.9890935309175));
#211806=CARTESIAN_POINT('Ctrl Pts',(-28.0074765980909,-70.8949012867121,
84.2658539888278));
#211807=CARTESIAN_POINT('Ctrl Pts',(-28.1051439843809,-67.3850051670203,
82.2643203620043));
#211808=CARTESIAN_POINT('Ctrl Pts',(-28.2028113706709,-64.7383025744529,
79.2113753875849));
#211809=CARTESIAN_POINT('Ctrl Pts',(-28.3004787569609,-63.254809017389,
75.453083954434));
#211810=CARTESIAN_POINT('Ctrl Pts',(-28.3981461432509,-63.1026850874199,
71.4154651090891));
#211811=CARTESIAN_POINT('Ctrl Pts',(-28.4958135295409,-64.2991747084623,
67.5562009023972));
#211812=CARTESIAN_POINT('Ctrl Pts',(-28.5934809158309,-66.7086504613652,
64.3127560937844));
#211813=CARTESIAN_POINT('Ctrl Pts',(-28.6911483021209,-70.0579875549346,
62.0527895754544));
#211814=CARTESIAN_POINT('Ctrl Pts',(-28.7888156884109,-73.9675237355834,
61.0324786020043));
#211815=CARTESIAN_POINT('Ctrl Pts',(-28.8864830747009,-77.994095692078,
61.367479959455));
#211816=CARTESIAN_POINT('Ctrl Pts',(-28.9841504609909,-81.6812735875568,
63.0198197542421));
#211817=CARTESIAN_POINT('Ctrl Pts',(-29.0818178472809,-84.6110994112092,
65.8021979228998));
#211818=CARTESIAN_POINT('Ctrl Pts',(-29.1794852335709,-86.4514643773875,
69.3992195271719));
#211819=CARTESIAN_POINT('Ctrl Pts',(-29.2771526198609,-86.99375493335,73.4031461727609));
#211820=CARTESIAN_POINT('Ctrl Pts',(-29.3748200061509,-86.176500033081,
77.3601149694952));
#211821=CARTESIAN_POINT('Ctrl Pts',(-29.4724873924409,-84.0923391537426,
80.8215859081834));
#211822=CARTESIAN_POINT('Ctrl Pts',(-29.5701547787309,-80.9775211989782,
83.3951858652538));
#211823=CARTESIAN_POINT('Ctrl Pts',(-29.6678221650209,-77.1851246351153,
84.789185841132));
#211824=CARTESIAN_POINT('Ctrl Pts',(-29.7654895513109,-73.1450344769205,
84.8455697396331));
#211825=CARTESIAN_POINT('Ctrl Pts',(-29.8631569376009,-69.3152129095361,
83.5579461951267));
#211826=CARTESIAN_POINT('Ctrl Pts',(-29.9608243238909,-66.1297872383019,
81.0722730622718));
#211827=CARTESIAN_POINT('Ctrl Pts',(-30.0584917101809,-63.9498396281978,
77.6703124441067));
#211828=CARTESIAN_POINT('Ctrl Pts',(-30.1561590964709,-63.0224768347345,
73.7376917047466));
#211829=CARTESIAN_POINT('Ctrl Pts',(-30.2538264827609,-63.4528195544114,
69.7201908928029));
#211830=CARTESIAN_POINT('Ctrl Pts',(-30.3514938690509,-65.1920865262802,
66.0732115905697));
#211831=CARTESIAN_POINT('Ctrl Pts',(-30.4491612553409,-68.0431241048049,
63.2101551195605));
#211832=CARTESIAN_POINT('Ctrl Pts',(-30.5468286416309,-71.6827545022938,
61.4555616623674));
#211833=CARTESIAN_POINT('Ctrl Pts',(-30.6444960279209,-75.6984094282703,
61.0083221897941));
#211834=CARTESIAN_POINT('Ctrl Pts',(-30.7421634142109,-79.634896539825,
61.9191332848712));
#211835=CARTESIAN_POINT('Ctrl Pts',(-30.8398308005009,-83.0459975178568,
64.0847504597221));
#211836=CARTESIAN_POINT('Ctrl Pts',(-30.9374981867909,-85.5450488978255,
67.2596913773822));
#211837=CARTESIAN_POINT('Ctrl Pts',(-31.0351655730809,-86.8487720928805,
71.0840623663197));
#211838=CARTESIAN_POINT('Ctrl Pts',(-31.1328329593709,-86.8093842813913,
75.1243539684997));
#211839=CARTESIAN_POINT('Ctrl Pts',(-31.2305003456609,-85.4313502469366,
78.9225811642113));
#211840=CARTESIAN_POINT('Ctrl Pts',(-31.3281677319509,-82.8708762752482,
82.0481980106353));
#211841=CARTESIAN_POINT('Ctrl Pts',(-31.4258351182409,-79.4182034770832,
84.1469019390542));
#211842=CARTESIAN_POINT('Ctrl Pts',(-31.5235025045309,-75.4647076676689,
84.980795526557));
#211843=CARTESIAN_POINT('Ctrl Pts',(-31.6211698908209,-71.4585351776186,
84.4553532267351));
#211844=CARTESIAN_POINT('Ctrl Pts',(-31.7188372771109,-67.8538034736301,
82.630136261015));
#211845=CARTESIAN_POINT('Ctrl Pts',(-31.8165046634009,-65.0591249238588,
79.712041088333));
#211846=CARTESIAN_POINT('Ctrl Pts',(-31.9141720496909,-63.3912887702861,
76.0318467751409));
#211847=CARTESIAN_POINT('Ctrl Pts',(-32.0118394359809,-63.0393516544576,
72.0067197036773));
#211848=CARTESIAN_POINT('Ctrl Pts',(-32.1095068222709,-64.0432072250839,
68.0929259582381));
#211849=CARTESIAN_POINT('Ctrl Pts',(-32.2071742085609,-66.2890639457993,
64.7341113461543));
#211850=CARTESIAN_POINT('Ctrl Pts',(-32.3048415948509,-69.5223441324314,
62.3110128795057));
#211851=CARTESIAN_POINT('Ctrl Pts',(-32.4025089811409,-73.3765404928114,
61.0982979039962));
#211852=CARTESIAN_POINT('Ctrl Pts',(-32.5001763674309,-77.4147649885621,
61.233439177867));
#211853=CARTESIAN_POINT('Ctrl Pts',(-32.5978437537209,-81.1792584882072,
62.7010949855073));
#211854=CARTESIAN_POINT('Ctrl Pts',(-32.6955111400109,-84.2433303651157,
65.3349852966984));
#211855=CARTESIAN_POINT('Ctrl Pts',(-32.7606227308709,-85.5874681664406,
67.6691475357372));
#211856=CARTESIAN_POINT('Ctrl Pts',(-32.7931785263009,-86.0468748830494,
68.9148385500206));
#211857=CARTESIAN_POINT('Ctrl Pts',(-26.7665939140209,-62.7962856369908,
73.1461018017394));
#211858=CARTESIAN_POINT('Ctrl Pts',(-26.7991497094509,-62.7785577189135,
71.7699608131093));
#211859=CARTESIAN_POINT('Ctrl Pts',(-26.8642613003109,-63.2131008357698,
69.0119758206586));
#211860=CARTESIAN_POINT('Ctrl Pts',(-26.9619286865909,-65.2010093736661,
65.3255218656522));
#211861=CARTESIAN_POINT('Ctrl Pts',(-27.0595960728809,-68.2996780309902,
62.5078190003945));
#211862=CARTESIAN_POINT('Ctrl Pts',(-27.1572634591709,-72.1578577224007,
60.8781721617226));
#211863=CARTESIAN_POINT('Ctrl Pts',(-27.2549308454609,-76.3382069483097,
60.6213343098834));
#211864=CARTESIAN_POINT('Ctrl Pts',(-27.3525982317509,-80.3668644473949,
61.766412393317));
#211865=CARTESIAN_POINT('Ctrl Pts',(-27.4502656180409,-83.787164000609,
64.1836085317263));
#211866=CARTESIAN_POINT('Ctrl Pts',(-27.5479330043309,-86.2113994377659,
67.5989223082413));
#211867=CARTESIAN_POINT('Ctrl Pts',(-27.6456003906209,-87.3647728934875,
71.6252128490111));
#211868=CARTESIAN_POINT('Ctrl Pts',(-27.7432677769109,-87.1165443572374,
75.8060821820241));
#211869=CARTESIAN_POINT('Ctrl Pts',(-27.8409351632009,-85.4948516375614,
79.6676101859858));
#211870=CARTESIAN_POINT('Ctrl Pts',(-27.9386025494909,-82.6835208156347,
82.7720754874777));
#211871=CARTESIAN_POINT('Ctrl Pts',(-28.0362699357809,-79.0012287417265,
84.7675731401279));
#211872=CARTESIAN_POINT('Ctrl Pts',(-28.1339373220709,-74.8653795970425,
85.4279046111302));
#211873=CARTESIAN_POINT('Ctrl Pts',(-28.2316047083609,-70.7447902736733,
84.6782183919009));
#211874=CARTESIAN_POINT('Ctrl Pts',(-28.3292720946509,-67.1065478950989,
82.6034947491145));
#211875=CARTESIAN_POINT('Ctrl Pts',(-28.4269394809409,-64.3630634136857,
79.4389128336908));
#211876=CARTESIAN_POINT('Ctrl Pts',(-28.5246068672309,-62.8253229952768,
75.543192078198));
#211877=CARTESIAN_POINT('Ctrl Pts',(-28.6222742535209,-62.6676363544306,
71.3579297539833));
#211878=CARTESIAN_POINT('Ctrl Pts',(-28.7199416398109,-63.9078779730934,
67.3575439567693));
#211879=CARTESIAN_POINT('Ctrl Pts',(-28.8176090261009,-66.4054609486044,
63.9954962058266));
#211880=CARTESIAN_POINT('Ctrl Pts',(-28.9152764123909,-69.8772731442938,
61.6528895642723));
#211881=CARTESIAN_POINT('Ctrl Pts',(-29.0129437986809,-73.9297692091192,
60.5952689121647));
#211882=CARTESIAN_POINT('Ctrl Pts',(-29.1106111849709,-78.1035806932568,
60.9425202535141));
#211883=CARTESIAN_POINT('Ctrl Pts',(-29.2082785712609,-81.9255875046266,
62.6552811046037));
#211884=CARTESIAN_POINT('Ctrl Pts',(-29.3059459575509,-84.9625481752439,
65.5394024065493));
#211885=CARTESIAN_POINT('Ctrl Pts',(-29.4036133438509,-86.8702097081482,
69.2679561845011));
#211886=CARTESIAN_POINT('Ctrl Pts',(-29.5012807301409,-87.4323301854809,
73.4182942873751));
#211887=CARTESIAN_POINT('Ctrl Pts',(-29.5989481164309,-86.5851907514749,
77.5199574352398));
#211888=CARTESIAN_POINT('Ctrl Pts',(-29.6966155027209,-84.4248184280816,
81.1080038707725));
#211889=CARTESIAN_POINT('Ctrl Pts',(-29.7942828890109,-81.1961010250256,
83.7757125749618));
#211890=CARTESIAN_POINT('Ctrl Pts',(-29.8919502753009,-77.2650280175932,
85.2206869032595));
#211891=CARTESIAN_POINT('Ctrl Pts',(-29.9896176615909,-73.0772040121119,
85.2791325899756));
#211892=CARTESIAN_POINT('Ctrl Pts',(-30.0872850478809,-69.1073374822569,
83.9444245566035));
#211893=CARTESIAN_POINT('Ctrl Pts',(-30.1849524341709,-65.8054304526251,
81.3678578939925));
#211894=CARTESIAN_POINT('Ctrl Pts',(-30.2826198204609,-63.5457687681484,
77.8414978909712));
#211895=CARTESIAN_POINT('Ctrl Pts',(-30.3802872067509,-62.5844951291497,
73.7650731351128));
#211896=CARTESIAN_POINT('Ctrl Pts',(-30.4779545930409,-63.0305741772578,
69.6006644997806));
#211897=CARTESIAN_POINT('Ctrl Pts',(-30.5756219793309,-64.8334408687264,
65.8203262223269));
#211898=CARTESIAN_POINT('Ctrl Pts',(-30.6732893656209,-67.7887322469773,
62.8525764571267));
#211899=CARTESIAN_POINT('Ctrl Pts',(-30.7709567519109,-71.5614528925225,
61.0338228372305));
#211900=CARTESIAN_POINT('Ctrl Pts',(-30.8686241382009,-75.7239481434376,
60.570229173206));
#211901=CARTESIAN_POINT('Ctrl Pts',(-30.9662915244909,-79.8043806529974,
61.5143458683933));
#211902=CARTESIAN_POINT('Ctrl Pts',(-31.0639589107809,-83.3402152511359,
63.7591530970452));
#211903=CARTESIAN_POINT('Ctrl Pts',(-31.1616262970709,-85.930649362801,
67.0501919774507));
#211904=CARTESIAN_POINT('Ctrl Pts',(-31.2592936833609,-87.2820457621323,
71.0144086177314));
#211905=CARTESIAN_POINT('Ctrl Pts',(-31.3569610696509,-87.2412176577989,
75.2024414334004));
#211906=CARTESIAN_POINT('Ctrl Pts',(-31.4546284559409,-85.8127930969901,
79.1395582812056));
#211907=CARTESIAN_POINT('Ctrl Pts',(-31.5522958422309,-83.1586903556685,
82.3794694586463));
#211908=CARTESIAN_POINT('Ctrl Pts',(-31.6499632285209,-79.5797637819886,
84.5549166263378));
#211909=CARTESIAN_POINT('Ctrl Pts',(-31.7476306148109,-75.4817006180579,
85.4193031739153));
#211910=CARTESIAN_POINT('Ctrl Pts',(-31.8452980011009,-71.329034547002,
84.8746470423661));
#211911=CARTESIAN_POINT('Ctrl Pts',(-31.9429653873909,-67.5924887343543,
82.98268742638));
#211912=CARTESIAN_POINT('Ctrl Pts',(-32.0406327736809,-64.695617263651,
79.9578863610724));
#211913=CARTESIAN_POINT('Ctrl Pts',(-32.1383001599709,-62.9667933989244,
76.1431185004145));
#211914=CARTESIAN_POINT('Ctrl Pts',(-32.2359675462609,-62.6019870098559,
71.970804736377));
#211915=CARTESIAN_POINT('Ctrl Pts',(-32.3336349325509,-63.642550534956,
67.9138954205205));
#211916=CARTESIAN_POINT('Ctrl Pts',(-32.4313023188409,-65.9705314263782,
64.4322591422073));
#211917=CARTESIAN_POINT('Ctrl Pts',(-32.5289697051309,-69.3220428659327,
61.9205553116032));
#211918=CARTESIAN_POINT('Ctrl Pts',(-32.6266370914209,-73.3171755010594,
60.6634950264663));
#211919=CARTESIAN_POINT('Ctrl Pts',(-32.7243044777109,-77.5030656224803,
60.8035780069626));
#211920=CARTESIAN_POINT('Ctrl Pts',(-32.8219718640009,-81.4052152352389,
62.3249015374696));
#211921=CARTESIAN_POINT('Ctrl Pts',(-32.9196392502909,-84.5813309302388,
65.0551052312263));
#211922=CARTESIAN_POINT('Ctrl Pts',(-32.9847508411509,-85.974619775455,
67.4746207060263));
#211923=CARTESIAN_POINT('Ctrl Pts',(-33.0173066365809,-86.4508256027431,
68.7658628636918));
#211924=CARTESIAN_POINT('Ctrl Pts',(-26.9907220242909,-62.3657752641363,
73.1516477833507));
#211925=CARTESIAN_POINT('Ctrl Pts',(-27.0232778197209,-62.3474219583749,
71.7269606756879));
#211926=CARTESIAN_POINT('Ctrl Pts',(-27.0883894105809,-62.7972944506722,
68.8716822599311));
#211927=CARTESIAN_POINT('Ctrl Pts',(-27.1860567968709,-64.8553304284946,
65.0551812864947));
#211928=CARTESIAN_POINT('Ctrl Pts',(-27.2837241831609,-68.0633108051291,
62.1380783308097));
#211929=CARTESIAN_POINT('Ctrl Pts',(-27.3813915694509,-72.0575954829508,
60.4509424484588));
#211930=CARTESIAN_POINT('Ctrl Pts',(-27.4790589557409,-76.3854148683847,
60.1850441289508));
#211931=CARTESIAN_POINT('Ctrl Pts',(-27.5767263420309,-80.5561912986817,
61.3705171264288));
#211932=CARTESIAN_POINT('Ctrl Pts',(-27.6743937283209,-84.0971487427805,
63.8729846813812));
#211933=CARTESIAN_POINT('Ctrl Pts',(-27.7720611146109,-86.6069039217849,
67.4087804655587));
#211934=CARTESIAN_POINT('Ctrl Pts',(-27.8697285009009,-87.8009649273485,
71.577106438364));
#211935=CARTESIAN_POINT('Ctrl Pts',(-27.9673958871909,-87.5439796342222,
75.9054642787186));
#211936=CARTESIAN_POINT('Ctrl Pts',(-28.0650632734809,-85.8650784682753,
79.9032153874961));
#211937=CARTESIAN_POINT('Ctrl Pts',(-28.1627306597709,-82.9545723424687,
83.1171968964905));
#211938=CARTESIAN_POINT('Ctrl Pts',(-28.2603980460609,-79.1423800687866,
85.1830897102328));
#211939=CARTESIAN_POINT('Ctrl Pts',(-28.3580654323509,-74.860630593725,
85.8667156913575));
#211940=CARTESIAN_POINT('Ctrl Pts',(-28.4557328186409,-70.5946792606203,
85.0905827949681));
#211941=CARTESIAN_POINT('Ctrl Pts',(-28.5534002049309,-66.8280906231621,
82.9426691362138));
#211942=CARTESIAN_POINT('Ctrl Pts',(-28.6510675912209,-63.987824252902,
79.666450279783));
#211943=CARTESIAN_POINT('Ctrl Pts',(-28.7487349775109,-62.3958369731654,
75.6333002019378));
#211944=CARTESIAN_POINT('Ctrl Pts',(-28.8464023638009,-62.2325876214517,
71.3003943988505));
#211945=CARTESIAN_POINT('Ctrl Pts',(-28.9440697500909,-63.5165812377356,
67.1588870111186));
#211946=CARTESIAN_POINT('Ctrl Pts',(-29.0417371363809,-66.1022714358647,
63.6782363178492));
#211947=CARTESIAN_POINT('Ctrl Pts',(-29.1394045226709,-69.6965587336775,
61.2529895530693));
#211948=CARTESIAN_POINT('Ctrl Pts',(-29.2370719089609,-73.8920146826892,
60.1580592223219));
#211949=CARTESIAN_POINT('Ctrl Pts',(-29.3347392952509,-78.2130656944676,
60.5175605475773));
#211950=CARTESIAN_POINT('Ctrl Pts',(-29.4324066815409,-82.1699014217328,
62.2907424549826));
#211951=CARTESIAN_POINT('Ctrl Pts',(-29.5300740678309,-85.3139969393028,
65.2766068902311));
#211952=CARTESIAN_POINT('Ctrl Pts',(-29.6277414541209,-87.2889550389062,
69.1366928418757));
#211953=CARTESIAN_POINT('Ctrl Pts',(-29.7254088404109,-87.8709054376088,
73.4334424020349));
#211954=CARTESIAN_POINT('Ctrl Pts',(-29.8230762267009,-86.9938814698514,
77.6797999010284));
#211955=CARTESIAN_POINT('Ctrl Pts',(-29.9207436129909,-84.7572977023885,
81.3944218333964));
#211956=CARTESIAN_POINT('Ctrl Pts',(-30.0184109992809,-81.4146808510287,
84.1562392846881));
#211957=CARTESIAN_POINT('Ctrl Pts',(-30.1160783855709,-77.3449314000249,
85.652187965406));
#211958=CARTESIAN_POINT('Ctrl Pts',(-30.2137457718609,-73.009373547253,
85.7126954403171));
#211959=CARTESIAN_POINT('Ctrl Pts',(-30.3114131581509,-68.8994620549307,
84.3309029180553));
#211960=CARTESIAN_POINT('Ctrl Pts',(-30.4090805444409,-65.4810736669192,
81.6634427256689));
#211961=CARTESIAN_POINT('Ctrl Pts',(-30.5067479307309,-63.1416979080774,
78.0126833377833));
#211962=CARTESIAN_POINT('Ctrl Pts',(-30.6044153170209,-62.1465134235629,
73.7924545654214));
#211963=CARTESIAN_POINT('Ctrl Pts',(-30.7020827033109,-62.6083288001179,
69.4811381067028));
#211964=CARTESIAN_POINT('Ctrl Pts',(-30.7997500896009,-64.4747952112035,
65.5674408540281));
#211965=CARTESIAN_POINT('Ctrl Pts',(-30.8974174758909,-67.5343403891965,
62.4949977946519));
#211966=CARTESIAN_POINT('Ctrl Pts',(-30.9950848621809,-71.4401512828104,
60.6120840120799));
#211967=CARTESIAN_POINT('Ctrl Pts',(-31.0927522484709,-75.7494868586634,
60.1321361566154));
#211968=CARTESIAN_POINT('Ctrl Pts',(-31.1904196347609,-79.973864766225,
61.1095584519391));
#211969=CARTESIAN_POINT('Ctrl Pts',(-31.2880870210509,-83.6344329844545,
63.4335557344114));
#211970=CARTESIAN_POINT('Ctrl Pts',(-31.3857544073409,-86.3162498277991,
66.8406925775738));
#211971=CARTESIAN_POINT('Ctrl Pts',(-31.4834217936309,-87.7153194313877,
70.9447548692043));
#211972=CARTESIAN_POINT('Ctrl Pts',(-31.5810891799209,-87.6730510341971,
75.2805288983569));
#211973=CARTESIAN_POINT('Ctrl Pts',(-31.6787565662109,-86.1942359470167,
79.3565353982501));
#211974=CARTESIAN_POINT('Ctrl Pts',(-31.7764239525009,-83.4465044360485,
82.7107409066955));
#211975=CARTESIAN_POINT('Ctrl Pts',(-31.8740913387909,-79.7413240868408,
84.9629313136325));
#211976=CARTESIAN_POINT('Ctrl Pts',(-31.9717587250809,-75.4986935683949,
85.8578108212734));
#211977=CARTESIAN_POINT('Ctrl Pts',(-32.0694261113709,-71.1995339163389,
85.2939408579817));
#211978=CARTESIAN_POINT('Ctrl Pts',(-32.1670934976609,-67.331173995054,
83.335238591712));
#211979=CARTESIAN_POINT('Ctrl Pts',(-32.2647608839509,-64.3321096034271,
80.203731633773));
#211980=CARTESIAN_POINT('Ctrl Pts',(-32.3624282702409,-62.5422980275575,
76.2543902256492));
#211981=CARTESIAN_POINT('Ctrl Pts',(-32.4600956565309,-62.1646223652701,
71.9348897690366));
#211982=CARTESIAN_POINT('Ctrl Pts',(-32.5577630428209,-63.2418938448422,
67.7348648827743));
#211983=CARTESIAN_POINT('Ctrl Pts',(-32.6554304291109,-65.6519989069735,
64.1304069382318));
#211984=CARTESIAN_POINT('Ctrl Pts',(-32.7530978154009,-69.1217415994551,
61.5300977436921));
#211985=CARTESIAN_POINT('Ctrl Pts',(-32.8507652016909,-73.2578105093222,
60.2286921489302));
#211986=CARTESIAN_POINT('Ctrl Pts',(-32.9484325879809,-77.5913662564109,
60.373716836065));
#211987=CARTESIAN_POINT('Ctrl Pts',(-33.0460999742709,-81.6311719822709,
61.948708089435));
#211988=CARTESIAN_POINT('Ctrl Pts',(-33.1437673605609,-84.9193314953615,
64.7752251657533));
#211989=CARTESIAN_POINT('Ctrl Pts',(-33.2088789514209,-86.3617713844579,
67.2800938763135));
#211990=CARTESIAN_POINT('Ctrl Pts',(-33.2414347468509,-86.8547763224244,
68.616887177359));
#211991=CARTESIAN_POINT('Ctrl Pts',(-27.2148501345709,-61.9352648912724,
73.1571937649659));
#211992=CARTESIAN_POINT('Ctrl Pts',(-27.2474059300009,-61.9162861978364,
71.6839605382664));
#211993=CARTESIAN_POINT('Ctrl Pts',(-27.3125175208609,-62.3814880655743,
68.7313886992026));
#211994=CARTESIAN_POINT('Ctrl Pts',(-27.4101849071509,-64.5096514833231,
64.7848407073371));
#211995=CARTESIAN_POINT('Ctrl Pts',(-27.5078522934409,-67.8269435792709,
61.7683376612345));
#211996=CARTESIAN_POINT('Ctrl Pts',(-27.6055196797309,-71.9573332435009,
60.023712735195));
#211997=CARTESIAN_POINT('Ctrl Pts',(-27.7031870660209,-76.4326227884626,
59.7487539480279));
#211998=CARTESIAN_POINT('Ctrl Pts',(-27.8008544523109,-80.7455181499671,
60.9746218595402));
#211999=CARTESIAN_POINT('Ctrl Pts',(-27.8985218386009,-84.4071334849508,
63.5623608310333));
#212000=CARTESIAN_POINT('Ctrl Pts',(-27.9961892248909,-87.0024084058022,
67.2186386228721));
#212001=CARTESIAN_POINT('Ctrl Pts',(-28.0938566111809,-88.2371569612167,
71.5290000277085));
#212002=CARTESIAN_POINT('Ctrl Pts',(-28.1915239974709,-87.9714149112048,
76.0048463754075));
#212003=CARTESIAN_POINT('Ctrl Pts',(-28.2891913837609,-86.2353052989911,
80.1388205889948));
#212004=CARTESIAN_POINT('Ctrl Pts',(-28.3868587700509,-83.225623869312,
83.4623183054996));
#212005=CARTESIAN_POINT('Ctrl Pts',(-28.4845261563409,-79.2835313958541,
85.5986062803239));
#212006=CARTESIAN_POINT('Ctrl Pts',(-28.5821935426309,-74.8558815904194,
86.3055267715799));
#212007=CARTESIAN_POINT('Ctrl Pts',(-28.6798609289209,-70.4445682475821,
85.5029471980399));
#212008=CARTESIAN_POINT('Ctrl Pts',(-28.7775283152109,-66.5496333512407,
83.281843523324));
#212009=CARTESIAN_POINT('Ctrl Pts',(-28.8751957015009,-63.6125850921352,
79.8939877258898));
#212010=CARTESIAN_POINT('Ctrl Pts',(-28.9728630877909,-61.9663509510528,
75.7234083257008));
#212011=CARTESIAN_POINT('Ctrl Pts',(-29.0705304740809,-61.7975388884712,
71.24285904374));
#212012=CARTESIAN_POINT('Ctrl Pts',(-29.1681978603709,-63.125284502366,
66.9602300654889));
#212013=CARTESIAN_POINT('Ctrl Pts',(-29.2658652466609,-65.799081923101,
63.3609764298818));
#212014=CARTESIAN_POINT('Ctrl Pts',(-29.3635326329509,-69.5158443230372,
60.8530895418871));
#212015=CARTESIAN_POINT('Ctrl Pts',(-29.4612000192409,-73.8542601562259,
59.720849532482));
#212016=CARTESIAN_POINT('Ctrl Pts',(-29.5588674055309,-78.3225506956497,
60.0926008416416));
#212017=CARTESIAN_POINT('Ctrl Pts',(-29.6565347918209,-82.4142153388091,
61.9262038053415));
#212018=CARTESIAN_POINT('Ctrl Pts',(-29.7542021781109,-85.6654457033379,
65.0138113738816));
#212019=CARTESIAN_POINT('Ctrl Pts',(-29.8518695644009,-87.7077003696673,
69.0054294992058));
#212020=CARTESIAN_POINT('Ctrl Pts',(-29.9495369506909,-88.3094806897396,
73.4485905166491));
#212021=CARTESIAN_POINT('Ctrl Pts',(-30.0472043369809,-87.4025721882447,
77.8396423667743));
#212022=CARTESIAN_POINT('Ctrl Pts',(-30.1448717232709,-85.0897769767237,
81.6808397959762));
#212023=CARTESIAN_POINT('Ctrl Pts',(-30.2425391095609,-81.6332606770752,
84.5367659943965));
#212024=CARTESIAN_POINT('Ctrl Pts',(-30.3402064958509,-77.4248347825067,
86.0836890275427));
#212025=CARTESIAN_POINT('Ctrl Pts',(-30.4378738821409,-72.9415430824435,
86.14625829066));
#212026=CARTESIAN_POINT('Ctrl Pts',(-30.5355412684309,-68.6915866276478,
84.7173812795336));
#212027=CARTESIAN_POINT('Ctrl Pts',(-30.6332086547209,-65.1567168812421,
81.9590275573886));
#212028=CARTESIAN_POINT('Ctrl Pts',(-30.7308760410109,-62.7376270480277,
78.183868784647));
#212029=CARTESIAN_POINT('Ctrl Pts',(-30.8285434273009,-61.7085317179689,
73.8198359957914));
#212030=CARTESIAN_POINT('Ctrl Pts',(-30.9262108135909,-62.1860834229676,
69.361611713678));
#212031=CARTESIAN_POINT('Ctrl Pts',(-31.0238781998809,-64.1161495536497,
65.3145554857853));
#212032=CARTESIAN_POINT('Ctrl Pts',(-31.1215455861709,-67.2799485313697,
62.1374191322177));
#212033=CARTESIAN_POINT('Ctrl Pts',(-31.2192129724609,-71.3188496730437,
60.1903451869519));
#212034=CARTESIAN_POINT('Ctrl Pts',(-31.3168803587509,-75.7750255738315,
59.6940431400269));
#212035=CARTESIAN_POINT('Ctrl Pts',(-31.4145477450409,-80.1433488793987,
60.7047710354617));
#212036=CARTESIAN_POINT('Ctrl Pts',(-31.5122151313309,-83.9286507177339,
63.1079583717354));
#212037=CARTESIAN_POINT('Ctrl Pts',(-31.6098825176209,-86.7018502927658,
66.6311931776471));
#212038=CARTESIAN_POINT('Ctrl Pts',(-31.7075499039109,-88.1485931006402,
70.8751011206178));
#212039=CARTESIAN_POINT('Ctrl Pts',(-31.8052172902009,-88.1048844106144,
75.3586163632546));
#212040=CARTESIAN_POINT('Ctrl Pts',(-31.9028846764909,-86.575678797071,
79.5735125152463));
#212041=CARTESIAN_POINT('Ctrl Pts',(-32.0005520627809,-83.7343185164689,
83.0420123547065));
#212042=CARTESIAN_POINT('Ctrl Pts',(-32.0982194490709,-79.9028843917455,
85.3709460009163));
#212043=CARTESIAN_POINT('Ctrl Pts',(-32.1958868353609,-75.5156865187867,
86.2963184686414));
#212044=CARTESIAN_POINT('Ctrl Pts',(-32.2935542216509,-71.0700332857199,
85.7132346736072));
#212045=CARTESIAN_POINT('Ctrl Pts',(-32.3912216079409,-67.0698592557778,
83.6877897570761));
#212046=CARTESIAN_POINT('Ctrl Pts',(-32.4888889942309,-63.9686019432188,
80.4495769065115));
#212047=CARTESIAN_POINT('Ctrl Pts',(-32.5865563805209,-62.1178026561958,
76.3656619509228));
#212048=CARTESIAN_POINT('Ctrl Pts',(-32.6842237668109,-61.7272577206776,
71.8989748017325));
#212049=CARTESIAN_POINT('Ctrl Pts',(-32.7818911531009,-62.8412371547143,
67.5558343450567));
#212050=CARTESIAN_POINT('Ctrl Pts',(-32.8795585393909,-65.3334663875495,
63.8285547342751));
#212051=CARTESIAN_POINT('Ctrl Pts',(-32.9772259256809,-68.9214403329571,
61.1396401757894));
#212052=CARTESIAN_POINT('Ctrl Pts',(-33.0748933119709,-73.1984455175702,
59.7938892714003));
#212053=CARTESIAN_POINT('Ctrl Pts',(-33.1725606982609,-77.6796668903304,
59.9438556651611));
#212054=CARTESIAN_POINT('Ctrl Pts',(-33.2702280845509,-81.8571287293036,
61.5725146413969));
#212055=CARTESIAN_POINT('Ctrl Pts',(-33.3678954708409,-85.2573320604846,
64.4953451002813));
#212056=CARTESIAN_POINT('Ctrl Pts',(-33.4330070617009,-86.7489229934631,
67.0855670466063));
#212057=CARTESIAN_POINT('Ctrl Pts',(-33.4655628571309,-87.2587270421088,
68.4679114910338));
#212058=CARTESIAN_POINT('',(-26.6970235948769,-64.1107820886051,68.3402936518987));
#212059=CARTESIAN_POINT('Ctrl Pts',(-22.3657263431209,-78.9572065659953,
84.0781567697157));
#212060=CARTESIAN_POINT('Ctrl Pts',(-22.4113638359009,-77.2042658920752,
84.7036938863734));
#212061=CARTESIAN_POINT('Ctrl Pts',(-22.5026388214709,-73.3978907787715,
85.1071590883939));
#212062=CARTESIAN_POINT('Ctrl Pts',(-22.6395512998309,-68.0405685475501,
83.0382494769742));
#212063=CARTESIAN_POINT('Ctrl Pts',(-22.7764637781809,-64.2196078175175,
78.7512421293735));
#212064=CARTESIAN_POINT('Ctrl Pts',(-22.9133762565409,-62.7778618409869,
73.1924757376221));
#212065=CARTESIAN_POINT('Ctrl Pts',(-23.0502887348909,-64.0336581279753,
67.5887670194206));
#212066=CARTESIAN_POINT('Ctrl Pts',(-23.1872012132509,-67.7098000647524,
63.1769076868417));
#212067=CARTESIAN_POINT('Ctrl Pts',(-23.3241136916009,-72.9949448440006,
60.930624514091));
#212068=CARTESIAN_POINT('Ctrl Pts',(-23.4610261699609,-78.7226196025488,
61.3456896355516));
#212069=CARTESIAN_POINT('Ctrl Pts',(-23.5979386483109,-83.6286848555507,
64.3304948862028));
#212070=CARTESIAN_POINT('Ctrl Pts',(-23.7348511266709,-86.6303355967727,
69.226271763487));
#212071=CARTESIAN_POINT('Ctrl Pts',(-23.8717636050209,-87.0650853842986,
74.9524861359762));
#212072=CARTESIAN_POINT('Ctrl Pts',(-24.0086760833809,-84.83698171689,80.2453202044371));
#212073=CARTESIAN_POINT('Ctrl Pts',(-24.1455885617309,-80.4377835331297,
83.9366063979646));
#212074=CARTESIAN_POINT('Ctrl Pts',(-24.2825010400909,-74.8384263620678,
85.2116505915669));
#212075=CARTESIAN_POINT('Ctrl Pts',(-24.4194135184409,-69.2747296862646,
83.7890411146377));
#212076=CARTESIAN_POINT('Ctrl Pts',(-24.5563259967909,-64.9746424533178,
79.9827583856073));
#212077=CARTESIAN_POINT('Ctrl Pts',(-24.6932384751509,-62.8872256743196,
74.6328771144893));
#212078=CARTESIAN_POINT('Ctrl Pts',(-24.8301509535009,-63.4731876492382,
68.920155609978));
#212079=CARTESIAN_POINT('Ctrl Pts',(-24.9670634318609,-66.6032022425639,
64.105433700007));
#212080=CARTESIAN_POINT('Ctrl Pts',(-25.1039759102109,-71.5864521163174,
61.251356069971));
#212081=CARTESIAN_POINT('Ctrl Pts',(-25.2408883885709,-77.3230972196102,
60.9878387312059));
#212082=CARTESIAN_POINT('Ctrl Pts',(-25.3778008669209,-82.5470176072806,
63.3730419092899));
#212083=CARTESIAN_POINT('Ctrl Pts',(-25.5147133452809,-86.1052554762516,
67.8805336366521));
#212084=CARTESIAN_POINT('Ctrl Pts',(-25.6516258236309,-87.212481417992,
73.5154772357479));
#212085=CARTESIAN_POINT('Ctrl Pts',(-25.7885383019909,-85.6243226056579,
79.0341988976569));
#212086=CARTESIAN_POINT('Ctrl Pts',(-25.9254507803409,-81.6912969855573,
83.2186765115833));
#212087=CARTESIAN_POINT('Ctrl Pts',(-26.0623632587009,-76.2814539762174,
85.1453630258059));
#212088=CARTESIAN_POINT('Ctrl Pts',(-26.1992757370509,-70.5887798524084,
84.3890317273547));
#212089=CARTESIAN_POINT('Ctrl Pts',(-26.3361882154009,-65.8697123503377,
81.116583535284));
#212090=CARTESIAN_POINT('Ctrl Pts',(-26.4731006937609,-63.1657005004853,
76.05037264205));
#212091=CARTESIAN_POINT('Ctrl Pts',(-26.6100131721109,-63.0738532573673,
70.3081733636108));
#212092=CARTESIAN_POINT('Ctrl Pts',(-26.7012881576809,-64.7667989074192,
66.8752138971438));
#212093=CARTESIAN_POINT('Ctrl Pts',(-26.7469256504709,-65.9591325242604,
65.446074912737));
#212094=CARTESIAN_POINT('Ctrl Pts',(-22.5898544533909,-79.1019096116296,
84.483657654596));
#212095=CARTESIAN_POINT('Ctrl Pts',(-22.6354919461809,-77.2848692122853,
85.1320687669441));
#212096=CARTESIAN_POINT('Ctrl Pts',(-22.7267669317509,-73.339306502245,
85.5502874680714));
#212097=CARTESIAN_POINT('Ctrl Pts',(-22.8636794101009,-67.7860832407449,
83.405724105221));
#212098=CARTESIAN_POINT('Ctrl Pts',(-23.0005918884609,-63.8254015621982,
78.9619538973823));
#212099=CARTESIAN_POINT('Ctrl Pts',(-23.1375043668109,-62.3309353067667,
73.1999202731971));
#212100=CARTESIAN_POINT('Ctrl Pts',(-23.2744168451709,-63.6326522563196,
67.391300917951));
#212101=CARTESIAN_POINT('Ctrl Pts',(-23.4113293235209,-67.4432195574419,
62.8181132666061));
#212102=CARTESIAN_POINT('Ctrl Pts',(-23.5482418018809,-72.921626056387,
60.4896903290827));
#212103=CARTESIAN_POINT('Ctrl Pts',(-23.6851542802309,-78.8587445142041,
60.9199331235345));
#212104=CARTESIAN_POINT('Ctrl Pts',(-23.8220667585909,-83.9442096980268,
64.0138836520905));
#212105=CARTESIAN_POINT('Ctrl Pts',(-23.9589792369409,-87.0556217056703,
69.088684245488));
#212106=CARTESIAN_POINT('Ctrl Pts',(-24.0958917153009,-87.5062689747379,
75.0242889153553));
#212107=CARTESIAN_POINT('Ctrl Pts',(-24.2328041936509,-85.1966903119605,
80.5106658775061));
#212108=CARTESIAN_POINT('Ctrl Pts',(-24.3697166720109,-80.6366267892543,
84.3369312149314));
#212109=CARTESIAN_POINT('Ctrl Pts',(-24.5066291503609,-74.8325181040322,
85.6585999086832));
#212110=CARTESIAN_POINT('Ctrl Pts',(-24.6435416287209,-69.0653739102596,
84.1839699166283));
#212111=CARTESIAN_POINT('Ctrl Pts',(-24.7804541070709,-64.6080455253229,
80.2385029690766));
#212112=CARTESIAN_POINT('Ctrl Pts',(-24.9173665854309,-62.4442982438864,
74.6929927610358));
#212113=CARTESIAN_POINT('Ctrl Pts',(-25.0542790637809,-63.0516870715546,
68.7713743524177));
#212114=CARTESIAN_POINT('Ctrl Pts',(-25.1911915421409,-66.2961568081638,
63.7805926607206));
#212115=CARTESIAN_POINT('Ctrl Pts',(-25.3281040204909,-71.4616290202873,
60.8221500654866));
#212116=CARTESIAN_POINT('Ctrl Pts',(-25.4650164988409,-77.408045841156,
60.5489966966417));
#212117=CARTESIAN_POINT('Ctrl Pts',(-25.6019289772009,-82.822989158162,
63.0214195228689));
#212118=CARTESIAN_POINT('Ctrl Pts',(-25.7388414555509,-86.5113409972175,
67.6937365557131));
#212119=CARTESIAN_POINT('Ctrl Pts',(-25.8757539339109,-87.6590548344714,
73.5347329567422));
#212120=CARTESIAN_POINT('Ctrl Pts',(-26.0126664122609,-86.0128218697664,
79.255257536733));
#212121=CARTESIAN_POINT('Ctrl Pts',(-26.1495788906209,-81.9359774279065,
83.5927488094103));
#212122=CARTESIAN_POINT('Ctrl Pts',(-26.2864913689709,-76.328312862688,
85.5898884076402));
#212123=CARTESIAN_POINT('Ctrl Pts',(-26.4234038473309,-70.4274749066969,
84.8059003668431));
#212124=CARTESIAN_POINT('Ctrl Pts',(-26.5603163256809,-65.5358454145695,
81.413788666648));
#212125=CARTESIAN_POINT('Ctrl Pts',(-26.6972288040409,-62.73295605009,76.1623218021048));
#212126=CARTESIAN_POINT('Ctrl Pts',(-26.8341412823909,-62.6377502317761,
70.2101477067446));
#212127=CARTESIAN_POINT('Ctrl Pts',(-26.9254162679609,-64.3926017711426,
66.6516553215257));
#212128=CARTESIAN_POINT('Ctrl Pts',(-26.9710537607409,-65.6285354131264,
65.170257057697));
#212129=CARTESIAN_POINT('Ctrl Pts',(-22.8139825636709,-79.2466126572418,
84.8891585394854));
#212130=CARTESIAN_POINT('Ctrl Pts',(-22.8596200564509,-77.3654725324694,
85.5604436475147));
#212131=CARTESIAN_POINT('Ctrl Pts',(-22.9508950420209,-73.2807222256896,
85.9934158477393));
#212132=CARTESIAN_POINT('Ctrl Pts',(-23.0878075203809,-67.5315979339206,
83.7731987334475));
#212133=CARTESIAN_POINT('Ctrl Pts',(-23.2247199987309,-63.4311953068659,
79.1726656653596));
#212134=CARTESIAN_POINT('Ctrl Pts',(-23.3616324770909,-61.8840087725427,
73.2073648087369));
#212135=CARTESIAN_POINT('Ctrl Pts',(-23.4985449554409,-63.2316463846813,
67.193834816445));
#212136=CARTESIAN_POINT('Ctrl Pts',(-23.6354574338009,-67.1766390501634,
62.4593188463355));
#212137=CARTESIAN_POINT('Ctrl Pts',(-23.7723699121509,-72.8483072688198,
60.0487561440661));
#212138=CARTESIAN_POINT('Ctrl Pts',(-23.9092823905109,-78.9948694259072,
60.4941766115334));
#212139=CARTESIAN_POINT('Ctrl Pts',(-24.0461948688609,-84.2597345405397,
63.6972724180149));
#212140=CARTESIAN_POINT('Ctrl Pts',(-24.1831073472209,-87.4809078145793,
68.9510967275428));
#212141=CARTESIAN_POINT('Ctrl Pts',(-24.3200198255709,-87.9474525651767,
75.0960916947856));
#212142=CARTESIAN_POINT('Ctrl Pts',(-24.4569323039309,-85.5563989069964,
80.776011550622));
#212143=CARTESIAN_POINT('Ctrl Pts',(-24.5938447822809,-80.835470045328,
84.7372560319301));
#212144=CARTESIAN_POINT('Ctrl Pts',(-24.7307572606409,-74.8266098459419,
86.1055492258111));
#212145=CARTESIAN_POINT('Ctrl Pts',(-24.8676697389909,-68.8560181341975,
84.5788987185906));
#212146=CARTESIAN_POINT('Ctrl Pts',(-25.0045822173509,-64.2414485972866,
80.4942475524981));
#212147=CARTESIAN_POINT('Ctrl Pts',(-25.1414946957009,-62.0013708134489,
74.7531084075192));
#212148=CARTESIAN_POINT('Ctrl Pts',(-25.2784071740609,-62.6301864938922,
68.6225930947988));
#212149=CARTESIAN_POINT('Ctrl Pts',(-25.4153196524109,-65.9891113738079,
63.4557516213943));
#212150=CARTESIAN_POINT('Ctrl Pts',(-25.5522321307709,-71.3368059243146,
60.3929440609893));
#212151=CARTESIAN_POINT('Ctrl Pts',(-25.6891446091209,-77.4929944627566,
60.1101546620874));
#212152=CARTESIAN_POINT('Ctrl Pts',(-25.8260570874809,-83.0989607090898,
62.6697971364817));
#212153=CARTESIAN_POINT('Ctrl Pts',(-25.9629695658309,-86.9174265182033,
67.5069394748223));
#212154=CARTESIAN_POINT('Ctrl Pts',(-26.0998820441809,-88.1056282509491,
73.5539886777848));
#212155=CARTESIAN_POINT('Ctrl Pts',(-26.2367945225409,-86.4013211338496,
79.4763161758422));
#212156=CARTESIAN_POINT('Ctrl Pts',(-26.3737070008909,-82.1806578702273,
83.9668211072705));
#212157=CARTESIAN_POINT('Ctrl Pts',(-26.5106194792509,-76.3751717491205,
86.0344137894687));
#212158=CARTESIAN_POINT('Ctrl Pts',(-26.6475319576009,-70.2661699609606,
85.2227690063212));
#212159=CARTESIAN_POINT('Ctrl Pts',(-26.7844444359609,-65.2019784787844,
81.7109937979974));
#212160=CARTESIAN_POINT('Ctrl Pts',(-26.9213569143109,-62.3002115996993,
76.2742709621448));
#212161=CARTESIAN_POINT('Ctrl Pts',(-27.0582693926709,-62.2016472061933,
70.1121220498728));
#212162=CARTESIAN_POINT('Ctrl Pts',(-27.1495443782409,-64.0184046348646,
66.4280967459093));
#212163=CARTESIAN_POINT('Ctrl Pts',(-27.1951818710209,-65.2979383019839,
64.8944392026497));
#212164=CARTESIAN_POINT('Ctrl Pts',(-23.0381106739509,-79.391315702872,
85.2946594243565));
#212165=CARTESIAN_POINT('Ctrl Pts',(-23.0837481667309,-77.4460758526756,
85.9888185280761));
#212166=CARTESIAN_POINT('Ctrl Pts',(-23.1750231523009,-73.2221379491631,
86.4365442274168));
#212167=CARTESIAN_POINT('Ctrl Pts',(-23.3119356306609,-67.2771126271247,
84.1406733616905));
#212168=CARTESIAN_POINT('Ctrl Pts',(-23.4488481090109,-63.0369890515466,
79.3833774333684));
#212169=CARTESIAN_POINT('Ctrl Pts',(-23.5857605873609,-61.4370822383221,
73.2148093443111));
#212170=CARTESIAN_POINT('Ctrl Pts',(-23.7226730657209,-62.830640513026,
66.9963687149763));
#212171=CARTESIAN_POINT('Ctrl Pts',(-23.8595855440709,-66.9100585428538,
62.1005244260995));
#212172=CARTESIAN_POINT('Ctrl Pts',(-23.9964980224309,-72.774988481211,
59.6078219590666));
#212173=CARTESIAN_POINT('Ctrl Pts',(-24.1334105007809,-79.1309943375632,
60.0684200995181));
#212174=CARTESIAN_POINT('Ctrl Pts',(-24.2703229791409,-84.5752593830162,
63.3806611839035));
#212175=CARTESIAN_POINT('Ctrl Pts',(-24.4072354574909,-87.9061939234772,
68.8135092095445));
#212176=CARTESIAN_POINT('Ctrl Pts',(-24.5441479358509,-88.3886361556165,
75.1678944741656));
#212177=CARTESIAN_POINT('Ctrl Pts',(-24.6810604142009,-85.9161075020708,
81.0413572237003));
#212178=CARTESIAN_POINT('Ctrl Pts',(-24.8179728925609,-81.0343133014518,
85.1375808488973));
#212179=CARTESIAN_POINT('Ctrl Pts',(-24.9548853709109,-74.8207015879063,
86.5524985429274));
#212180=CARTESIAN_POINT('Ctrl Pts',(-25.0917978492709,-68.6466623581968,
84.9738275205784));
#212181=CARTESIAN_POINT('Ctrl Pts',(-25.2287103276209,-63.8748516692914,
80.7499921359665));
#212182=CARTESIAN_POINT('Ctrl Pts',(-25.3656228059809,-61.5584433830157,
74.8132240540657));
#212183=CARTESIAN_POINT('Ctrl Pts',(-25.5025352843309,-62.2086859162091,
68.4738118372371));
#212184=CARTESIAN_POINT('Ctrl Pts',(-25.6394477626909,-65.6820659394125,
63.1309105821168));
#212185=CARTESIAN_POINT('Ctrl Pts',(-25.7763602410409,-71.2119828282853,
59.9637380565046));
#212186=CARTESIAN_POINT('Ctrl Pts',(-25.9132727194009,-77.5779430843033,
59.6713126275229));
#212187=CARTESIAN_POINT('Ctrl Pts',(-26.0501851977509,-83.3749322599808,
62.3181747500578));
#212188=CARTESIAN_POINT('Ctrl Pts',(-26.1870976761109,-87.3235120391694,
67.3201423938839));
#212189=CARTESIAN_POINT('Ctrl Pts',(-26.3240101544609,-88.5522016674284,
73.5732443987791));
#212190=CARTESIAN_POINT('Ctrl Pts',(-26.4609226328209,-86.7898203979605,
79.697374814927));
#212191=CARTESIAN_POINT('Ctrl Pts',(-26.5978351111709,-82.4253383125765,
84.3408934050975));
#212192=CARTESIAN_POINT('Ctrl Pts',(-26.7347475895209,-76.4220306355901,
86.4789391713034));
#212193=CARTESIAN_POINT('Ctrl Pts',(-26.8716600678809,-70.1048650152488,
85.6396376458087));
#212194=CARTESIAN_POINT('Ctrl Pts',(-27.0085725462309,-64.8681115430162,
82.0081989293614));
#212195=CARTESIAN_POINT('Ctrl Pts',(-27.1454850245909,-61.8674671493036,
76.3862201221987));
#212196=CARTESIAN_POINT('Ctrl Pts',(-27.2823975029409,-61.7655441806113,
70.0140963930029));
#212197=CARTESIAN_POINT('Ctrl Pts',(-27.3736724885109,-63.6442074985899,
66.2045381702958));
#212198=CARTESIAN_POINT('Ctrl Pts',(-27.4193099813009,-64.967341190849,
64.6186213476101));
#212199=CARTESIAN_POINT('',(-22.5674166601918,-72.2136650090823,84.4952548267707));
#212200=CARTESIAN_POINT('Ctrl Pts',(-22.5675364832709,-72.213605770789,
84.4954770366417));
#212201=CARTESIAN_POINT('Ctrl Pts',(-22.5675364832709,-72.7621512638099,
84.6563729599098));
#212202=CARTESIAN_POINT('Ctrl Pts',(-22.5675364832727,-73.3221605020505,
84.7774848925876));
#212203=CARTESIAN_POINT('Ctrl Pts',(-22.5675364832727,-74.4604827599086,
84.9369083570789));
#212204=CARTESIAN_POINT('Ctrl Pts',(-22.5675364832709,-75.0358317053909,
84.9749462493133));
#212205=CARTESIAN_POINT('Ctrl Pts',(-22.5675364832709,-75.6109582839319,
84.971915110047));
#212206=CARTESIAN_POINT('Ctrl Pts',(-22.5674166601918,-72.213719011673,
84.4950313516973));
#212207=CARTESIAN_POINT('Ctrl Pts',(-22.5674566012175,-72.2106294569051,
84.4942847630103));
#212208=CARTESIAN_POINT('Ctrl Pts',(-22.5674965422431,-72.2075402027097,
84.4935369402495));
#212209=CARTESIAN_POINT('Ctrl Pts',(-22.5675364832687,-72.2044512501038,
84.4927878836052));
#212210=CARTESIAN_POINT('Origin',(-21.6548258024609,-75.,72.98888938658));
#212211=CARTESIAN_POINT('Ctrl Pts',(-25.6386080251009,-61.9352648912724,
73.1571937649659));
#212212=CARTESIAN_POINT('Ctrl Pts',(-25.6711638205309,-61.9162861978364,
71.6839605382664));
#212213=CARTESIAN_POINT('Ctrl Pts',(-25.7362754113909,-62.3814880655743,
68.7313886992026));
#212214=CARTESIAN_POINT('Ctrl Pts',(-25.8339427976809,-64.5096514833231,
64.7848407073371));
#212215=CARTESIAN_POINT('Ctrl Pts',(-25.9316101839709,-67.8269435792709,
61.7683376612345));
#212216=CARTESIAN_POINT('Ctrl Pts',(-26.0292775702609,-71.9573332435009,
60.023712735195));
#212217=CARTESIAN_POINT('Ctrl Pts',(-26.1269449565509,-76.4326227884626,
59.7487539480279));
#212218=CARTESIAN_POINT('Ctrl Pts',(-26.2246123428409,-80.7455181499671,
60.9746218595402));
#212219=CARTESIAN_POINT('Ctrl Pts',(-26.3222797291309,-84.4071334849508,
63.5623608310333));
#212220=CARTESIAN_POINT('Ctrl Pts',(-26.4199471154209,-87.0024084058022,
67.2186386228721));
#212221=CARTESIAN_POINT('Ctrl Pts',(-26.5176145017109,-88.2371569612167,
71.5290000277085));
#212222=CARTESIAN_POINT('Ctrl Pts',(-26.6152818880009,-87.9714149112048,
76.0048463754075));
#212223=CARTESIAN_POINT('Ctrl Pts',(-26.7129492742909,-86.2353052989911,
80.1388205889948));
#212224=CARTESIAN_POINT('Ctrl Pts',(-26.8106166605809,-83.225623869312,
83.4623183054996));
#212225=CARTESIAN_POINT('Ctrl Pts',(-26.9082840468709,-79.2835313958541,
85.5986062803239));
#212226=CARTESIAN_POINT('Ctrl Pts',(-27.0059514331609,-74.8558815904194,
86.3055267715799));
#212227=CARTESIAN_POINT('Ctrl Pts',(-27.1036188194509,-70.4445682475821,
85.5029471980399));
#212228=CARTESIAN_POINT('Ctrl Pts',(-27.2012862057409,-66.5496333512407,
83.281843523324));
#212229=CARTESIAN_POINT('Ctrl Pts',(-27.2989535920309,-63.6125850921352,
79.8939877258898));
#212230=CARTESIAN_POINT('Ctrl Pts',(-27.3966209783209,-61.9663509510528,
75.7234083257008));
#212231=CARTESIAN_POINT('Ctrl Pts',(-27.4942883646109,-61.7975388884712,
71.24285904374));
#212232=CARTESIAN_POINT('Ctrl Pts',(-27.5919557509009,-63.125284502366,
66.9602300654889));
#212233=CARTESIAN_POINT('Ctrl Pts',(-27.6896231371909,-65.799081923101,
63.3609764298818));
#212234=CARTESIAN_POINT('Ctrl Pts',(-27.7872905234809,-69.5158443230372,
60.8530895418871));
#212235=CARTESIAN_POINT('Ctrl Pts',(-27.8849579097709,-73.8542601562259,
59.720849532482));
#212236=CARTESIAN_POINT('Ctrl Pts',(-27.9826252960609,-78.3225506956497,
60.0926008416416));
#212237=CARTESIAN_POINT('Ctrl Pts',(-28.0802926823509,-82.4142153388091,
61.9262038053415));
#212238=CARTESIAN_POINT('Ctrl Pts',(-28.1779600686409,-85.6654457033379,
65.0138113738816));
#212239=CARTESIAN_POINT('Ctrl Pts',(-28.2756274549309,-87.7077003696673,
69.0054294992058));
#212240=CARTESIAN_POINT('Ctrl Pts',(-28.3732948412209,-88.3094806897396,
73.4485905166491));
#212241=CARTESIAN_POINT('Ctrl Pts',(-28.4709622275109,-87.4025721882447,
77.8396423667743));
#212242=CARTESIAN_POINT('Ctrl Pts',(-28.5686296138009,-85.0897769767237,
81.6808397959762));
#212243=CARTESIAN_POINT('Ctrl Pts',(-28.6662970000909,-81.6332606770752,
84.5367659943965));
#212244=CARTESIAN_POINT('Ctrl Pts',(-28.7639643863809,-77.4248347825067,
86.0836890275427));
#212245=CARTESIAN_POINT('Ctrl Pts',(-28.8616317726709,-72.9415430824435,
86.14625829066));
#212246=CARTESIAN_POINT('Ctrl Pts',(-28.9592991589609,-68.6915866276478,
84.7173812795336));
#212247=CARTESIAN_POINT('Ctrl Pts',(-29.0569665452509,-65.1567168812421,
81.9590275573886));
#212248=CARTESIAN_POINT('Ctrl Pts',(-29.1546339315409,-62.7376270480277,
78.183868784647));
#212249=CARTESIAN_POINT('Ctrl Pts',(-29.2523013178309,-61.7085317179689,
73.8198359957914));
#212250=CARTESIAN_POINT('Ctrl Pts',(-29.3499687041209,-62.1860834229676,
69.361611713678));
#212251=CARTESIAN_POINT('Ctrl Pts',(-29.4476360904109,-64.1161495536497,
65.3145554857853));
#212252=CARTESIAN_POINT('Ctrl Pts',(-29.5453034767009,-67.2799485313697,
62.1374191322177));
#212253=CARTESIAN_POINT('Ctrl Pts',(-29.6429708629909,-71.3188496730437,
60.1903451869519));
#212254=CARTESIAN_POINT('Ctrl Pts',(-29.7406382492809,-75.7750255738315,
59.6940431400269));
#212255=CARTESIAN_POINT('Ctrl Pts',(-29.8383056355709,-80.1433488793987,
60.7047710354617));
#212256=CARTESIAN_POINT('Ctrl Pts',(-29.9359730218609,-83.9286507177339,
63.1079583717354));
#212257=CARTESIAN_POINT('Ctrl Pts',(-30.0336404081509,-86.7018502927658,
66.6311931776471));
#212258=CARTESIAN_POINT('Ctrl Pts',(-30.1313077944409,-88.1485931006402,
70.8751011206178));
#212259=CARTESIAN_POINT('Ctrl Pts',(-30.2289751807309,-88.1048844106144,
75.3586163632546));
#212260=CARTESIAN_POINT('Ctrl Pts',(-30.3266425670209,-86.575678797071,
79.5735125152463));
#212261=CARTESIAN_POINT('Ctrl Pts',(-30.4243099533109,-83.7343185164689,
83.0420123547065));
#212262=CARTESIAN_POINT('Ctrl Pts',(-30.5219773396009,-79.9028843917455,
85.3709460009163));
#212263=CARTESIAN_POINT('Ctrl Pts',(-30.6196447258909,-75.5156865187867,
86.2963184686414));
#212264=CARTESIAN_POINT('Ctrl Pts',(-30.7173121121809,-71.0700332857199,
85.7132346736072));
#212265=CARTESIAN_POINT('Ctrl Pts',(-30.8149794984709,-67.0698592557778,
83.6877897570761));
#212266=CARTESIAN_POINT('Ctrl Pts',(-30.9126468847609,-63.9686019432188,
80.4495769065115));
#212267=CARTESIAN_POINT('Ctrl Pts',(-31.0103142710509,-62.1178026561954,
76.3656619509219));
#212268=CARTESIAN_POINT('Ctrl Pts',(-31.1079816573409,-61.7272577206776,
71.8989748017325));
#212269=CARTESIAN_POINT('Ctrl Pts',(-31.2056490436309,-62.8412371547143,
67.5558343450567));
#212270=CARTESIAN_POINT('Ctrl Pts',(-31.3033164299209,-65.3334663875495,
63.8285547342751));
#212271=CARTESIAN_POINT('Ctrl Pts',(-31.4009838162109,-68.9214403329571,
61.1396401757894));
#212272=CARTESIAN_POINT('Ctrl Pts',(-31.4986512025009,-73.1984455175702,
59.7938892714003));
#212273=CARTESIAN_POINT('Ctrl Pts',(-31.5963185887909,-77.6796668903304,
59.9438556651611));
#212274=CARTESIAN_POINT('Ctrl Pts',(-31.6939859750809,-81.8571287293036,
61.5725146413969));
#212275=CARTESIAN_POINT('Ctrl Pts',(-31.7916533613709,-85.2573320604846,
64.4953451002813));
#212276=CARTESIAN_POINT('Ctrl Pts',(-31.8567649522309,-86.7489229934631,
67.0855670466063));
#212277=CARTESIAN_POINT('Ctrl Pts',(-31.8893207476609,-87.2587270421088,
68.4679114910338));
#212278=CARTESIAN_POINT('Ctrl Pts',(-25.8627361353809,-62.3657752641363,
73.1516477833507));
#212279=CARTESIAN_POINT('Ctrl Pts',(-25.8952919308109,-62.3474219583749,
71.7269606756879));
#212280=CARTESIAN_POINT('Ctrl Pts',(-25.9604035216709,-62.7972944506722,
68.8716822599311));
#212281=CARTESIAN_POINT('Ctrl Pts',(-26.0580709079509,-64.8553304284946,
65.0551812864947));
#212282=CARTESIAN_POINT('Ctrl Pts',(-26.1557382942409,-68.0633108051291,
62.1380783308097));
#212283=CARTESIAN_POINT('Ctrl Pts',(-26.2534056805309,-72.0575954829508,
60.4509424484588));
#212284=CARTESIAN_POINT('Ctrl Pts',(-26.3510730668209,-76.3854148683847,
60.1850441289508));
#212285=CARTESIAN_POINT('Ctrl Pts',(-26.4487404531109,-80.5561912986817,
61.3705171264288));
#212286=CARTESIAN_POINT('Ctrl Pts',(-26.5464078394009,-84.0971487427805,
63.8729846813812));
#212287=CARTESIAN_POINT('Ctrl Pts',(-26.6440752256909,-86.6069039217849,
67.4087804655587));
#212288=CARTESIAN_POINT('Ctrl Pts',(-26.7417426119809,-87.8009649273485,
71.577106438364));
#212289=CARTESIAN_POINT('Ctrl Pts',(-26.8394099982709,-87.5439796342222,
75.9054642787186));
#212290=CARTESIAN_POINT('Ctrl Pts',(-26.9370773845609,-85.8650784682753,
79.9032153874961));
#212291=CARTESIAN_POINT('Ctrl Pts',(-27.0347447708509,-82.9545723424687,
83.1171968964905));
#212292=CARTESIAN_POINT('Ctrl Pts',(-27.1324121571409,-79.1423800687866,
85.1830897102328));
#212293=CARTESIAN_POINT('Ctrl Pts',(-27.2300795434309,-74.860630593725,
85.8667156913575));
#212294=CARTESIAN_POINT('Ctrl Pts',(-27.3277469297209,-70.5946792606203,
85.0905827949681));
#212295=CARTESIAN_POINT('Ctrl Pts',(-27.4254143160109,-66.8280906231621,
82.9426691362138));
#212296=CARTESIAN_POINT('Ctrl Pts',(-27.5230817023009,-63.9878242529024,
79.6664502797839));
#212297=CARTESIAN_POINT('Ctrl Pts',(-27.6207490885909,-62.3958369731654,
75.6333002019378));
#212298=CARTESIAN_POINT('Ctrl Pts',(-27.7184164748809,-62.2325876214517,
71.3003943988505));
#212299=CARTESIAN_POINT('Ctrl Pts',(-27.8160838611709,-63.5165812377356,
67.1588870111186));
#212300=CARTESIAN_POINT('Ctrl Pts',(-27.9137512474609,-66.1022714358647,
63.6782363178492));
#212301=CARTESIAN_POINT('Ctrl Pts',(-28.0114186337509,-69.6965587336775,
61.2529895530693));
#212302=CARTESIAN_POINT('Ctrl Pts',(-28.1090860200409,-73.8920146826892,
60.1580592223219));
#212303=CARTESIAN_POINT('Ctrl Pts',(-28.2067534063309,-78.2130656944676,
60.5175605475773));
#212304=CARTESIAN_POINT('Ctrl Pts',(-28.3044207926209,-82.1699014217328,
62.2907424549826));
#212305=CARTESIAN_POINT('Ctrl Pts',(-28.4020881789109,-85.3139969393028,
65.2766068902311));
#212306=CARTESIAN_POINT('Ctrl Pts',(-28.4997555652109,-87.2889550389062,
69.1366928418757));
#212307=CARTESIAN_POINT('Ctrl Pts',(-28.5974229515009,-87.8709054376088,
73.4334424020349));
#212308=CARTESIAN_POINT('Ctrl Pts',(-28.6950903377909,-86.9938814698514,
77.6797999010284));
#212309=CARTESIAN_POINT('Ctrl Pts',(-28.7927577240809,-84.7572977023885,
81.3944218333964));
#212310=CARTESIAN_POINT('Ctrl Pts',(-28.8904251103709,-81.4146808510287,
84.1562392846881));
#212311=CARTESIAN_POINT('Ctrl Pts',(-28.9880924966609,-77.3449314000249,
85.652187965406));
#212312=CARTESIAN_POINT('Ctrl Pts',(-29.0857598829509,-73.009373547253,
85.7126954403171));
#212313=CARTESIAN_POINT('Ctrl Pts',(-29.1834272692409,-68.8994620549307,
84.3309029180553));
#212314=CARTESIAN_POINT('Ctrl Pts',(-29.2810946555309,-65.4810736669192,
81.6634427256689));
#212315=CARTESIAN_POINT('Ctrl Pts',(-29.3787620418209,-63.1416979080774,
78.0126833377833));
#212316=CARTESIAN_POINT('Ctrl Pts',(-29.4764294281109,-62.1465134235629,
73.7924545654214));
#212317=CARTESIAN_POINT('Ctrl Pts',(-29.5740968144009,-62.6083288001179,
69.4811381067028));
#212318=CARTESIAN_POINT('Ctrl Pts',(-29.6717642006909,-64.4747952112035,
65.5674408540281));
#212319=CARTESIAN_POINT('Ctrl Pts',(-29.7694315869809,-67.5343403891965,
62.4949977946519));
#212320=CARTESIAN_POINT('Ctrl Pts',(-29.8670989732709,-71.4401512828104,
60.6120840120799));
#212321=CARTESIAN_POINT('Ctrl Pts',(-29.9647663595609,-75.7494868586634,
60.1321361566154));
#212322=CARTESIAN_POINT('Ctrl Pts',(-30.0624337458509,-79.973864766225,
61.1095584519391));
#212323=CARTESIAN_POINT('Ctrl Pts',(-30.1601011321409,-83.6344329844545,
63.4335557344114));
#212324=CARTESIAN_POINT('Ctrl Pts',(-30.2577685184309,-86.3162498277991,
66.8406925775738));
#212325=CARTESIAN_POINT('Ctrl Pts',(-30.3554359047209,-87.7153194313877,
70.9447548692043));
#212326=CARTESIAN_POINT('Ctrl Pts',(-30.4531032910109,-87.6730510341971,
75.2805288983569));
#212327=CARTESIAN_POINT('Ctrl Pts',(-30.5507706773009,-86.1942359470167,
79.3565353982501));
#212328=CARTESIAN_POINT('Ctrl Pts',(-30.6484380635909,-83.4465044360485,
82.7107409066955));
#212329=CARTESIAN_POINT('Ctrl Pts',(-30.7461054498809,-79.7413240868409,
84.9629313136324));
#212330=CARTESIAN_POINT('Ctrl Pts',(-30.8437728361709,-75.4986935683949,
85.8578108212734));
#212331=CARTESIAN_POINT('Ctrl Pts',(-30.9414402224609,-71.1995339163389,
85.2939408579817));
#212332=CARTESIAN_POINT('Ctrl Pts',(-31.0391076087509,-67.331173995054,
83.335238591712));
#212333=CARTESIAN_POINT('Ctrl Pts',(-31.1367749950409,-64.3321096034267,
80.2037316337721));
#212334=CARTESIAN_POINT('Ctrl Pts',(-31.2344423813309,-62.5422980275575,
76.2543902256492));
#212335=CARTESIAN_POINT('Ctrl Pts',(-31.3321097676209,-62.1646223652701,
71.9348897690366));
#212336=CARTESIAN_POINT('Ctrl Pts',(-31.4297771539109,-63.2418938448422,
67.7348648827743));
#212337=CARTESIAN_POINT('Ctrl Pts',(-31.5274445402009,-65.6519989069735,
64.1304069382318));
#212338=CARTESIAN_POINT('Ctrl Pts',(-31.6251119264909,-69.1217415994551,
61.5300977436921));
#212339=CARTESIAN_POINT('Ctrl Pts',(-31.7227793127809,-73.2578105093222,
60.2286921489302));
#212340=CARTESIAN_POINT('Ctrl Pts',(-31.8204466990709,-77.5913662564109,
60.373716836065));
#212341=CARTESIAN_POINT('Ctrl Pts',(-31.9181140853609,-81.6311719822709,
61.948708089435));
#212342=CARTESIAN_POINT('Ctrl Pts',(-32.0157814716509,-84.9193314953615,
64.7752251657533));
#212343=CARTESIAN_POINT('Ctrl Pts',(-32.0808930625109,-86.3617713844579,
67.2800938763135));
#212344=CARTESIAN_POINT('Ctrl Pts',(-32.1134488579409,-86.8547763224244,
68.616887177359));
#212345=CARTESIAN_POINT('Ctrl Pts',(-26.0868642456509,-62.7962856369908,
73.1461018017394));
#212346=CARTESIAN_POINT('Ctrl Pts',(-26.1194200410809,-62.7785577189135,
71.7699608131093));
#212347=CARTESIAN_POINT('Ctrl Pts',(-26.1845316319409,-63.2131008357698,
69.0119758206586));
#212348=CARTESIAN_POINT('Ctrl Pts',(-26.2821990182309,-65.2010093736661,
65.3255218656522));
#212349=CARTESIAN_POINT('Ctrl Pts',(-26.3798664045209,-68.2996780309902,
62.5078190003945));
#212350=CARTESIAN_POINT('Ctrl Pts',(-26.4775337908109,-72.1578577224007,
60.8781721617226));
#212351=CARTESIAN_POINT('Ctrl Pts',(-26.5752011771009,-76.3382069483097,
60.6213343098834));
#212352=CARTESIAN_POINT('Ctrl Pts',(-26.6728685633909,-80.3668644473949,
61.766412393317));
#212353=CARTESIAN_POINT('Ctrl Pts',(-26.7705359496809,-83.787164000609,
64.1836085317263));
#212354=CARTESIAN_POINT('Ctrl Pts',(-26.8682033359709,-86.2113994377659,
67.5989223082413));
#212355=CARTESIAN_POINT('Ctrl Pts',(-26.9658707222609,-87.3647728934875,
71.6252128490111));
#212356=CARTESIAN_POINT('Ctrl Pts',(-27.0635381085509,-87.1165443572374,
75.8060821820241));
#212357=CARTESIAN_POINT('Ctrl Pts',(-27.1612054948409,-85.4948516375614,
79.6676101859858));
#212358=CARTESIAN_POINT('Ctrl Pts',(-27.2588728811309,-82.6835208156347,
82.7720754874777));
#212359=CARTESIAN_POINT('Ctrl Pts',(-27.3565402674209,-79.0012287417265,
84.7675731401279));
#212360=CARTESIAN_POINT('Ctrl Pts',(-27.4542076537109,-74.8653795970425,
85.4279046111302));
#212361=CARTESIAN_POINT('Ctrl Pts',(-27.5518750400009,-70.7447902736733,
84.6782183919009));
#212362=CARTESIAN_POINT('Ctrl Pts',(-27.6495424262909,-67.1065478950989,
82.6034947491145));
#212363=CARTESIAN_POINT('Ctrl Pts',(-27.7472098125809,-64.3630634136857,
79.4389128336908));
#212364=CARTESIAN_POINT('Ctrl Pts',(-27.8448771988709,-62.8253229952768,
75.543192078198));
#212365=CARTESIAN_POINT('Ctrl Pts',(-27.9425445851609,-62.6676363544306,
71.3579297539833));
#212366=CARTESIAN_POINT('Ctrl Pts',(-28.0402119714509,-63.9078779730934,
67.3575439567693));
#212367=CARTESIAN_POINT('Ctrl Pts',(-28.1378793577409,-66.4054609486044,
63.9954962058266));
#212368=CARTESIAN_POINT('Ctrl Pts',(-28.2355467440309,-69.8772731442938,
61.6528895642723));
#212369=CARTESIAN_POINT('Ctrl Pts',(-28.3332141303209,-73.9297692091192,
60.5952689121647));
#212370=CARTESIAN_POINT('Ctrl Pts',(-28.4308815166109,-78.1035806932568,
60.9425202535141));
#212371=CARTESIAN_POINT('Ctrl Pts',(-28.5285489029009,-81.9255875046266,
62.6552811046037));
#212372=CARTESIAN_POINT('Ctrl Pts',(-28.6262162891909,-84.9625481752439,
65.5394024065493));
#212373=CARTESIAN_POINT('Ctrl Pts',(-28.7238836754809,-86.8702097081482,
69.2679561845011));
#212374=CARTESIAN_POINT('Ctrl Pts',(-28.8215510617709,-87.4323301854809,
73.4182942873751));
#212375=CARTESIAN_POINT('Ctrl Pts',(-28.9192184480609,-86.5851907514749,
77.5199574352398));
#212376=CARTESIAN_POINT('Ctrl Pts',(-29.0168858343509,-84.4248184280816,
81.1080038707725));
#212377=CARTESIAN_POINT('Ctrl Pts',(-29.1145532206409,-81.1961010250256,
83.7757125749618));
#212378=CARTESIAN_POINT('Ctrl Pts',(-29.2122206069309,-77.2650280175932,
85.2206869032595));
#212379=CARTESIAN_POINT('Ctrl Pts',(-29.3098879932209,-73.0772040121119,
85.2791325899756));
#212380=CARTESIAN_POINT('Ctrl Pts',(-29.4075553795109,-69.1073374822569,
83.9444245566035));
#212381=CARTESIAN_POINT('Ctrl Pts',(-29.5052227658009,-65.8054304526251,
81.3678578939925));
#212382=CARTESIAN_POINT('Ctrl Pts',(-29.6028901520909,-63.5457687681484,
77.8414978909712));
#212383=CARTESIAN_POINT('Ctrl Pts',(-29.7005575383809,-62.5844951291497,
73.7650731351128));
#212384=CARTESIAN_POINT('Ctrl Pts',(-29.7982249246709,-63.0305741772578,
69.6006644997806));
#212385=CARTESIAN_POINT('Ctrl Pts',(-29.8958923109609,-64.8334408687264,
65.8203262223269));
#212386=CARTESIAN_POINT('Ctrl Pts',(-29.9935596972509,-67.7887322469773,
62.8525764571267));
#212387=CARTESIAN_POINT('Ctrl Pts',(-30.0912270835409,-71.5614528925225,
61.0338228372305));
#212388=CARTESIAN_POINT('Ctrl Pts',(-30.1888944698309,-75.7239481434376,
60.570229173206));
#212389=CARTESIAN_POINT('Ctrl Pts',(-30.2865618561209,-79.8043806529974,
61.5143458683933));
#212390=CARTESIAN_POINT('Ctrl Pts',(-30.3842292424109,-83.3402152511359,
63.7591530970452));
#212391=CARTESIAN_POINT('Ctrl Pts',(-30.4818966287009,-85.930649362801,
67.0501919774507));
#212392=CARTESIAN_POINT('Ctrl Pts',(-30.5795640149909,-87.2820457621323,
71.0144086177314));
#212393=CARTESIAN_POINT('Ctrl Pts',(-30.6772314012809,-87.2412176577989,
75.2024414334004));
#212394=CARTESIAN_POINT('Ctrl Pts',(-30.7748987875709,-85.8127930969901,
79.1395582812056));
#212395=CARTESIAN_POINT('Ctrl Pts',(-30.8725661738609,-83.1586903556685,
82.3794694586463));
#212396=CARTESIAN_POINT('Ctrl Pts',(-30.9702335601509,-79.5797637819886,
84.5549166263378));
#212397=CARTESIAN_POINT('Ctrl Pts',(-31.0679009464409,-75.4817006180579,
85.4193031739153));
#212398=CARTESIAN_POINT('Ctrl Pts',(-31.1655683327309,-71.329034547002,
84.8746470423661));
#212399=CARTESIAN_POINT('Ctrl Pts',(-31.2632357190209,-67.5924887343543,
82.98268742638));
#212400=CARTESIAN_POINT('Ctrl Pts',(-31.3609031053109,-64.695617263651,
79.9578863610724));
#212401=CARTESIAN_POINT('Ctrl Pts',(-31.4585704916009,-62.9667933989244,
76.1431185004145));
#212402=CARTESIAN_POINT('Ctrl Pts',(-31.5562378778909,-62.6019870098559,
71.970804736377));
#212403=CARTESIAN_POINT('Ctrl Pts',(-31.6539052641809,-63.642550534956,
67.9138954205205));
#212404=CARTESIAN_POINT('Ctrl Pts',(-31.7515726504709,-65.9705314263782,
64.4322591422073));
#212405=CARTESIAN_POINT('Ctrl Pts',(-31.8492400367609,-69.3220428659327,
61.9205553116032));
#212406=CARTESIAN_POINT('Ctrl Pts',(-31.9469074230509,-73.3171755010594,
60.6634950264663));
#212407=CARTESIAN_POINT('Ctrl Pts',(-32.0445748093409,-77.5030656224803,
60.8035780069626));
#212408=CARTESIAN_POINT('Ctrl Pts',(-32.1422421956309,-81.4052152352389,
62.3249015374696));
#212409=CARTESIAN_POINT('Ctrl Pts',(-32.2399095819209,-84.5813309302388,
65.0551052312263));
#212410=CARTESIAN_POINT('Ctrl Pts',(-32.3050211727809,-85.974619775455,
67.4746207060263));
#212411=CARTESIAN_POINT('Ctrl Pts',(-32.3375769682109,-86.4508256027431,
68.7658628636918));
#212412=CARTESIAN_POINT('Ctrl Pts',(-26.3109923559309,-63.226796009855,
73.1405558201252));
#212413=CARTESIAN_POINT('Ctrl Pts',(-26.3435481513609,-63.2096934794613,
71.8129609505269));
#212414=CARTESIAN_POINT('Ctrl Pts',(-26.4086597422209,-63.6289072208686,
69.1522693813868));
#212415=CARTESIAN_POINT('Ctrl Pts',(-26.5063271285109,-65.5466883188414,
65.595862444819));
#212416=CARTESIAN_POINT('Ctrl Pts',(-26.6039945148009,-68.5360452568475,
62.8775596699701));
#212417=CARTESIAN_POINT('Ctrl Pts',(-26.7016619010909,-72.2581199618507,
61.3054018749864));
#212418=CARTESIAN_POINT('Ctrl Pts',(-26.7993292873809,-76.2909990282318,
61.0576244908063));
#212419=CARTESIAN_POINT('Ctrl Pts',(-26.8969966736709,-80.1775375961095,
62.1623076602056));
#212420=CARTESIAN_POINT('Ctrl Pts',(-26.9946640599609,-83.4771792584479,
64.4942323820704));
#212421=CARTESIAN_POINT('Ctrl Pts',(-27.0923314462509,-85.8158949537486,
67.789064150928));
#212422=CARTESIAN_POINT('Ctrl Pts',(-27.1899988325409,-86.9285808596196,
71.6733192596676));
#212423=CARTESIAN_POINT('Ctrl Pts',(-27.2876662188309,-86.6891090802536,
75.7067000853347));
#212424=CARTESIAN_POINT('Ctrl Pts',(-27.3853336051209,-85.1246248068445,
79.4320049844843));
#212425=CARTESIAN_POINT('Ctrl Pts',(-27.4830009914109,-82.4124692887962,
82.4269540784775));
#212426=CARTESIAN_POINT('Ctrl Pts',(-27.5806683777009,-78.860077414659,
84.3520565700369));
#212427=CARTESIAN_POINT('Ctrl Pts',(-27.6783357639909,-74.870128600351,
84.9890935309175));
#212428=CARTESIAN_POINT('Ctrl Pts',(-27.7760031502809,-70.8949012867121,
84.2658539888278));
#212429=CARTESIAN_POINT('Ctrl Pts',(-27.8736705365709,-67.3850051670203,
82.2643203620043));
#212430=CARTESIAN_POINT('Ctrl Pts',(-27.9713379228609,-64.7383025744529,
79.2113753875849));
#212431=CARTESIAN_POINT('Ctrl Pts',(-28.0690053091509,-63.254809017389,
75.453083954434));
#212432=CARTESIAN_POINT('Ctrl Pts',(-28.1666726954409,-63.1026850874199,
71.4154651090891));
#212433=CARTESIAN_POINT('Ctrl Pts',(-28.2643400817309,-64.2991747084623,
67.5562009023972));
#212434=CARTESIAN_POINT('Ctrl Pts',(-28.3620074680209,-66.7086504613652,
64.3127560937844));
#212435=CARTESIAN_POINT('Ctrl Pts',(-28.4596748543109,-70.0579875549346,
62.0527895754544));
#212436=CARTESIAN_POINT('Ctrl Pts',(-28.5573422406009,-73.9675237355834,
61.0324786020043));
#212437=CARTESIAN_POINT('Ctrl Pts',(-28.6550096268909,-77.994095692078,
61.367479959455));
#212438=CARTESIAN_POINT('Ctrl Pts',(-28.7526770131809,-81.6812735875568,
63.0198197542421));
#212439=CARTESIAN_POINT('Ctrl Pts',(-28.8503443994709,-84.6110994112092,
65.8021979228998));
#212440=CARTESIAN_POINT('Ctrl Pts',(-28.9480117857609,-86.4514643773875,
69.3992195271719));
#212441=CARTESIAN_POINT('Ctrl Pts',(-29.0456791720509,-86.99375493335,73.4031461727609));
#212442=CARTESIAN_POINT('Ctrl Pts',(-29.1433465583409,-86.176500033081,
77.3601149694952));
#212443=CARTESIAN_POINT('Ctrl Pts',(-29.2410139446309,-84.0923391537426,
80.8215859081834));
#212444=CARTESIAN_POINT('Ctrl Pts',(-29.3386813309209,-80.9775211989782,
83.3951858652538));
#212445=CARTESIAN_POINT('Ctrl Pts',(-29.4363487172109,-77.1851246351153,
84.789185841132));
#212446=CARTESIAN_POINT('Ctrl Pts',(-29.5340161035009,-73.1450344769205,
84.8455697396331));
#212447=CARTESIAN_POINT('Ctrl Pts',(-29.6316834897909,-69.3152129095361,
83.5579461951267));
#212448=CARTESIAN_POINT('Ctrl Pts',(-29.7293508760809,-66.1297872383019,
81.0722730622718));
#212449=CARTESIAN_POINT('Ctrl Pts',(-29.8270182623709,-63.9498396281978,
77.6703124441067));
#212450=CARTESIAN_POINT('Ctrl Pts',(-29.9246856486609,-63.0224768347345,
73.7376917047466));
#212451=CARTESIAN_POINT('Ctrl Pts',(-30.0223530349509,-63.4528195544114,
69.7201908928029));
#212452=CARTESIAN_POINT('Ctrl Pts',(-30.1200204212409,-65.1920865262802,
66.0732115905697));
#212453=CARTESIAN_POINT('Ctrl Pts',(-30.2176878075309,-68.0431241048049,
63.2101551195605));
#212454=CARTESIAN_POINT('Ctrl Pts',(-30.3153551938209,-71.6827545022938,
61.4555616623674));
#212455=CARTESIAN_POINT('Ctrl Pts',(-30.4130225801109,-75.6984094282703,
61.0083221897941));
#212456=CARTESIAN_POINT('Ctrl Pts',(-30.5106899664009,-79.634896539825,
61.9191332848712));
#212457=CARTESIAN_POINT('Ctrl Pts',(-30.6083573526909,-83.0459975178568,
64.0847504597221));
#212458=CARTESIAN_POINT('Ctrl Pts',(-30.7060247389809,-85.5450488978255,
67.2596913773822));
#212459=CARTESIAN_POINT('Ctrl Pts',(-30.8036921252709,-86.8487720928805,
71.0840623663197));
#212460=CARTESIAN_POINT('Ctrl Pts',(-30.9013595115609,-86.8093842813913,
75.1243539684997));
#212461=CARTESIAN_POINT('Ctrl Pts',(-30.9990268978509,-85.4313502469366,
78.9225811642113));
#212462=CARTESIAN_POINT('Ctrl Pts',(-31.0966942841409,-82.8708762752482,
82.0481980106353));
#212463=CARTESIAN_POINT('Ctrl Pts',(-31.1943616704309,-79.4182034770832,
84.1469019390542));
#212464=CARTESIAN_POINT('Ctrl Pts',(-31.2920290567209,-75.4647076676689,
84.980795526557));
#212465=CARTESIAN_POINT('Ctrl Pts',(-31.3896964430109,-71.4585351776186,
84.4553532267351));
#212466=CARTESIAN_POINT('Ctrl Pts',(-31.4873638293009,-67.8538034736301,
82.630136261015));
#212467=CARTESIAN_POINT('Ctrl Pts',(-31.5850312155909,-65.0591249238588,
79.712041088333));
#212468=CARTESIAN_POINT('Ctrl Pts',(-31.6826986018809,-63.3912887702861,
76.0318467751409));
#212469=CARTESIAN_POINT('Ctrl Pts',(-31.7803659881709,-63.0393516544576,
72.0067197036773));
#212470=CARTESIAN_POINT('Ctrl Pts',(-31.8780333744609,-64.0432072250835,
68.0929259582372));
#212471=CARTESIAN_POINT('Ctrl Pts',(-31.9757007607509,-66.2890639457993,
64.7341113461543));
#212472=CARTESIAN_POINT('Ctrl Pts',(-32.0733681470409,-69.5223441324314,
62.3110128795057));
#212473=CARTESIAN_POINT('Ctrl Pts',(-32.1710355333309,-73.3765404928114,
61.0982979039962));
#212474=CARTESIAN_POINT('Ctrl Pts',(-32.2687029196209,-77.4147649885621,
61.233439177867));
#212475=CARTESIAN_POINT('Ctrl Pts',(-32.3663703059109,-81.1792584882072,
62.7010949855073));
#212476=CARTESIAN_POINT('Ctrl Pts',(-32.4640376922009,-84.2433303651157,
65.3349852966984));
#212477=CARTESIAN_POINT('Ctrl Pts',(-32.5291492830609,-85.5874681664406,
67.6691475357372));
#212478=CARTESIAN_POINT('Ctrl Pts',(-32.5617050784909,-86.0468748830494,
68.9148385500206));
#212479=CARTESIAN_POINT('',(-25.7929823067402,-63.0439337595017,67.8848523453354));
#212480=CARTESIAN_POINT('Ctrl Pts',(-21.8528274563309,-63.9256801348964,
79.922508163981));
#212481=CARTESIAN_POINT('Ctrl Pts',(-21.8943126079409,-62.9293684428046,
78.331207182819));
#212482=CARTESIAN_POINT('Ctrl Pts',(-21.9772829111709,-61.634085238876,
74.7135063587071));
#212483=CARTESIAN_POINT('Ctrl Pts',(-22.1017383660109,-62.1361793310051,
68.9705612798485));
#212484=CARTESIAN_POINT('Ctrl Pts',(-22.2261938208509,-64.992093640751,
63.9630709697879));
#212485=CARTESIAN_POINT('Ctrl Pts',(-22.3506492756909,-69.6791054908813,
60.6069640495695));
#212486=CARTESIAN_POINT('Ctrl Pts',(-22.4751047305309,-75.339685598698,
59.516380349804));
#212487=CARTESIAN_POINT('Ctrl Pts',(-22.5995601853709,-80.9381110935543,
60.8908421950948));
#212488=CARTESIAN_POINT('Ctrl Pts',(-22.7240156402109,-85.4500477813155,
64.47887134835));
#212489=CARTESIAN_POINT('Ctrl Pts',(-22.8484710950509,-88.049950735903,
69.6239686585276));
#212490=CARTESIAN_POINT('Ctrl Pts',(-22.9729265498909,-88.262118873329,
75.3847418289771));
#212491=CARTESIAN_POINT('Ctrl Pts',(-23.0973820047309,-86.0477319607849,
80.7071485391445));
#212492=CARTESIAN_POINT('Ctrl Pts',(-23.2218374595709,-81.8119539092029,
84.6173540230353));
#212493=CARTESIAN_POINT('Ctrl Pts',(-23.3462929144109,-76.3298002796115,
86.3999123553094));
#212494=CARTESIAN_POINT('Ctrl Pts',(-23.4707483692509,-70.6043345825818,
85.7286708365146));
#212495=CARTESIAN_POINT('Ctrl Pts',(-23.5952038240909,-65.6831388635119,
82.726445774969));
#212496=CARTESIAN_POINT('Ctrl Pts',(-23.7196592789309,-62.4666387912098,
77.9425509276692));
#212497=CARTESIAN_POINT('Ctrl Pts',(-23.8441147337709,-61.5433537812183,
72.2522901765632));
#212498=CARTESIAN_POINT('Ctrl Pts',(-23.9685701886109,-63.0822162576926,
66.6968041578817));
#212499=CARTESIAN_POINT('Ctrl Pts',(-24.0930256434509,-66.8016622769115,
62.2925739260189));
#212500=CARTESIAN_POINT('Ctrl Pts',(-24.2174810982909,-72.0211489667569,
59.8454365534837));
#212501=CARTESIAN_POINT('Ctrl Pts',(-24.3419365531309,-77.785672693591,
59.8031420245331));
#212502=CARTESIAN_POINT('Ctrl Pts',(-24.4663920079709,-83.0405050080979,
62.1734289212542));
#212503=CARTESIAN_POINT('Ctrl Pts',(-24.5908474628109,-86.824175125915,
66.5226085068829));
#212504=CARTESIAN_POINT('Ctrl Pts',(-24.7153029176509,-88.4443891690571,
72.0549162569263));
#212505=CARTESIAN_POINT('Ctrl Pts',(-24.8397583724909,-87.6046983680189,
77.7581120451255));
#212506=CARTESIAN_POINT('Ctrl Pts',(-24.9642138273309,-84.4587400856684,
82.588688427932));
#212507=CARTESIAN_POINT('Ctrl Pts',(-25.0886692821709,-79.582126496041,
85.6628006211223));
#212508=CARTESIAN_POINT('Ctrl Pts',(-25.2131247370109,-73.8671272050187,
86.4179803938817));
#212509=CARTESIAN_POINT('Ctrl Pts',(-25.3375801918409,-68.3594052031391,
84.7160584470277));
#212510=CARTESIAN_POINT('Ctrl Pts',(-25.4620356466809,-64.0667172511486,
80.8684145069103));
#212511=CARTESIAN_POINT('Ctrl Pts',(-25.5864911015209,-61.7744355441518,
75.5791186817847));
#212512=CARTESIAN_POINT('Ctrl Pts',(-25.7109465563609,-61.9021857092216,
69.8156825060804));
#212513=CARTESIAN_POINT('Ctrl Pts',(-25.7939168595909,-63.5846031768828,
66.3609771213051));
#212514=CARTESIAN_POINT('Ctrl Pts',(-25.8354020112009,-64.7486531924386,
64.8879315138231));
#212515=CARTESIAN_POINT('Ctrl Pts',(-22.0769555666009,-64.2906021585369,
79.6940309097319));
#212516=CARTESIAN_POINT('Ctrl Pts',(-22.1184407182209,-63.327121022488,
78.155166627284));
#212517=CARTESIAN_POINT('Ctrl Pts',(-22.2014110214409,-62.0745201118013,
74.6566766189857));
#212518=CARTESIAN_POINT('Ctrl Pts',(-22.3258664762809,-62.5600691524593,
69.1029736033338));
#212519=CARTESIAN_POINT('Ctrl Pts',(-22.4503219311209,-65.3218751068457,
64.2604905821706));
#212520=CARTESIAN_POINT('Ctrl Pts',(-22.5747773859609,-69.8544401042544,
61.0149744109849));
#212521=CARTESIAN_POINT('Ctrl Pts',(-22.6992328408009,-75.3284922470942,
59.9603277272687));
#212522=CARTESIAN_POINT('Ctrl Pts',(-22.8236882956409,-80.7424379015931,
61.2894981773207));
#212523=CARTESIAN_POINT('Ctrl Pts',(-22.9481437504809,-85.1056968297407,
64.7592942584412));
#212524=CARTESIAN_POINT('Ctrl Pts',(-23.0725992053209,-87.6199275390778,
69.7348498409864));
#212525=CARTESIAN_POINT('Ctrl Pts',(-23.1970546601609,-87.8251042921967,
75.3057934752901));
#212526=CARTESIAN_POINT('Ctrl Pts',(-23.3215101150009,-85.6836860642405,
80.452815741888));
#212527=CARTESIAN_POINT('Ctrl Pts',(-23.4459655698409,-81.5874857670595,
84.2341717690691));
#212528=CARTESIAN_POINT('Ctrl Pts',(-23.5704210246809,-76.2859805764563,
85.9579910725117));
#212529=CARTESIAN_POINT('Ctrl Pts',(-23.6948764795209,-70.7491809604065,
85.3088683670014));
#212530=CARTESIAN_POINT('Ctrl Pts',(-23.8193319343609,-65.9901489428121,
82.4055729063876));
#212531=CARTESIAN_POINT('Ctrl Pts',(-23.9437873892009,-62.8796392816311,
77.7793174093933));
#212532=CARTESIAN_POINT('Ctrl Pts',(-24.0682428440409,-61.9867784456194,
72.2765626625984));
#212533=CARTESIAN_POINT('Ctrl Pts',(-24.1926982988809,-63.4749321818895,
66.9041415386483));
#212534=CARTESIAN_POINT('Ctrl Pts',(-24.3171537537209,-67.0718146681149,
62.6450399131801));
#212535=CARTESIAN_POINT('Ctrl Pts',(-24.4416092085609,-72.1193083445342,
60.278540840157));
#212536=CARTESIAN_POINT('Ctrl Pts',(-24.5660646634009,-77.6938789465367,
60.2376400044813));
#212537=CARTESIAN_POINT('Ctrl Pts',(-24.6905201182409,-82.7755535352872,
62.5298209857594));
#212538=CARTESIAN_POINT('Ctrl Pts',(-24.8149755730809,-86.434543801599,
66.7356859990377));
#212539=CARTESIAN_POINT('Ctrl Pts',(-24.9394310279209,-88.0013684001015,
72.0856926268273));
#212540=CARTESIAN_POINT('Ctrl Pts',(-25.0638864827609,-87.1893471688506,
77.6009561741625));
#212541=CARTESIAN_POINT('Ctrl Pts',(-25.1883419376009,-84.1470547979677,
82.2723549523412));
#212542=CARTESIAN_POINT('Ctrl Pts',(-25.3127973924409,-79.4311358353121,
85.2451687131141));
#212543=CARTESIAN_POINT('Ctrl Pts',(-25.4372528472809,-73.9044577352793,
85.9754637313838));
#212544=CARTESIAN_POINT('Ctrl Pts',(-25.5617083021209,-68.5782267037815,
84.3296236756515));
#212545=CARTESIAN_POINT('Ctrl Pts',(-25.6861637569609,-64.4269918065508,
80.6087676584068));
#212546=CARTESIAN_POINT('Ctrl Pts',(-25.8106192118009,-62.2102455806975,
75.4937652038599));
#212547=CARTESIAN_POINT('Ctrl Pts',(-25.9350746666409,-62.3337861103748,
69.9202463159047));
#212548=CARTESIAN_POINT('Ctrl Pts',(-26.0180449698709,-63.9607644003393,
66.5793807059784));
#212549=CARTESIAN_POINT('Ctrl Pts',(-26.0595301214809,-65.0864565309473,
65.1548750350942));
#212550=CARTESIAN_POINT('Ctrl Pts',(-22.3010836768809,-64.6555241821984,
79.4655536555077));
#212551=CARTESIAN_POINT('Ctrl Pts',(-22.3425688284909,-63.7248736021842,
77.9791260717798));
#212552=CARTESIAN_POINT('Ctrl Pts',(-22.4255391317209,-62.5149549847303,
74.5998468792995));
#212553=CARTESIAN_POINT('Ctrl Pts',(-22.5499945865609,-62.9839589739056,
69.2353859268549));
#212554=CARTESIAN_POINT('Ctrl Pts',(-22.6744500414009,-65.6516565729139,
64.557910194586));
#212555=CARTESIAN_POINT('Ctrl Pts',(-22.7989054962409,-70.0297747175908,
61.4229847724263));
#212556=CARTESIAN_POINT('Ctrl Pts',(-22.9233609510809,-75.3172988954431,
60.4042751047314));
#212557=CARTESIAN_POINT('Ctrl Pts',(-23.0478164059209,-80.5467647095836,
61.6881541595265));
#212558=CARTESIAN_POINT('Ctrl Pts',(-23.1722718607609,-84.761345878138,
65.0397171684909));
#212559=CARTESIAN_POINT('Ctrl Pts',(-23.2967273156009,-87.1899043422416,
69.8457310233925));
#212560=CARTESIAN_POINT('Ctrl Pts',(-23.4211827704409,-87.3880897110839,
75.2268451215454));
#212561=CARTESIAN_POINT('Ctrl Pts',(-23.5456382252809,-85.3196401677329,
80.1984829445947));
#212562=CARTESIAN_POINT('Ctrl Pts',(-23.6700936801209,-81.3630176249706,
83.8509895150804));
#212563=CARTESIAN_POINT('Ctrl Pts',(-23.7945491349609,-76.2421608733568,
85.5160697897019));
#212564=CARTESIAN_POINT('Ctrl Pts',(-23.9190045898009,-70.8940273382887,
84.8890658975066));
#212565=CARTESIAN_POINT('Ctrl Pts',(-24.0434600446409,-66.2971590221518,
82.0847000378495));
#212566=CARTESIAN_POINT('Ctrl Pts',(-24.1679154994809,-63.2926397720848,
77.6160838911696));
#212567=CARTESIAN_POINT('Ctrl Pts',(-24.2923709543209,-62.4302031100231,
72.3008351486921));
#212568=CARTESIAN_POINT('Ctrl Pts',(-24.4168264091609,-63.8676481060571,
67.1114789194617));
#212569=CARTESIAN_POINT('Ctrl Pts',(-24.5412818640009,-67.3419670592723,
62.9975059003819));
#212570=CARTESIAN_POINT('Ctrl Pts',(-24.6657373188409,-72.2174677222541,
60.7116451268433));
#212571=CARTESIAN_POINT('Ctrl Pts',(-24.7901927736809,-77.6020851994283,
60.6721379844194));
#212572=CARTESIAN_POINT('Ctrl Pts',(-24.9146482285209,-82.5106020624308,
62.8862130502326));
#212573=CARTESIAN_POINT('Ctrl Pts',(-25.0391036833609,-86.044912477272,
66.9487634911396));
#212574=CARTESIAN_POINT('Ctrl Pts',(-25.1635591382009,-87.5583476311469,
72.1164689966782));
#212575=CARTESIAN_POINT('Ctrl Pts',(-25.2880145930409,-86.7739959696993,
77.4438003031567));
#212576=CARTESIAN_POINT('Ctrl Pts',(-25.4124700478809,-83.8353695102982,
81.9560214767265));
#212577=CARTESIAN_POINT('Ctrl Pts',(-25.5369255027209,-79.2801451746127,
84.8275368050828));
#212578=CARTESIAN_POINT('Ctrl Pts',(-25.6613809575609,-73.9417882655686,
85.5329470688847));
#212579=CARTESIAN_POINT('Ctrl Pts',(-25.7858364124009,-68.7970482044449,
83.9431889042894));
#212580=CARTESIAN_POINT('Ctrl Pts',(-25.9102918672409,-64.7872663619598,
80.3491208099199));
#212581=CARTESIAN_POINT('Ctrl Pts',(-26.0347473220809,-62.6460556172474,
75.4084117259451));
#212582=CARTESIAN_POINT('Ctrl Pts',(-26.1592027769209,-62.7653865115381,
70.024810125727));
#212583=CARTESIAN_POINT('Ctrl Pts',(-26.2421730801409,-64.3369256238002,
66.7977842906575));
#212584=CARTESIAN_POINT('Ctrl Pts',(-26.2836582317609,-65.4242598694568,
65.4218185563542));
#212585=CARTESIAN_POINT('Ctrl Pts',(-22.5252117871509,-65.0204462058481,
79.2370764012548));
#212586=CARTESIAN_POINT('Ctrl Pts',(-22.5666969387709,-64.1226261818582,
77.8030855162482));
#212587=CARTESIAN_POINT('Ctrl Pts',(-22.6496672419909,-62.9553898576556,
74.5430171395781));
#212588=CARTESIAN_POINT('Ctrl Pts',(-22.7741226968309,-63.4078487953635,
69.3677982503388));
#212589=CARTESIAN_POINT('Ctrl Pts',(-22.8985781516709,-65.9814380390095,
64.8553298069684));
#212590=CARTESIAN_POINT('Ctrl Pts',(-23.0230336065109,-70.2051093309645,
61.8309951338414));
#212591=CARTESIAN_POINT('Ctrl Pts',(-23.1474890613509,-75.3061055438402,
60.8482224821958));
#212592=CARTESIAN_POINT('Ctrl Pts',(-23.2719445161909,-80.3510915176178,
62.0868101417542));
#212593=CARTESIAN_POINT('Ctrl Pts',(-23.3963999710309,-84.4169949265728,
65.3201400785791));
#212594=CARTESIAN_POINT('Ctrl Pts',(-23.5208554258709,-86.7598811454164,
69.9566122058513));
#212595=CARTESIAN_POINT('Ctrl Pts',(-23.6453108807209,-86.9510751299516,
75.1478967678584));
#212596=CARTESIAN_POINT('Ctrl Pts',(-23.7697663355609,-84.9555942711914,
79.9441501473478));
#212597=CARTESIAN_POINT('Ctrl Pts',(-23.8942217904009,-81.1385494828272,
83.4678072611142));
#212598=CARTESIAN_POINT('Ctrl Pts',(-24.0186772452409,-76.1983411702007,
85.0741485069047));
#212599=CARTESIAN_POINT('Ctrl Pts',(-24.1431327000809,-71.0388737161131,
84.4692634279924));
#212600=CARTESIAN_POINT('Ctrl Pts',(-24.2675881549209,-66.6041691014425,
81.7638271692711));
#212601=CARTESIAN_POINT('Ctrl Pts',(-24.3920436097609,-63.7056402625057,
77.4528503728929));
#212602=CARTESIAN_POINT('Ctrl Pts',(-24.5164990646009,-62.8736277744238,
72.3251076347263));
#212603=CARTESIAN_POINT('Ctrl Pts',(-24.6409545194409,-64.260364030253,
67.3188163002233));
#212604=CARTESIAN_POINT('Ctrl Pts',(-24.7654099742709,-67.6121194504766,
63.3499718875427));
#212605=CARTESIAN_POINT('Ctrl Pts',(-24.8898654291109,-72.3156271000323,
61.1447494135163));
#212606=CARTESIAN_POINT('Ctrl Pts',(-25.0143208839509,-77.5102914523739,
61.1066359643676));
#212607=CARTESIAN_POINT('Ctrl Pts',(-25.1387763387909,-82.2456505896205,
63.2426051147388));
#212608=CARTESIAN_POINT('Ctrl Pts',(-25.2632317936309,-85.655281152956,
67.1618409832944));
#212609=CARTESIAN_POINT('Ctrl Pts',(-25.3876872484709,-87.1153268621918,
72.1472453665801));
#212610=CARTESIAN_POINT('Ctrl Pts',(-25.5121427033109,-86.3586447705307,
77.2866444321927));
#212611=CARTESIAN_POINT('Ctrl Pts',(-25.6365981581509,-83.5236842225936,
81.6396880011264));
#212612=CARTESIAN_POINT('Ctrl Pts',(-25.7610536129909,-79.1291545138833,
84.4099048970747));
#212613=CARTESIAN_POINT('Ctrl Pts',(-25.8855090678309,-73.9791187958291,
85.0904304063868));
#212614=CARTESIAN_POINT('Ctrl Pts',(-26.0099645226709,-69.0158697050855,
83.556754132914));
#212615=CARTESIAN_POINT('Ctrl Pts',(-26.1344199775109,-65.1475409173708,
80.0894739614117));
#212616=CARTESIAN_POINT('Ctrl Pts',(-26.2588754323509,-63.0818656537839,
75.3230582480241));
#212617=CARTESIAN_POINT('Ctrl Pts',(-26.3833308871909,-63.1969869126954,
70.1293739355506));
#212618=CARTESIAN_POINT('Ctrl Pts',(-26.4663011904209,-64.7130868472582,
67.0161878753345));
#212619=CARTESIAN_POINT('Ctrl Pts',(-26.5077863420309,-65.7620632079617,
65.688762077616));
#212620=CARTESIAN_POINT('',(-22.5675364832709,-63.0005606563318,73.0560055650936));
#212621=CARTESIAN_POINT('Ctrl Pts',(-22.5675364832709,-63.0009379796994,
73.0559939530083));
#212622=CARTESIAN_POINT('Ctrl Pts',(-22.5675364832709,-63.030239404122,
73.6283224514651));
#212623=CARTESIAN_POINT('Ctrl Pts',(-22.5675364832698,-63.1004752890019,
74.1992222599949));
#212624=CARTESIAN_POINT('Ctrl Pts',(-22.5675364832698,-63.3236284085513,
75.3219313585469));
#212625=CARTESIAN_POINT('Ctrl Pts',(-22.5675364832709,-63.4751104430327,
75.8722213989227));
#212626=CARTESIAN_POINT('Ctrl Pts',(-22.5675364832709,-63.6650775896172,
76.4088722773802));
#212627=CARTESIAN_POINT('Ctrl Pts',(-22.5673477912806,-63.0003719673623,
73.0560066204831));
#212628=CARTESIAN_POINT('Ctrl Pts',(-22.5674106883502,-63.000278188672,
73.0504855961934));
#212629=CARTESIAN_POINT('Ctrl Pts',(-22.5674735854198,-63.0001882203141,
73.0449644637677));
#212630=CARTESIAN_POINT('Ctrl Pts',(-22.5675364824894,-63.000102062494,
73.0394432284656));
#212631=CARTESIAN_POINT('Origin',(-21.7675364832709,-75.,72.98888938658));
#212632=CARTESIAN_POINT('',(-23.0675424572509,-65.2956417762688,76.9983072327892));
#212633=CARTESIAN_POINT('',(-23.0675424572509,-84.7043582237312,68.9794715403708));
#212634=CARTESIAN_POINT('Origin',(-23.0675424572509,-75.,72.98888938658));
#212635=CARTESIAN_POINT('',(-38.5675364832709,-65.2956417762688,76.9983072327892));
#212636=CARTESIAN_POINT('',(-21.7675364832709,-65.2956417762688,76.9983072327892));
#212637=CARTESIAN_POINT('Origin',(-38.5675364832709,-75.,72.98888938658));
#212638=CARTESIAN_POINT('Origin',(-23.0675424572509,-75.,72.98888938658));
#212639=CARTESIAN_POINT('Origin',(-22.8175393993109,-75.,72.98888938658));
#212640=CARTESIAN_POINT('',(-22.5675364832709,-85.1664763034716,68.7885444915901));
#212641=CARTESIAN_POINT('',(-22.8175393993109,-84.9354173291752,68.8840079888882));
#212642=CARTESIAN_POINT('Origin',(-22.5675364832709,-75.,72.98888938658));
#212643=CARTESIAN_POINT('Origin',(-22.5675364832709,-75.,72.98888938658));
#212644=CARTESIAN_POINT('Origin',(-38.5675364832709,-75.,72.98888938658));
#212645=CARTESIAN_POINT('Origin',(-48.5675364832709,-83.3180213346267,69.5522455184007));
#212646=CARTESIAN_POINT('',(-48.5675364832709,-76.1552807409203,72.5115777382218));
#212647=CARTESIAN_POINT('Origin',(-48.5675364832709,-83.3180213346267,69.5522455184007));
#212648=CARTESIAN_POINT('Origin',(-47.7675364832709,-83.3180213346267,69.5522455184007));
#212649=CARTESIAN_POINT('',(-64.0675410045048,-76.1552807409203,72.5115777382218));
#212650=CARTESIAN_POINT('',(-47.7675364832709,-76.1552807409204,72.5115777382218));
#212651=CARTESIAN_POINT('Origin',(-64.0675410045048,-83.3180213346267,69.5522455184007));
#212652=CARTESIAN_POINT('Origin',(-64.3175392245649,-83.3180213346267,69.5522455184006));
#212653=CARTESIAN_POINT('',(-64.5675367041794,-75.6931730807022,72.7025004821099));
#212654=CARTESIAN_POINT('',(-64.3175392245649,-75.924226752407,72.6070391756115));
#212655=CARTESIAN_POINT('Origin',(-64.5675367039552,-83.3180213346267,69.5522455184007));
#212656=CARTESIAN_POINT('Origin',(-64.5675364832709,-83.3180213346267,69.5522455184007));
#212657=CARTESIAN_POINT('Ctrl Pts',(-64.5675364832709,-92.3390416319356,
70.6705889999386));
#212658=CARTESIAN_POINT('Ctrl Pts',(-64.5675364832709,-92.3115488079351,
71.1096763190362));
#212659=CARTESIAN_POINT('Ctrl Pts',(-64.5675364832708,-92.2516905128383,
71.5466701563317));
#212660=CARTESIAN_POINT('Ctrl Pts',(-64.5675364832708,-92.0696201922871,
72.4106673105199));
#212661=CARTESIAN_POINT('Ctrl Pts',(-64.5675364832709,-91.9469758966146,
72.8375946044303));
#212662=CARTESIAN_POINT('Ctrl Pts',(-64.5675364832709,-91.7945388584896,
73.25356812809));
#212663=CARTESIAN_POINT('Origin',(-45.8894114130409,-83.3180213346267,69.5522455184007));
#212664=CARTESIAN_POINT('',(-63.5674079539854,-86.5607427128165,59.8285649416409));
#212665=CARTESIAN_POINT('Ctrl Pts',(-63.567539947994,-86.5649230506972,
59.8300991896837));
#212666=CARTESIAN_POINT('Ctrl Pts',(-63.5674959499171,-86.5635297248365,
59.829587474225));
#212667=CARTESIAN_POINT('Ctrl Pts',(-63.5674519518401,-86.5621362788099,
59.8290760582622));
#212668=CARTESIAN_POINT('Ctrl Pts',(-63.5674079537632,-86.5607427127462,
59.8285649418516));
#212669=CARTESIAN_POINT('',(-62.9075072593131,-73.8447139480805,73.4661881802199));
#212670=CARTESIAN_POINT('Ctrl Pts',(-63.5674123768639,-86.5606760704595,
59.8286818576752));
#212671=CARTESIAN_POINT('Ctrl Pts',(-63.5537244696136,-86.1049641428571,
59.6767091353507));
#212672=CARTESIAN_POINT('Ctrl Pts',(-63.5400136073417,-85.6391282969738,
59.5569597714857));
#212673=CARTESIAN_POINT('Ctrl Pts',(-63.5129296748257,-84.6949018026879,
59.3838289856031));
#212674=CARTESIAN_POINT('Ctrl Pts',(-63.4995889539748,-84.2176985104596,
59.330549021255));
#212675=CARTESIAN_POINT('Ctrl Pts',(-63.4597780386861,-82.7876084763752,
59.2718310830067));
#212676=CARTESIAN_POINT('Ctrl Pts',(-63.4325802602361,-81.8358809821594,
59.3654163782555));
#212677=CARTESIAN_POINT('Ctrl Pts',(-63.3869424607677,-80.2668114174402,
59.744516418622));
#212678=CARTESIAN_POINT('Ctrl Pts',(-63.3686283032081,-79.6394241802636,
59.9621800299818));
#212679=CARTESIAN_POINT('Ctrl Pts',(-63.3128692356677,-77.8226955709727,
60.7971770385973));
#212680=CARTESIAN_POINT('Ctrl Pts',(-63.2745815754463,-76.7288390210066,
61.5877935685209));
#212681=CARTESIAN_POINT('Ctrl Pts',(-63.2002097006855,-74.9063461491549,
63.5444294238348));
#212682=CARTESIAN_POINT('Ctrl Pts',(-63.1618824850836,-74.1952322716333,
64.6917037744084));
#212683=CARTESIAN_POINT('Ctrl Pts',(-63.1061663303517,-73.4911387374014,
66.563278327776));
#212684=CARTESIAN_POINT('Ctrl Pts',(-63.0878060649446,-73.3185146829425,
67.2046067609665));
#212685=CARTESIAN_POINT('Ctrl Pts',(-63.0553782680594,-73.1303627086226,
68.3273127282598));
#212686=CARTESIAN_POINT('Ctrl Pts',(-63.0417928519769,-73.0844909277082,
68.8014397964857));
#212687=CARTESIAN_POINT('Ctrl Pts',(-63.0081560309446,-73.0525026114093,
69.9923893239146));
#212688=CARTESIAN_POINT('Ctrl Pts',(-62.9884692522367,-73.1082554644126,
70.7077860596406));
#212689=CARTESIAN_POINT('Ctrl Pts',(-62.9483777816462,-73.3679537925859,
72.1157259528594));
#212690=CARTESIAN_POINT('Ctrl Pts',(-62.9277656193976,-73.5712828969068,
72.8043756242868));
#212691=CARTESIAN_POINT('Ctrl Pts',(-62.9075072593131,-73.8447139480805,
73.46618818022));
#212692=CARTESIAN_POINT('Ctrl Pts',(-62.9075072593131,-73.8447139480805,
73.4661881802199));
#212693=CARTESIAN_POINT('Ctrl Pts',(-62.9075071281503,-73.8447157184106,
73.4661924651272));
#212694=CARTESIAN_POINT('Ctrl Pts',(-62.9075069969875,-73.8447174887436,
73.4661967500333));
#212695=CARTESIAN_POINT('Ctrl Pts',(-62.9075068658247,-73.8447192590795,
73.4662010349381));
#212696=CARTESIAN_POINT('Ctrl Pts',(-64.7235137149846,-91.0358871866423,
74.2288240611484));
#212697=CARTESIAN_POINT('Ctrl Pts',(-64.6818903153503,-91.7101176437746,
73.1161259264027));
#212698=CARTESIAN_POINT('Ctrl Pts',(-64.5986435160818,-92.5693071181569,
70.5953071644979));
#212699=CARTESIAN_POINT('Ctrl Pts',(-64.4737733171789,-92.1546318852882,
66.6213799744605));
#212700=CARTESIAN_POINT('Ctrl Pts',(-64.3489031182761,-90.1124097711939,
63.1873940424806));
#212701=CARTESIAN_POINT('Ctrl Pts',(-64.2240329193733,-86.8188823631399,
60.9255881378498));
#212702=CARTESIAN_POINT('Ctrl Pts',(-64.0991627204705,-82.8805899113611,
60.2525763176751));
#212703=CARTESIAN_POINT('Ctrl Pts',(-63.9742925215677,-79.0228616330947,
61.2922934738363));
#212704=CARTESIAN_POINT('Ctrl Pts',(-63.8494223226649,-75.9561779481362,
63.8532574547353));
#212705=CARTESIAN_POINT('Ctrl Pts',(-63.7245521237622,-74.2453345756984,
67.4638112038692));
#212706=CARTESIAN_POINT('Ctrl Pts',(-63.5996819248594,-74.2054195650181,
71.4589945804266));
#212707=CARTESIAN_POINT('Ctrl Pts',(-63.4748117259569,-75.8437841906902,
75.1030097681569));
#212708=CARTESIAN_POINT('Ctrl Pts',(-63.3499415270539,-78.8586886049028,
77.7247325999806));
#212709=CARTESIAN_POINT('Ctrl Pts',(-63.2250713281509,-82.694874402881,
78.8413215436999));
#212710=CARTESIAN_POINT('Ctrl Pts',(-63.1002011292489,-86.6458247360063,
78.2471160211358));
#212711=CARTESIAN_POINT('Ctrl Pts',(-62.9753309303459,-89.9838938499185,
76.0516149086199));
#212712=CARTESIAN_POINT('Ctrl Pts',(-62.8504607314429,-92.0942834014676,
72.6589303077136));
#212713=CARTESIAN_POINT('Ctrl Pts',(-62.7672139321749,-92.4236956643394,
70.0161625645472));
#212714=CARTESIAN_POINT('Ctrl Pts',(-62.7255905325409,-92.3038054643285,
68.72066644786));
#212715=CARTESIAN_POINT('Ctrl Pts',(-64.4993856047086,-91.4041086405805,
74.4519448802345));
#212716=CARTESIAN_POINT('Ctrl Pts',(-64.4577622050742,-92.1105068140245,
73.2861596184454));
#212717=CARTESIAN_POINT('Ctrl Pts',(-64.3745154058057,-93.0106884491278,
70.6450719159536));
#212718=CARTESIAN_POINT('Ctrl Pts',(-64.2496452069029,-92.5762289494608,
66.4815475917031));
#212719=CARTESIAN_POINT('Ctrl Pts',(-64.1247750080001,-90.4365718694728,
62.8837252680371));
#212720=CARTESIAN_POINT('Ctrl Pts',(-63.9999048090973,-86.9859093836459,
60.5140079958518));
#212721=CARTESIAN_POINT('Ctrl Pts',(-63.8750346101945,-82.8597199405946,
59.8088866008653));
#212722=CARTESIAN_POINT('Ctrl Pts',(-63.7501644112917,-78.8179384094302,
60.8982089419637));
#212723=CARTESIAN_POINT('Ctrl Pts',(-63.6252942123889,-75.604942421705,
63.5813572026399));
#212724=CARTESIAN_POINT('Ctrl Pts',(-63.5004240134859,-73.8124742521855,
67.3641714414642));
#212725=CARTESIAN_POINT('Ctrl Pts',(-63.3755538145829,-73.7706548856186,
71.5499660906055));
#212726=CARTESIAN_POINT('Ctrl Pts',(-63.2506836156809,-75.4871863278845,
75.3678382222557));
#212727=CARTESIAN_POINT('Ctrl Pts',(-63.1258134167779,-78.6459326419415,
78.1146441549624));
#212728=CARTESIAN_POINT('Ctrl Pts',(-63.0009432178749,-82.6651438952985,
79.2845058572658));
#212729=CARTESIAN_POINT('Ctrl Pts',(-62.8760730189729,-86.8045951306179,
78.6619506295288));
#212730=CARTESIAN_POINT('Ctrl Pts',(-62.7512028200699,-90.3019244190495,
76.3617015689027));
#212731=CARTESIAN_POINT('Ctrl Pts',(-62.6263326211669,-92.5130012232632,
72.8071510739181));
#212732=CARTESIAN_POINT('Ctrl Pts',(-62.5430858218989,-92.8581298337256,
70.0382961714913));
#212733=CARTESIAN_POINT('Ctrl Pts',(-62.5014624222649,-92.7325196400449,
68.6809915869217));
#212734=CARTESIAN_POINT('Ctrl Pts',(-64.2752574944325,-91.7723300945254,
74.6750656993104));
#212735=CARTESIAN_POINT('Ctrl Pts',(-64.2336340947982,-92.5108959842799,
73.456193310475));
#212736=CARTESIAN_POINT('Ctrl Pts',(-64.1503872955297,-93.4520697801033,
70.6948366673944));
#212737=CARTESIAN_POINT('Ctrl Pts',(-64.0255170966268,-92.9978260136282,
66.3417152089329));
#212738=CARTESIAN_POINT('Ctrl Pts',(-63.900646897724,-90.7607339677282,
62.5800564935892));
#212739=CARTESIAN_POINT('Ctrl Pts',(-63.7757766988212,-87.1529364041481,
60.1024278538446));
#212740=CARTESIAN_POINT('Ctrl Pts',(-63.6509064999184,-82.838849969827,
59.3651968840528));
#212741=CARTESIAN_POINT('Ctrl Pts',(-63.5260363010159,-78.6130151857575,
60.5041244100999));
#212742=CARTESIAN_POINT('Ctrl Pts',(-63.4011661021129,-75.2537068952662,
63.309456950552));
#212743=CARTESIAN_POINT('Ctrl Pts',(-63.2762959032099,-73.3796139286711,
67.2645316790695));
#212744=CARTESIAN_POINT('Ctrl Pts',(-63.1514257043069,-73.3358902062209,
71.6409376007934));
#212745=CARTESIAN_POINT('Ctrl Pts',(-63.0265555054049,-75.1305884650834,
75.6326666763601));
#212746=CARTESIAN_POINT('Ctrl Pts',(-62.9016853065019,-78.4331766789858,
78.5045557099474));
#212747=CARTESIAN_POINT('Ctrl Pts',(-62.7768151075989,-82.6354133877224,
79.7276901708313));
#212748=CARTESIAN_POINT('Ctrl Pts',(-62.6519449086969,-86.9633655252361,
79.0767852379245));
#212749=CARTESIAN_POINT('Ctrl Pts',(-62.5270747097939,-90.6199549881801,
76.6717882291845));
#212750=CARTESIAN_POINT('Ctrl Pts',(-62.4022045108909,-92.9317190450487,
72.9553718401246));
#212751=CARTESIAN_POINT('Ctrl Pts',(-62.3189577116229,-93.2925640031029,
70.0604297784402));
#212752=CARTESIAN_POINT('Ctrl Pts',(-62.2773343119879,-93.1612338157616,
68.6413167259844));
#212753=CARTESIAN_POINT('Ctrl Pts',(-64.0511293841564,-92.1405515484729,
74.8981865183927));
#212754=CARTESIAN_POINT('Ctrl Pts',(-64.0095059845222,-92.911285154521,
73.6262270025224));
#212755=CARTESIAN_POINT('Ctrl Pts',(-63.9262591852536,-93.8934511110742,
70.7446014188501));
#212756=CARTESIAN_POINT('Ctrl Pts',(-63.8013889863508,-93.4194230778007,
66.2018828261753));
#212757=CARTESIAN_POINT('Ctrl Pts',(-63.676518787448,-91.0848960660067,
62.2763877191447));
#212758=CARTESIAN_POINT('Ctrl Pts',(-63.5516485885449,-87.319963424663,
59.6908477118418));
#212759=CARTESIAN_POINT('Ctrl Pts',(-63.4267783896419,-82.817979999059,
58.9215071672393));
#212760=CARTESIAN_POINT('Ctrl Pts',(-63.3019081907399,-78.4080919620894,
60.1100398782211));
#212761=CARTESIAN_POINT('Ctrl Pts',(-63.1770379918369,-74.9024713688351,
63.0375566984567));
#212762=CARTESIAN_POINT('Ctrl Pts',(-63.0521677929339,-72.9467536051585,
67.1648919166654));
#212763=CARTESIAN_POINT('Ctrl Pts',(-62.9272975940309,-72.9011255268212,
71.7319091109724));
#212764=CARTESIAN_POINT('Ctrl Pts',(-62.8024273951289,-74.7739906022782,
75.8974951304588));
#212765=CARTESIAN_POINT('Ctrl Pts',(-62.6775571962259,-78.2204207160243,
78.8944672649293));
#212766=CARTESIAN_POINT('Ctrl Pts',(-62.5526869973229,-82.6056828801404,
80.1708744843959));
#212767=CARTESIAN_POINT('Ctrl Pts',(-62.4278167984199,-87.1221359198457,
79.4916198463129));
#212768=CARTESIAN_POINT('Ctrl Pts',(-62.3029465995179,-90.9379855573115,
76.9818748894682));
#212769=CARTESIAN_POINT('Ctrl Pts',(-62.1780764006149,-93.3504368668442,
73.1035926063291));
#212770=CARTESIAN_POINT('Ctrl Pts',(-62.0948296013469,-93.7269981724799,
70.0825633853881));
#212771=CARTESIAN_POINT('Ctrl Pts',(-62.0532062017119,-93.589947991478,
68.601641865046));
#212772=CARTESIAN_POINT('Origin',(-113.778845940191,-83.3180213346267,69.5522455184007));
#212773=CARTESIAN_POINT('',(-47.1840596451118,-88.6014372352785,74.6727879441187));
#212774=CARTESIAN_POINT('Ctrl Pts',(-47.1840596451125,-88.6014372352776,
74.6727879441184));
#212775=CARTESIAN_POINT('Ctrl Pts',(-47.1330608433754,-88.9445087024433,
73.6555434581613));
#212776=CARTESIAN_POINT('Ctrl Pts',(-47.0897582262311,-89.1384560838077,
72.5407972914318));
#212777=CARTESIAN_POINT('Ctrl Pts',(-47.0209270037,-89.1523705823679,70.0468757692862));
#212778=CARTESIAN_POINT('Ctrl Pts',(-47.002286125824,-88.8674259744689,
68.6660964641815));
#212779=CARTESIAN_POINT('Ctrl Pts',(-47.002286125824,-87.8745905336971,
66.2630466589398));
#212780=CARTESIAN_POINT('Ctrl Pts',(-47.0209270037,-87.1018460587871,65.0838049977557));
#212781=CARTESIAN_POINT('Ctrl Pts',(-47.0897582262311,-85.3317069868201,
63.3269766516198));
#212782=CARTESIAN_POINT('Ctrl Pts',(-47.1330608433754,-84.4074978736294,
62.6742040127388));
#212783=CARTESIAN_POINT('Ctrl Pts',(-47.1840596451125,-83.4464714330091,
62.1957559421795));
#212784=CARTESIAN_POINT('Origin',(-113.778845940191,-85.8955042357612,75.7907615193707));
#212785=CARTESIAN_POINT('Origin',(-113.778845940191,-83.3180213346267,69.5522455184007));
#212786=CARTESIAN_POINT('Origin',(-51.8559251551109,-81.1469531033262,77.7526558780789));
#212787=CARTESIAN_POINT('',(-47.1840596451109,-88.6014372352783,74.6727879441188));
#212788=CARTESIAN_POINT('Origin',(-51.5615184913109,-79.584953311077,71.0945865171214));
#221645=UNCERTAINTY_MEASURE_WITH_UNIT(LENGTH_MEASURE(0.01),#221663,
'DISTANCE_ACCURACY_VALUE',
'Maximum model space distance between geometric entities at asserted c
onnectivities');
#221647=UNCERTAINTY_MEASURE_WITH_UNIT(LENGTH_MEASURE(0.01),#221663,
'DISTANCE_ACCURACY_VALUE',
'Maximum model space distance between geometric entities at asserted c
onnectivities');
#221660=(
GEOMETRIC_REPRESENTATION_CONTEXT(3)
GLOBAL_UNCERTAINTY_ASSIGNED_CONTEXT((#221645))
GLOBAL_UNIT_ASSIGNED_CONTEXT((#221663,#221665,#221666))
REPRESENTATION_CONTEXT('','3D')
);
#221662=(
GEOMETRIC_REPRESENTATION_CONTEXT(3)
GLOBAL_UNCERTAINTY_ASSIGNED_CONTEXT((#221647))
GLOBAL_UNIT_ASSIGNED_CONTEXT((#221663,#221665,#221666))
REPRESENTATION_CONTEXT('','3D')
);
#221663=(
LENGTH_UNIT()
NAMED_UNIT(*)
SI_UNIT(.MILLI.,.METRE.)
);
#221665=(
NAMED_UNIT(*)
PLANE_ANGLE_UNIT()
SI_UNIT($,.RADIAN.)
);
#221666=(
NAMED_UNIT(*)
SI_UNIT($,.STERADIAN.)
SOLID_ANGLE_UNIT()
);
#221679=SHAPE_DEFINITION_REPRESENTATION(#221693,#221720);
#221693=PRODUCT_DEFINITION_SHAPE('',$,#221735);
#221720=SHAPE_REPRESENTATION('',(#85967),#221660);
#221722=PRODUCT_DEFINITION_CONTEXT('part definition',#221766,'design');
#221735=PRODUCT_DEFINITION('2026-10-05-23-02-49-354',
'Eccentric Connector (1)',#221749,#221722);
#221749=PRODUCT_DEFINITION_FORMATION('',$,#221780);
#221766=APPLICATION_CONTEXT(
'Core Data for Automotive Mechanical Design Process');
#221767=PRODUCT_CONTEXT('part definition',#221766,'mechanical');
#221780=PRODUCT('2026-10-05-23-02-49-354','Eccentric Connector (1)',$,(#221767));
#221783=PRESENTATION_STYLE_ASSIGNMENT((#221785));
#221785=SURFACE_STYLE_USAGE(.BOTH.,#221787);
#221787=SURFACE_SIDE_STYLE('',(#221789));
#221789=SURFACE_STYLE_FILL_AREA(#221791);
#221791=FILL_AREA_STYLE('Opaque(202,209,238)',(#221793));
#221793=FILL_AREA_STYLE_COLOUR('Opaque(202,209,238)',#221795);
#221795=COLOUR_RGB('Opaque(202,209,238)', 0.09019608, 0.27058824, 0.51372549);
ENDSEC;
END-ISO-10303-21;
